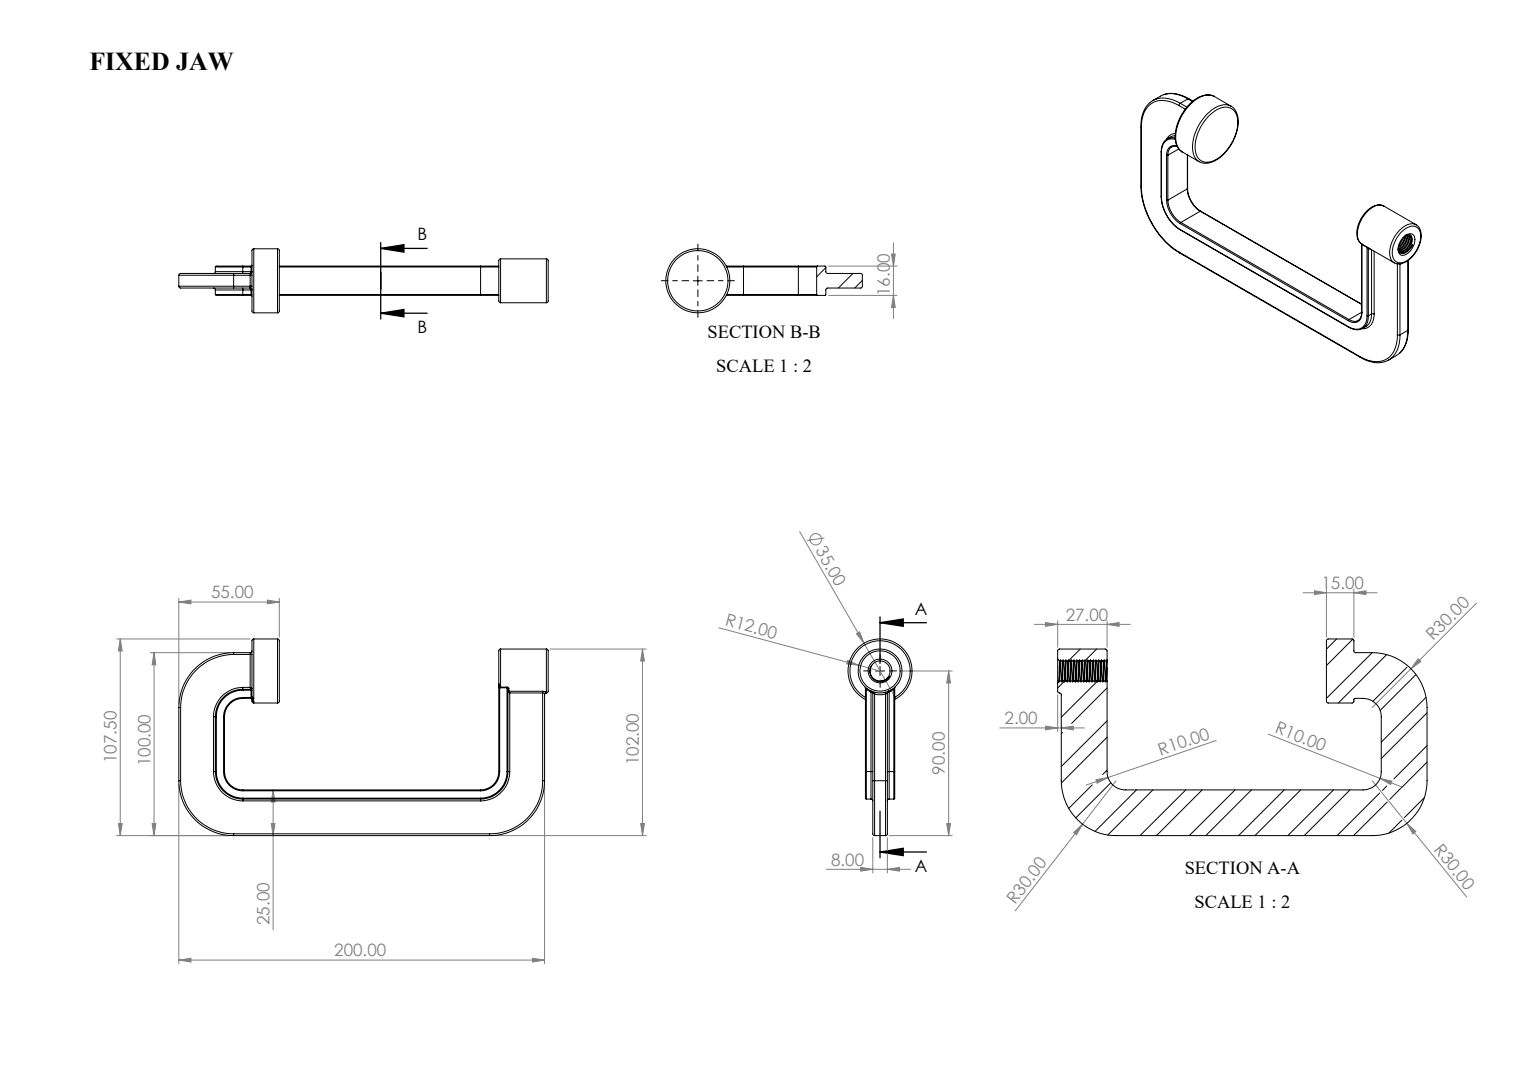
ISO-10303-21;
HEADER;
FILE_DESCRIPTION (('STEP AP214'),
    '1' );
FILE_NAME ('Fixed Jaw.step',
    '2026-10-07T06:38:26',
    ( '' ),
    ( '' ),
    'SwSTEP 2.0',
    'SolidWorks 2021',
    '' );
FILE_SCHEMA (( 'AUTOMOTIVE_DESIGN' ));
ENDSEC;

DATA;
#2=ORIENTED_EDGE ( 'NONE', *, *, #13115, .T. ) ;
#3=CARTESIAN_POINT ( 'NONE',  ( 151.8675748654052029, -5.500000000000012434, 2.278174593052012309 ) ) ;
#4=CARTESIAN_POINT ( 'NONE',  ( 134.2500000000000284, -6.000000000000005329, 0.000000000000000000 ) ) ;
#7=( NAMED_UNIT ( * ) PLANE_ANGLE_UNIT ( ) SI_UNIT ( $, .RADIAN. ) );
#9=ADVANCED_FACE ( 'NONE', ( #19589 ), #12972, .F. ) ;
#11=VECTOR ( 'NONE', #10192, 1000.000000000000000 ) ;
#14=CARTESIAN_POINT ( 'NONE',  ( 116.0000000000000142, 6.735557395310442023E-16, 5.500000000000000000 ) ) ;
#17=CARTESIAN_POINT ( 'NONE',  ( 143.2351497308104058, 3.535533905932725318, -3.535533905932725318 ) ) ;
#19=DIRECTION ( 'NONE',  ( -0.000000000000000000, -0.000000000000000000, -1.000000000000000000 ) ) ;
#25=DIRECTION ( 'NONE',  ( 0.000000000000000000, 0.000000000000000000, -1.000000000000000000 ) ) ;
#28=DIRECTION ( 'NONE',  ( 1.000000000000000000, 0.000000000000000000, 0.000000000000000000 ) ) ;
#31=ORIENTED_EDGE ( 'NONE', *, *, #1535, .F. ) ;
#33=CARTESIAN_POINT ( 'NONE',  ( 142.6875000000000284, 4.242640687119269671, 4.242640687119298093 ) ) ;
#38=CARTESIAN_POINT ( 'NONE',  ( 160.5788997308103774, -4.999999999999989342, 2.071067811865468400 ) ) ;
#42=VERTEX_POINT ( 'NONE', #1381 ) ;
#44=ORIENTED_EDGE ( 'NONE', *, *, #20112, .T. ) ;
#49=CARTESIAN_POINT ( 'NONE',  ( 159.6411875853270885, -12.17723633016814233, -3.777793391642500165 ) ) ;
#53=DIRECTION ( 'NONE',  ( -1.000000000000000000, -0.000000000000000000, -0.000000000000000000 ) ) ;
#54=VECTOR ( 'NONE', #17424, 1000.000000000000000 ) ;
#56=ADVANCED_FACE ( 'NONE', ( #10625 ), #5822, .T. ) ;
#60=CARTESIAN_POINT ( 'NONE',  ( 139.5760635317500089, -9.165151396444613852, -8.000000000000007105 ) ) ;
#64=DIRECTION ( 'NONE',  ( 6.938893903907222067E-15, 1.000000000000000000, 0.000000000000000000 ) ) ;
#69=CARTESIAN_POINT ( 'NONE',  ( 145.1398502691896510, -3.535533905932752852, 3.535533905932725318 ) ) ;
#72=CARTESIAN_POINT ( 'NONE',  ( 157.4062500000000284, 6.000000000000005329, -2.485281374238556218 ) ) ;
#77=DIRECTION ( 'NONE',  ( 1.000000000000000000, 0.000000000000000000, 0.000000000000000000 ) ) ;
#79=CARTESIAN_POINT ( 'NONE',  ( 150.3750000000000284, 0.000000000000000000, 6.000000000000005329 ) ) ;
#83=ORIENTED_EDGE ( 'NONE', *, *, #26629, .F. ) ;
#88=EDGE_CURVE ( 'NONE', #16343, #27983, #2946, .T. ) ;
#93=CARTESIAN_POINT ( 'NONE',  ( 156.4538997308104626, -2.071067811865468400, -4.999999999999989342 ) ) ;
#96=CARTESIAN_POINT ( 'NONE',  ( 135.6737246954180023, -8.728829995094853800, 8.172675940893835644 ) ) ;
#98=ADVANCED_FACE ( 'NONE', ( #17543 ), #26707, .F. ) ;
#101=STYLED_ITEM ( 'NONE', ( #7132 ), #3790 ) ;
#107=CARTESIAN_POINT ( 'NONE',  ( 135.0000000000000284, -54.99999999999993605, -7.500000000000007105 ) ) ;
#108=CARTESIAN_POINT ( 'NONE',  ( 125.0000000000000568, -55.00000000000000711, -7.500000000000007105 ) ) ;
#111=CARTESIAN_POINT ( 'NONE',  ( 161.5461002691896226, -2.071067811865468400, 4.999999999999989342 ) ) ;
#112=CARTESIAN_POINT ( 'NONE',  ( 0.7724517649218355375, -15.49026069396310490, 8.142614232235679594 ) ) ;
#117=CARTESIAN_POINT ( 'NONE',  ( -4.999999999999990230, -55.00000000000002132, 5.000000000000004441 ) ) ;
#121=DIRECTION ( 'NONE',  ( 0.000000000000000000, 0.000000000000000000, -1.000000000000000000 ) ) ;
#125=CARTESIAN_POINT ( 'NONE',  ( 151.9687500000000568, -2.485281374238585972, 6.000000000000005329 ) ) ;
#126=ORIENTED_EDGE ( 'NONE', *, *, #11372, .T. ) ;
#136=CARTESIAN_POINT ( 'NONE',  ( 134.2351497308104058, 3.535533905932725318, -3.535533905932725318 ) ) ;
#138=CARTESIAN_POINT ( 'NONE',  ( 0.1879814459054835185, -15.40071801525260220, -8.313003687118166951 ) ) ;
#139=ADVANCED_FACE ( 'NONE', ( #915 ), #19679, .F. ) ;
#140=COLOUR_RGB ( '', 0.31764706, 0.68627451, 0.89019608) ;
#142=CYLINDRICAL_SURFACE ( 'NONE', #25085, 0.5000000000000004441 ) ;
#146=CARTESIAN_POINT ( 'NONE',  ( -0.5130136762305975706, -9.973972647538804637, -4.738252045315842764 ) ) ;
#147=CARTESIAN_POINT ( 'NONE',  ( 159.9897649647779474, -11.17313463120727057, -4.377898023955410167 ) ) ;
#150=CARTESIAN_POINT ( 'NONE',  ( 135.0000000000000284, -8.662311887307041047, -7.546725650337192448 ) ) ;
#151=CARTESIAN_POINT ( 'NONE',  ( 154.1175748654052313, 5.500000000000012434, -2.278174593052012309 ) ) ;
#158=AXIS2_PLACEMENT_3D ( 'NONE', #25640, #4289, #30093 ) ;
#162=CARTESIAN_POINT ( 'NONE',  ( 142.5863248654052313, 0.000000000000000000, 5.500000000000005329 ) ) ;
#164=ORIENTED_EDGE ( 'NONE', *, *, #27531, .F. ) ;
#167=CARTESIAN_POINT ( 'NONE',  ( 135.1875000000000568, 4.242640687119269671, 4.242640687119298093 ) ) ;
#168=EDGE_CURVE ( 'NONE', #2390, #1119, #5990, .T. ) ;
#169=ADVANCED_FACE ( 'NONE', ( #22749 ), #29791, .T. ) ;
#171=CARTESIAN_POINT ( 'NONE',  ( -4.999999999999920952, -65.50000000000001421, -8.000000000000007105 ) ) ;
#172=( NAMED_UNIT ( * ) PLANE_ANGLE_UNIT ( ) SI_UNIT ( $, .RADIAN. ) );
#175=CIRCLE ( 'NONE', #14898, 0.5000000000000004441 ) ;
#176=CARTESIAN_POINT ( 'NONE',  ( 144.5476497308104058, 0.000000000000000000, -5.000000000000004441 ) ) ;
#180=AXIS2_PLACEMENT_3D ( 'NONE', #24945, #8684, #29090 ) ;
#183=ORIENTED_EDGE ( 'NONE', *, *, #15487, .T. ) ;
#185=DIRECTION ( 'NONE',  ( 0.000000000000000000, 0.000000000000000000, 1.000000000000000000 ) ) ;
#187=ORIENTED_EDGE ( 'NONE', *, *, #6959, .T. ) ;
#189=CARTESIAN_POINT ( 'NONE',  ( 139.2187500000000284, 2.485281374238556218, -6.000000000000005329 ) ) ;
#191=DIRECTION ( 'NONE',  ( -0.000000000000000000, 1.000000000000000000, -0.000000000000000000 ) ) ;
#192=CARTESIAN_POINT ( 'NONE',  ( 132.8437500000000284, -6.000000000000005329, -2.485281374238555774 ) ) ;
#193=COLOUR_RGB ( '', 0.31764706, 0.68627451, 0.89019608) ;
#195=EDGE_CURVE ( 'NONE', #1664, #6421, #4446, .T. ) ;
#200=CARTESIAN_POINT ( 'NONE',  ( -19.99999999999998224, -25.00000000000010658, -5.000000000000004441 ) ) ;
#217=CARTESIAN_POINT ( 'NONE',  ( 145.0461002691896510, -2.071067811865468400, 4.999999999999989342 ) ) ;
#219=CARTESIAN_POINT ( 'NONE',  ( 157.2187500000000284, 2.485281374238556218, -6.000000000000005329 ) ) ;
#227=CARTESIAN_POINT ( 'NONE',  ( 149.4375000000000284, -4.242640687119298093, -4.242640687119298093 ) ) ;
#234=VERTEX_POINT ( 'NONE', #29941 ) ;
#239=CARTESIAN_POINT ( 'NONE',  ( 154.6726497308104058, -5.000000000000004441, 0.000000000000000000 ) ) ;
#242=DIRECTION ( 'NONE',  ( 1.000000000000000000, -0.000000000000000000, -0.000000000000000000 ) ) ;
#245=LINE ( 'NONE', #5439, #2253 ) ;
#246=AXIS2_PLACEMENT_3D ( 'NONE', #9140, #8524, #18081 ) ;
#250=AXIS2_PLACEMENT_3D ( 'NONE', #6454, #4145, #24741 ) ;
#252=DIRECTION ( 'NONE',  ( 1.000000000000000000, 0.000000000000000000, 0.000000000000000000 ) ) ;
#253=CARTESIAN_POINT ( 'NONE',  ( 144.7574251345947687, -2.278174593051733421, 5.500000000000292211 ) ) ;
#257=CARTESIAN_POINT ( 'NONE',  ( 156.7648502691896510, 3.535533905932725318, 3.535533905932752852 ) ) ;
#258=CARTESIAN_POINT ( 'NONE',  ( 124.9999999999999432, -65.00000000000000000, -7.500000000000007105 ) ) ;
#259=ORIENTED_EDGE ( 'NONE', *, *, #5614, .F. ) ;
#273=CARTESIAN_POINT ( 'NONE',  ( 153.4687500000000853, -2.485281374238585972, 6.000000000000005329 ) ) ;
#278=VERTEX_POINT ( 'NONE', #29639 ) ;
#279=CARTESIAN_POINT ( 'NONE',  ( 116.0000000000000142, 0.000000000000000000, 0.000000000000000000 ) ) ;
#289=SURFACE_SIDE_STYLE ('',( #7647 ) ) ;
#294=ORIENTED_EDGE ( 'NONE', *, *, #12008, .F. ) ;
#296=CIRCLE ( 'NONE', #5196, 0.5000000000000004441 ) ;
#299=LINE ( 'NONE', #12465, #20459 ) ;
#302=PLANE ( 'NONE',  #5431 ) ;
#307=CARTESIAN_POINT ( 'NONE',  ( 157.0386751345948539, -5.500000000000005329, 0.000000000000000000 ) ) ;
#308=CARTESIAN_POINT ( 'NONE',  ( 140.9925748654052029, 2.278174593052074925, 5.499999999999950262 ) ) ;
#311=CARTESIAN_POINT ( 'NONE',  ( 138.4687500000000284, -2.485281374238585972, 6.000000000000005329 ) ) ;
#314=( LENGTH_UNIT ( ) NAMED_UNIT ( * ) SI_UNIT ( .MILLI., .METRE. ) );
#318=CARTESIAN_POINT ( 'NONE',  ( 0.1092184406287978471, -15.15152031211519201, 8.760553818335999665 ) ) ;
#319=CARTESIAN_POINT ( 'NONE',  ( 136.1101497308104342, 3.535533905932725318, 3.535533905932725318 ) ) ;
#327=ORIENTED_EDGE ( 'NONE', *, *, #30362, .T. ) ;
#328=ADVANCED_FACE ( 'NONE', ( #15715 ), #11243, .F. ) ;
#329=CARTESIAN_POINT ( 'NONE',  ( -20.99999999999998224, -54.99999999999990763, -4.000000000000003553 ) ) ;
#332=EDGE_CURVE ( 'NONE', #7475, #16343, #25564, .T. ) ;
#333=ORIENTED_EDGE ( 'NONE', *, *, #11296, .T. ) ;
#337=CARTESIAN_POINT ( 'NONE',  ( 133.5000000000000284, 6.000000000000005329, 0.000000000000000000 ) ) ;
#339=COLOUR_RGB ( '', 0.72549020, 0.75294118, 0.79215686) ;
#346=CARTESIAN_POINT ( 'NONE',  ( 159.0000000000000284, -12.00000000000001066, -4.000000000000003553 ) ) ;
#348=AXIS2_PLACEMENT_3D ( 'NONE', #13196, #18093, #13038 ) ;
#350=CARTESIAN_POINT ( 'NONE',  ( 140.9019117484300523, -11.80382349685862486, -4.000000000000003553 ) ) ;
#351=DIRECTION ( 'NONE',  ( 1.000000000000000000, -0.000000000000000000, -0.000000000000000000 ) ) ;
#354=CARTESIAN_POINT ( 'NONE',  ( 140.0509928599997238, -9.340762233865111952, 7.535282035301673176 ) ) ;
#355=AXIS2_PLACEMENT_3D ( 'NONE', #19839, #19142, #17411 ) ;
#358=AXIS2_PLACEMENT_3D ( 'NONE', #28689, #759, #17069 ) ;
#359=CARTESIAN_POINT ( 'NONE',  ( 145.1175748654052597, 5.500000000000012434, -2.278174593052012309 ) ) ;
#362=EDGE_CURVE ( 'NONE', #22602, #4075, #22644, .T. ) ;
#363=CARTESIAN_POINT ( 'NONE',  ( 139.5500633684294769, -9.165151389911672553, 8.000000000000010658 ) ) ;
#364=CARTESIAN_POINT ( 'NONE',  ( 146.8273502691896510, -5.000000000000004441, 0.000000000000000000 ) ) ;
#365=CARTESIAN_POINT ( 'NONE',  ( 13.99999999999999822, 0.000000000000000000, 17.50000000000000355 ) ) ;
#366=CARTESIAN_POINT ( 'NONE',  ( 160.5937500000000284, 6.000000000000005329, 2.485281374238585972 ) ) ;
#367=CARTESIAN_POINT ( 'NONE',  ( 135.0000000000000284, -8.301023251189437957, -7.690744244795082452 ) ) ;
#368=FACE_OUTER_BOUND ( 'NONE', #26036, .T. ) ;
#370=( NAMED_UNIT ( * ) PLANE_ANGLE_UNIT ( ) SI_UNIT ( $, .RADIAN. ) );
#372=CARTESIAN_POINT ( 'NONE',  ( 148.4062500000000568, 6.000000000000005329, -2.485281374238555774 ) ) ;
#374=( NAMED_UNIT ( * ) PLANE_ANGLE_UNIT ( ) SI_UNIT ( $, .RADIAN. ) );
#379=VERTEX_POINT ( 'NONE', #23659 ) ;
#383=CARTESIAN_POINT ( 'NONE',  ( 155.5163997308104342, 4.999999999999989342, 2.071067811865468400 ) ) ;
#387=SURFACE_SIDE_STYLE ('',( #14990 ) ) ;
#397=PLANE ( 'NONE',  #15284 ) ;
#400=CARTESIAN_POINT ( 'NONE',  ( 155.3586002691896226, 2.071067811865468400, 4.999999999999989342 ) ) ;
#404=CARTESIAN_POINT ( 'NONE',  ( 149.3363248654052029, 0.000000000000000000, -5.500000000000005329 ) ) ;
#410=ORIENTED_EDGE ( 'NONE', *, *, #8956, .T. ) ;
#412=ORIENTED_EDGE ( 'NONE', *, *, #17980, .F. ) ;
#413=CARTESIAN_POINT ( 'NONE',  ( 146.7187500000000284, 2.485281374238555774, -6.000000000000005329 ) ) ;
#414=ORIENTED_EDGE ( 'NONE', *, *, #12706, .T. ) ;
#418=UNCERTAINTY_MEASURE_WITH_UNIT (LENGTH_MEASURE( 1.000000000000000082E-05 ), #11834, 'distance_accuracy_value', 'NONE');
#423=CARTESIAN_POINT ( 'NONE',  ( 133.4851497308104058, -3.535533905932725318, 3.535533905932725318 ) ) ;
#426=CARTESIAN_POINT ( 'NONE',  ( 0.2111655239558809238, -15.49101385207805492, -8.141616853885579985 ) ) ;
#427=CARTESIAN_POINT ( 'NONE',  ( 158.5386751345948539, -5.500000000000005329, 0.000000000000000000 ) ) ;
#428=CYLINDRICAL_SURFACE ( 'NONE', #8935, 30.00000000000000000 ) ;
#436=EDGE_CURVE ( 'NONE', #17742, #25655, #11378, .T. ) ;
#438=CARTESIAN_POINT ( 'NONE',  ( 135.4999999999990052, -9.047800747817513312, -8.000000000000007105 ) ) ;
#441=DIRECTION ( 'NONE',  ( 0.000000000000000000, 0.000000000000000000, -1.000000000000000000 ) ) ;
#446=AXIS2_PLACEMENT_3D ( 'NONE', #10967, #13586, #23085 ) ;
#450=( BOUNDED_CURVE ( )  B_SPLINE_CURVE ( 2, ( #19930, #8557, #7941, #22090, #29276, #19775, #5935, #15359, #8402 ),
 .UNSPECIFIED., .F., .F. ) 
 B_SPLINE_CURVE_WITH_KNOTS ( ( 3, 2, 2, 2, 3 ),
 ( 0.1874999999999996947, 0.1937499999999999500, 0.2000000000000002054, 0.2062500000000004330, 0.2125000000000006883 ),
 .UNSPECIFIED. ) 
 CURVE ( )  GEOMETRIC_REPRESENTATION_ITEM ( )  RATIONAL_B_SPLINE_CURVE ( ( 1.000000000000003775, 0.9238795325112830747, 1.000000000000000000, 0.9238795325112867385, 1.000000000000000000, 0.9238795325112867385, 1.000000000000000000, 0.9238795325112783008, 1.000000000000008438 ) ) 
 REPRESENTATION_ITEM ( '' )  );
#452=VERTEX_POINT ( 'NONE', #16766 ) ;
#454=CARTESIAN_POINT ( 'NONE',  ( 134.4523502691896510, 0.000000000000000000, 5.000000000000004441 ) ) ;
#459=CARTESIAN_POINT ( 'NONE',  ( 116.0000000000000142, 0.000000000000000000, -5.500000000000000000 ) ) ;
#461=ORIENTED_EDGE ( 'NONE', *, *, #4777, .F. ) ;
#463=CARTESIAN_POINT ( 'NONE',  ( 0.1053031288717025393, -15.23283975038566318, 8.619984219653339608 ) ) ;
#464=CARTESIAN_POINT ( 'NONE',  ( 139.8601497308104058, -3.535533905932725318, -3.535533905932725318 ) ) ;
#466=DIRECTION ( 'NONE',  ( 1.000000000000000000, 0.000000000000000000, 0.000000000000000000 ) ) ;
#468=( NAMED_UNIT ( * ) PLANE_ANGLE_UNIT ( ) SI_UNIT ( $, .RADIAN. ) );
#476=VERTEX_POINT ( 'NONE', #745 ) ;
#477=DIRECTION ( 'NONE',  ( 0.000000000000000000, 1.224646799147353454E-16, 1.000000000000000000 ) ) ;
#479=ORIENTED_EDGE ( 'NONE', *, *, #25996, .F. ) ;
#481=CARTESIAN_POINT ( 'NONE',  ( 136.2187500000000284, 2.485281374238556218, -6.000000000000005329 ) ) ;
#485=CARTESIAN_POINT ( 'NONE',  ( 160.9538997308104058, -2.071067811865468400, -4.999999999999989342 ) ) ;
#487=CIRCLE ( 'NONE', #25995, 17.50000000000000355 ) ;
#489=AXIS2_PLACEMENT_3D ( 'NONE', #15313, #15469, #1284 ) ;
#493=EDGE_CURVE ( 'NONE', #3216, #20658, #28980, .T. ) ;
#502=CARTESIAN_POINT ( 'NONE',  ( 116.0000000000000142, 0.000000000000000000, -5.500000000000000000 ) ) ;
#507=CARTESIAN_POINT ( 'NONE',  ( 139.6011751345948539, 3.889087296526011706, -3.889087296526011706 ) ) ;
#508=AXIS2_PLACEMENT_3D ( 'NONE', #25825, #23387, #22922 ) ;
#513=CARTESIAN_POINT ( 'NONE',  ( 146.5461002691896510, -2.071067811865468400, 4.999999999999989342 ) ) ;
#515=CARTESIAN_POINT ( 'NONE',  ( 153.9375000000000284, -4.242640687119298093, -4.242640687119298093 ) ) ;
#519=AXIS2_PLACEMENT_3D ( 'NONE', #17217, #21810, #19211 ) ;
#520=ORIENTED_EDGE ( 'NONE', *, *, #8340, .T. ) ;
#521=CARTESIAN_POINT ( 'NONE',  ( 149.6250000000000284, 0.000000000000000000, -6.000000000000005329 ) ) ;
#523=UNCERTAINTY_MEASURE_WITH_UNIT (LENGTH_MEASURE( 1.000000000000000082E-05 ), #26176, 'distance_accuracy_value', 'NONE');
#527=ORIENTED_EDGE ( 'NONE', *, *, #25589, .T. ) ;
#535=ORIENTED_EDGE ( 'NONE', *, *, #24962, .F. ) ;
#540=CARTESIAN_POINT ( 'NONE',  ( 134.9486760520005078, -8.594915014419392207, 8.000000000000007105 ) ) ;
#543=CARTESIAN_POINT ( 'NONE',  ( 143.3363248654052029, 0.000000000000000000, -5.500000000000005329 ) ) ;
#547=( BOUNDED_SURFACE ( )  B_SPLINE_SURFACE ( 3, 2, ( 
 ( #13704, #1829, #23045 ),
 ( #11233, #20739, #27768 ),
 ( #8443, #14456, #16759 ),
 ( #2587, #11702, #20890 ),
 ( #2301, #21499, #23504 ),
 ( #4588, #426, #4740 ),
 ( #16902, #19192, #4435 ),
 ( #7051, #14167, #11858 ),
 ( #21198, #138, #737 ),
 ( #26662, #8079, #7637 ),
 ( #12747, #12446, #19491 ),
 ( #10269, #10420, #14736 ),
 ( #17198, #19634, #26225 ),
 ( #24223, #10119, #7781 ) ),
 .UNSPECIFIED., .F., .F., .F. ) 
 B_SPLINE_SURFACE_WITH_KNOTS ( ( 4, 2, 2, 2, 2, 2, 4 ),
 ( 3, 3 ),
 ( 0.007087992156775593799, 0.007143427954787825995, 0.007198863752800057324, 0.007254299550812288652, 0.007309735348824520848, 0.007420606944848983505, 0.007531478540873447029 ),
 ( 0.000000000000000000, 1.000000000000000000 ),
 .UNSPECIFIED. ) 
 GEOMETRIC_REPRESENTATION_ITEM ( )  RATIONAL_B_SPLINE_SURFACE ( (
 ( 1.000000000000000000, 0.8593225670956824436, 1.000000000000000000),
 ( 1.000000000000000000, 0.8663660590095438874, 1.000000000000000000),
 ( 1.000000000000000000, 0.8726340236266260098, 1.000000000000000000),
 ( 1.000000000000000000, 0.8802009473587890653, 1.000000000000000000),
 ( 1.000000000000000000, 0.8813323811479394365, 1.000000000000000000),
 ( 1.000000000000000000, 0.8771298408144754255, 1.000000000000000000),
 ( 1.000000000000000000, 0.8720285761146205905, 1.000000000000000000),
 ( 1.000000000000000000, 0.8593306477498514617, 1.000000000000000000),
 ( 1.000000000000000000, 0.8518162931196250343, 1.000000000000000000),
 ( 1.000000000000000000, 0.8295128813679467639, 1.000000000000000000),
 ( 1.000000000000000000, 0.8153081809651850920, 1.000000000000000000),
 ( 1.000000000000000000, 0.7919334258735726273, 1.000000000000000000),
 ( 1.000000000000000000, 0.7823637235328708694, 1.000000000000000000),
 ( 1.000000000000000000, 0.7743236465966842896, 1.000000000000000000) ) ) 
 REPRESENTATION_ITEM ( '' )  SURFACE ( )  );
#550=CARTESIAN_POINT ( 'NONE',  ( 145.4136751345948539, 0.000000000000000000, -5.500000000000005329 ) ) ;
#552=CARTESIAN_POINT ( 'NONE',  ( 135.5550748654052313, -5.500000000000012434, -2.278174593052012309 ) ) ;
#556=DIRECTION ( 'NONE',  ( 0.000000000000000000, 0.000000000000000000, -1.000000000000000000 ) ) ;
#557=AXIS2_PLACEMENT_3D ( 'NONE', #30242, #4590, #11704 ) ;
#558=( NAMED_UNIT ( * ) PLANE_ANGLE_UNIT ( ) SI_UNIT ( $, .RADIAN. ) );
#560=ORIENTED_EDGE ( 'NONE', *, *, #8732, .F. ) ;
#573=CARTESIAN_POINT ( 'NONE',  ( 158.3363248654052313, 0.000000000000000000, -5.500000000000005329 ) ) ;
#577=CARTESIAN_POINT ( 'NONE',  ( 132.7351497308104058, 3.535533905932725318, -3.535533905932725318 ) ) ;
#582=CARTESIAN_POINT ( 'NONE',  ( 158.7261751345948539, -3.889087296526011706, -3.889087296526011706 ) ) ;
#587=DIRECTION ( 'NONE',  ( 0.000000000000000000, 1.000000000000000000, -1.224646799147353207E-16 ) ) ;
#588=DIRECTION ( 'NONE',  ( 1.000000000000000000, 0.000000000000000000, 0.000000000000000000 ) ) ;
#591=( BOUNDED_CURVE ( )  B_SPLINE_CURVE ( 3, ( #1681, #22434, #25161, #22888 ),
 .UNSPECIFIED., .F., .T. ) 
 B_SPLINE_CURVE_WITH_KNOTS ( ( 4, 4 ),
 ( 1.570796326794896558, 2.746801533890014468 ),
 .UNSPECIFIED. ) 
 CURVE ( )  GEOMETRIC_REPRESENTATION_ITEM ( )  RATIONAL_B_SPLINE_CURVE ( ( 1.000000000000000000, 0.8880335295585656263, 0.8880335295585656263, 1.000000000000000000 ) ) 
 REPRESENTATION_ITEM ( '' )  );
#593=DIRECTION ( 'NONE',  ( -1.000000000000000000, 6.938893903907221278E-15, 0.000000000000000000 ) ) ;
#598=PLANE ( 'NONE',  #4757 ) ;
#600=ORIENTED_EDGE ( 'NONE', *, *, #19995, .T. ) ;
#601=EDGE_CURVE ( 'NONE', #5531, #29422, #23638, .T. ) ;
#605=VERTEX_POINT ( 'NONE', #14955 ) ;
#608=FACE_OUTER_BOUND ( 'NONE', #22324, .T. ) ;
#609=CARTESIAN_POINT ( 'NONE',  ( 161.5312500000000568, -2.485281374238555774, -6.000000000000005329 ) ) ;
#610=EDGE_CURVE ( 'NONE', #5920, #21964, #16795, .T. ) ;
#612=EDGE_LOOP ( 'NONE', ( #28143, #13844, #4187, #4536 ) ) ;
#613=CARTESIAN_POINT ( 'NONE',  ( 135.0000000000000284, 6.735557395310442023E-16, 5.500000000000000000 ) ) ;
#615=CARTESIAN_POINT ( 'NONE',  ( 116.0000000000000142, 0.000000000000000000, 0.000000000000000000 ) ) ;
#617=LINE ( 'NONE', #459, #26505 ) ;
#618=B_SPLINE_CURVE_WITH_KNOTS ( 'NONE', 3,
 ( #5629, #26527, #9972, #878 ),
 .UNSPECIFIED., .F., .F.,
 ( 4, 4 ),
 ( 0.000000000000000000, 0.0004191943366147233034 ),
 .UNSPECIFIED. ) ;
#619=ORIENTED_EDGE ( 'NONE', *, *, #4595, .F. ) ;
#622=DIRECTION ( 'NONE',  ( 0.000000000000000000, 0.000000000000000000, 1.000000000000000000 ) ) ;
#624=CARTESIAN_POINT ( 'NONE',  ( 139.2038997308104058, 2.071067811865468400, 4.999999999999989342 ) ) ;
#627=DIRECTION ( 'NONE',  ( 1.000000000000000000, 0.000000000000000000, 0.000000000000000000 ) ) ;
#631=( NAMED_UNIT ( * ) SI_UNIT ( $, .STERADIAN. ) SOLID_ANGLE_UNIT ( ) );
#632=CARTESIAN_POINT ( 'NONE',  ( 153.7574251345948539, -2.278174593051795149, 5.500000000000228262 ) ) ;
#652=ORIENTED_EDGE ( 'NONE', *, *, #19956, .F. ) ;
#653=MECHANICAL_DESIGN_GEOMETRIC_PRESENTATION_REPRESENTATION('',(#6546),#18839);
#657=DIRECTION ( 'NONE',  ( 1.000000000000000000, 0.000000000000000000, 0.000000000000000000 ) ) ;
#660=CARTESIAN_POINT ( 'NONE',  ( 152.7261751345948539, -3.889087296526011706, -3.889087296526011706 ) ) ;
#662=CARTESIAN_POINT ( 'NONE',  ( 140.3637585460053288, -11.68187927300243345, -4.222310544175148728 ) ) ;
#665=CARTESIAN_POINT ( 'NONE',  ( 139.9918614756773536, -8.909704403337718404, 8.038575526839014884 ) ) ;
#672=CARTESIAN_POINT ( 'NONE',  ( 144.2961002691896795, 2.071067811865468400, -4.999999999999989342 ) ) ;
#673=CARTESIAN_POINT ( 'NONE',  ( 150.0000000000000284, 6.000000000000005329, 0.000000000000000000 ) ) ;
#676=EDGE_CURVE ( 'NONE', #12037, #42, #5973, .T. ) ;
#678=( LENGTH_UNIT ( ) NAMED_UNIT ( * ) SI_UNIT ( .MILLI., .METRE. ) );
#680=CARTESIAN_POINT ( 'NONE',  ( 142.3125000000000284, 4.242640687119298093, -4.242640687119298093 ) ) ;
#682=B_SPLINE_CURVE_WITH_KNOTS ( 'NONE', 3,
 ( #9797, #28649, #26068, #3010, #25919, #2864, #19176, #7620 ),
 .UNSPECIFIED., .F., .F.,
 ( 4, 2, 2, 4 ),
 ( 0.000000000000000000, 0.0002903981794584280240, 0.0005807963589168560481, 0.001161592717833712096 ),
 .UNSPECIFIED. ) ;
#683=EDGE_CURVE ( 'NONE', #22336, #13151, #10426, .T. ) ;
#691=VERTEX_POINT ( 'NONE', #5851 ) ;
#692=DIRECTION ( 'NONE',  ( -0.000000000000000000, 0.000000000000000000, 1.000000000000000000 ) ) ;
#695=DIRECTION ( 'NONE',  ( 0.000000000000000000, 0.000000000000000000, -1.000000000000000000 ) ) ;
#703=DIRECTION ( 'NONE',  ( 0.000000000000000000, 0.000000000000000000, 1.000000000000000000 ) ) ;
#707=CARTESIAN_POINT ( 'NONE',  ( 140.0000000000000284, 0.000000000000000000, 0.000000000000000000 ) ) ;
#708=CARTESIAN_POINT ( 'NONE',  ( 157.4211002691896510, -4.999999999999989342, -2.071067811865468400 ) ) ;
#714=FILL_AREA_STYLE_COLOUR ( '', #23926 ) ;
#717=EDGE_LOOP ( 'NONE', ( #27605, #12662, #17142, #22496 ) ) ;
#722=CARTESIAN_POINT ( 'NONE',  ( 145.5000000000000284, 6.000000000000005329, 0.000000000000000000 ) ) ;
#731=CARTESIAN_POINT ( 'NONE',  ( -0.4142135623730960892, -9.292893218813460976, 4.000000000000004441 ) ) ;
#732=TOROIDAL_SURFACE ( 'NONE', #28662, 1.000000000000000000, 0.5000000000000000000 ) ;
#737=CARTESIAN_POINT ( 'NONE',  ( 0.7723847956792433411, -15.49036276797524891, -8.142419924191026226 ) ) ;
#738=CARTESIAN_POINT ( 'NONE',  ( 158.2574251345948539, -2.278174593051826236, 5.500000000000198064 ) ) ;
#739=CARTESIAN_POINT ( 'NONE',  ( 116.0000000000000142, 0.000000000000000000, 0.000000000000000000 ) ) ;
#745=CARTESIAN_POINT ( 'NONE',  ( -19.99999999999998224, -25.00000000000010658, 5.000000000000004441 ) ) ;
#746=AXIS2_PLACEMENT_3D ( 'NONE', #18168, #3378, #12804 ) ;
#755=EDGE_LOOP ( 'NONE', ( #871, #25414, #7664, #11467 ) ) ;
#756=FILL_AREA_STYLE ('',( #7658 ) ) ;
#759=DIRECTION ( 'NONE',  ( 1.000000000000000000, 0.000000000000000000, -0.000000000000000000 ) ) ;
#762=ORIENTED_EDGE ( 'NONE', *, *, #5312, .T. ) ;
#763=ORIENTED_EDGE ( 'NONE', *, *, #21634, .T. ) ;
#764=CARTESIAN_POINT ( 'NONE',  ( 135.3898502691896510, 3.535533905932725318, -3.535533905932725318 ) ) ;
#765=VERTEX_POINT ( 'NONE', #10655 ) ;
#769=( LENGTH_UNIT ( ) NAMED_UNIT ( * ) SI_UNIT ( .MILLI., .METRE. ) );
#772=ORIENTED_EDGE ( 'NONE', *, *, #22651, .T. ) ;
#775=CARTESIAN_POINT ( 'NONE',  ( 135.5000000000000284, -9.047800747817580813, -8.000000000000007105 ) ) ;
#777=CARTESIAN_POINT ( 'NONE',  ( 139.7663997308104342, -4.999999999999989342, -2.071067811865468400 ) ) ;
#779=DIRECTION ( 'NONE',  ( 1.000000000000000000, -0.000000000000000000, 0.000000000000000000 ) ) ;
#780=ADVANCED_FACE ( 'NONE', ( #10194 ), #11219, .F. ) ;
#782=CARTESIAN_POINT ( 'NONE',  ( -0.5000000000000004441, -15.50000000000001421, 7.500000000000007105 ) ) ;
#786=CARTESIAN_POINT ( 'NONE',  ( 0.8631338372297875372, -15.37878787878788067, -8.351220472436777342 ) ) ;
#789=DIRECTION ( 'NONE',  ( 1.000000000000000000, 0.000000000000000000, 0.000000000000000000 ) ) ;
#790=ADVANCED_FACE ( 'NONE', ( #29667 ), #8635, .T. ) ;
#791=ORIENTED_EDGE ( 'NONE', *, *, #29842, .T. ) ;
#795=CARTESIAN_POINT ( 'NONE',  ( 13.99999999999999822, 0.000000000000000000, 0.000000000000000000 ) ) ;
#797=CARTESIAN_POINT ( 'NONE',  ( 140.4831164018241338, -11.48311640182299698, 4.126236462591083232 ) ) ;
#800=EDGE_LOOP ( 'NONE', ( #8417, #10263, #10021, #8901 ) ) ;
#802=CARTESIAN_POINT ( 'NONE',  ( 159.0000000000000284, -11.07692307692306777, 4.615384615384604317 ) ) ;
#807=DIRECTION ( 'NONE',  ( -1.000000000000000000, 0.000000000000000000, 0.000000000000000000 ) ) ;
#811=CARTESIAN_POINT ( 'NONE',  ( 140.5000000000000000, -9.600000000000008527, 7.199999999999995737 ) ) ;
#816=ORIENTED_EDGE ( 'NONE', *, *, #14649, .T. ) ;
#817=CARTESIAN_POINT ( 'NONE',  ( 142.0461002691896795, -2.071067811865468400, 4.999999999999989342 ) ) ;
#818=CARTESIAN_POINT ( 'NONE',  ( 152.3437500000000853, -6.000000000000005329, -2.485281374238556218 ) ) ;
#822=CIRCLE ( 'NONE', #18037, 10.49999999999999822 ) ;
#824=CARTESIAN_POINT ( 'NONE',  ( 141.8437500000000284, -6.000000000000005329, -2.485281374238555774 ) ) ;
#825=LINE ( 'NONE', #21591, #17050 ) ;
#826=COLOUR_RGB ( '', 0.31764706, 0.68627451, 0.89019608) ;
#827=CARTESIAN_POINT ( 'NONE',  ( -4.999999999999990230, -9.165151389911669000, -8.000000000000007105 ) ) ;
#831=FILL_AREA_STYLE_COLOUR ( '', #193 ) ;
#834=CARTESIAN_POINT ( 'NONE',  ( 0.000000000000000000, 11.00000000000001066, 4.000000000000003553 ) ) ;
#836=DIRECTION ( 'NONE',  ( 0.000000000000000000, 0.000000000000000000, 1.000000000000000000 ) ) ;
#838=CARTESIAN_POINT ( 'NONE',  ( -20.99999999999998224, -54.99999999999990763, -5.000000000000004441 ) ) ;
#842=CARTESIAN_POINT ( 'NONE',  ( 135.0000000000000284, 6.000000000000005329, 0.000000000000000000 ) ) ;
#845=EDGE_CURVE ( 'NONE', #8188, #25843, #3483, .T. ) ;
#850=DIRECTION ( 'NONE',  ( 0.000000000000000000, 0.000000000000000000, -1.000000000000000000 ) ) ;
#852=( BOUNDED_CURVE ( )  B_SPLINE_CURVE ( 2, ( #24151, #4805, #2504, #29351, #26590, #5848, #8314, #29192, #17722 ),
 .UNSPECIFIED., .F., .T. ) 
 B_SPLINE_CURVE_WITH_KNOTS ( ( 3, 2, 2, 2, 3 ),
 ( 0.2624999999999988454, 0.2687499999999991562, 0.2749999999999993561, 0.2812499999999996114, 0.2874999999999998113 ),
 .UNSPECIFIED. ) 
 CURVE ( )  GEOMETRIC_REPRESENTATION_ITEM ( )  RATIONAL_B_SPLINE_CURVE ( ( 1.000000000000013545, 0.9238795325112731938, 1.000000000000000000, 0.9238795325112867385, 1.000000000000000000, 0.9238795325112867385, 1.000000000000000000, 0.9238795325112887369, 0.9999999999999980016 ) ) 
 REPRESENTATION_ITEM ( '' )  );
#857=MECHANICAL_DESIGN_GEOMETRIC_PRESENTATION_REPRESENTATION('',(#20483),#28806);
#858=CARTESIAN_POINT ( 'NONE',  ( 147.3750000000000284, 0.000000000000000000, 6.000000000000005329 ) ) ;
#867=CARTESIAN_POINT ( 'NONE',  ( 147.0074251345948539, 2.278174593052012309, -5.500000000000012434 ) ) ;
#868=( GEOMETRIC_REPRESENTATION_CONTEXT ( 3 ) GLOBAL_UNCERTAINTY_ASSIGNED_CONTEXT ( ( #5005 ) ) GLOBAL_UNIT_ASSIGNED_CONTEXT ( ( #1107, #10205, #8488 ) ) REPRESENTATION_CONTEXT ( 'NONE', 'WORKASPACE' ) );
#871=ORIENTED_EDGE ( 'NONE', *, *, #20566, .F. ) ;
#872=DIRECTION ( 'NONE',  ( 1.000000000000000000, 1.067522139062651411E-16, -0.000000000000000000 ) ) ;
#874=DIRECTION ( 'NONE',  ( 1.000000000000000000, 1.067522139062651904E-16, -0.000000000000000000 ) ) ;
#878=CARTESIAN_POINT ( 'NONE',  ( 0.000000000000000000, -14.14213562373095634, 8.500000000000007105 ) ) ;
#880=CARTESIAN_POINT ( 'NONE',  ( 160.0000000000000284, -59.99999999999980105, 4.000000000000003553 ) ) ;
#894=FILL_AREA_STYLE ('',( #9836 ) ) ;
#896=DIRECTION ( 'NONE',  ( -1.000000000000000000, 6.938893903907222067E-15, 0.000000000000000000 ) ) ;
#897=ORIENTED_EDGE ( 'NONE', *, *, #14049, .F. ) ;
#898=CARTESIAN_POINT ( 'NONE',  ( 134.5461002691896510, -2.071067811865468400, 4.999999999999989342 ) ) ;
#902=CARTESIAN_POINT ( 'NONE',  ( 161.0000000000000284, 0.000000000000000000, 0.000000000000000000 ) ) ;
#903=CARTESIAN_POINT ( 'NONE',  ( 143.9136751345948539, 0.000000000000000000, -5.500000000000005329 ) ) ;
#905=DIRECTION ( 'NONE',  ( -1.000000000000000000, -6.938893903907222067E-15, 0.000000000000000000 ) ) ;
#906=CARTESIAN_POINT ( 'NONE',  ( -4.999999999999990230, -55.00000000000002132, 8.000000000000007105 ) ) ;
#909=CARTESIAN_POINT ( 'NONE',  ( 137.9851497308104058, -3.535533905932725318, 3.535533905932725318 ) ) ;
#910=CARTESIAN_POINT ( 'NONE',  ( 137.8050748654052597, 5.500000000000012434, 2.278174593052012309 ) ) ;
#913=( LENGTH_UNIT ( ) NAMED_UNIT ( * ) SI_UNIT ( .MILLI., .METRE. ) );
#915=FACE_OUTER_BOUND ( 'NONE', #16215, .T. ) ;
#917=DIRECTION ( 'NONE',  ( 1.000000000000000000, -0.000000000000000000, -0.000000000000000000 ) ) ;
#924=STYLED_ITEM ( 'NONE', ( #25837 ), #14331 ) ;
#927=CARTESIAN_POINT ( 'NONE',  ( 136.5000000000000284, 6.000000000000005329, 0.000000000000000000 ) ) ;
#929=FACE_OUTER_BOUND ( 'NONE', #23458, .T. ) ;
#932=CARTESIAN_POINT ( 'NONE',  ( 140.6451377260904678, -11.29027545218218087, 4.288736938852112601 ) ) ;
#940=FACE_OUTER_BOUND ( 'NONE', #9045, .T. ) ;
#943=ADVANCED_FACE ( 'NONE', ( #22128 ), #15230, .F. ) ;
#945=CARTESIAN_POINT ( 'NONE',  ( 157.2976497308104342, 0.000000000000000000, 5.000000000000004441 ) ) ;
#949=CARTESIAN_POINT ( 'NONE',  ( 135.5000000000000000, -54.99999999999993605, 8.000000000000007105 ) ) ;
#950=CARTESIAN_POINT ( 'NONE',  ( 139.8824251345948539, 5.500000000000012434, 2.278174593052012309 ) ) ;
#953=FACE_OUTER_BOUND ( 'NONE', #5363, .T. ) ;
#955=CARTESIAN_POINT ( 'NONE',  ( 136.0000000000000284, 0.000000000000000000, 0.000000000000000000 ) ) ;
#957=CARTESIAN_POINT ( 'NONE',  ( 138.8586002691896226, 2.071067811865468400, 4.999999999999989342 ) ) ;
#958=CARTESIAN_POINT ( 'NONE',  ( 151.1250000000000284, 0.000000000000000000, -6.000000000000005329 ) ) ;
#960=AXIS2_PLACEMENT_3D ( 'NONE', #4048, #22201, #11151 ) ;
#965=CARTESIAN_POINT ( 'NONE',  ( 146.0625000000000284, -4.242640687119298093, 4.242640687119298093 ) ) ;
#966=CARTESIAN_POINT ( 'NONE',  ( -4.999999999999920952, -65.00000000000001421, 7.500000000000007105 ) ) ;
#973=SURFACE_SIDE_STYLE ('',( #7890 ) ) ;
#977=EDGE_CURVE ( 'NONE', #23810, #29031, #4696, .T. ) ;
#978=ORIENTED_EDGE ( 'NONE', *, *, #13835, .F. ) ;
#979=ADVANCED_FACE ( 'NONE', ( #10082 ), #9930, .F. ) ;
#983=CARTESIAN_POINT ( 'NONE',  ( 135.0000000000000284, -7.170817622374790368, -8.464363312639777703 ) ) ;
#986=CARTESIAN_POINT ( 'NONE',  ( 137.3363248654052029, 0.000000000000000000, -5.500000000000005329 ) ) ;
#991=DIRECTION ( 'NONE',  ( 1.000000000000000000, -0.000000000000000000, -0.000000000000000000 ) ) ;
#1000=CARTESIAN_POINT ( 'NONE',  ( 160.1250000000000568, 0.000000000000000000, -6.000000000000005329 ) ) ;
#1001=DIRECTION ( 'NONE',  ( 1.000000000000000000, 0.000000000000000000, 0.000000000000000000 ) ) ;
#1005=VECTOR ( 'NONE', #25347, 1000.000000000000000 ) ;
#1006=ORIENTED_EDGE ( 'NONE', *, *, #436, .T. ) ;
#1007=AXIS2_PLACEMENT_3D ( 'NONE', #11830, #2700, #14140 ) ;
#1008=CARTESIAN_POINT ( 'NONE',  ( 147.2812500000000284, 2.485281374238585972, 6.000000000000005329 ) ) ;
#1009=ORIENTED_EDGE ( 'NONE', *, *, #24041, .F. ) ;
#1013=EDGE_CURVE ( 'NONE', #6421, #8510, #3135, .T. ) ;
#1014=ORIENTED_EDGE ( 'NONE', *, *, #14291, .F. ) ;
#1020=EDGE_LOOP ( 'NONE', ( #18550, #4036, #18447, #25532 ) ) ;
#1025=CARTESIAN_POINT ( 'NONE',  ( 0.9172842643931518047, -15.89806073124487185, -7.323133569090728656 ) ) ;
#1031=CARTESIAN_POINT ( 'NONE',  ( 116.0000000000000142, 6.735557395310442023E-16, 5.500000000000000000 ) ) ;
#1033=CARTESIAN_POINT ( 'NONE',  ( 135.5571281299438056, -8.633349045433602598, 8.190208147179278697 ) ) ;
#1036=SURFACE_STYLE_FILL_AREA ( #5338 ) ;
#1040=AXIS2_PLACEMENT_3D ( 'NONE', #7864, #2954, #12983 ) ;
#1044=CARTESIAN_POINT ( 'NONE',  ( 135.3284178065447634, -8.627956986131243511, -8.066146656158570849 ) ) ;
#1045=ORIENTED_EDGE ( 'NONE', *, *, #27533, .F. ) ;
#1049=AXIS2_PLACEMENT_3D ( 'NONE', #25942, #13872, #14024 ) ;
#1051=EDGE_CURVE ( 'NONE', #4225, #9180, #11354, .T. ) ;
#1053=VERTEX_POINT ( 'NONE', #1286 ) ;
#1054=AXIS2_PLACEMENT_3D ( 'NONE', #3334, #26390, #14748 ) ;
#1055=ORIENTED_EDGE ( 'NONE', *, *, #17559, .T. ) ;
#1056=EDGE_LOOP ( 'NONE', ( #1553, #10806, #23532, #17880 ) ) ;
#1057=CARTESIAN_POINT ( 'NONE',  ( 133.0461002691896510, -2.071067811865468400, 4.999999999999989342 ) ) ;
#1059=EDGE_CURVE ( 'NONE', #22372, #26763, #10533, .T. ) ;
#1062=CARTESIAN_POINT ( 'NONE',  ( 157.5863248654052597, 0.000000000000000000, 5.500000000000005329 ) ) ;
#1066=CARTESIAN_POINT ( 'NONE',  ( 140.5384615384615756, -11.07692307692306777, -4.615384615384604317 ) ) ;
#1068=CARTESIAN_POINT ( 'NONE',  ( -0.02759001725020546192, -15.32981123538816703, -6.905035842853324723 ) ) ;
#1069=CARTESIAN_POINT ( 'NONE',  ( 149.1636751345948255, 0.000000000000000000, 5.500000000000005329 ) ) ;
#1070=SURFACE_STYLE_FILL_AREA ( #19813 ) ;
#1076=CARTESIAN_POINT ( 'NONE',  ( 135.0000000000000000, 2.502093630246796874, 4.956520372253784501 ) ) ;
#1080=DIRECTION ( 'NONE',  ( 0.000000000000000000, 1.776356839400250465E-15, -1.000000000000000000 ) ) ;
#1082=CARTESIAN_POINT ( 'NONE',  ( 141.8363248654052029, 0.000000000000000000, -5.500000000000005329 ) ) ;
#1090=EDGE_CURVE ( 'NONE', #15347, #24916, #19018, .T. ) ;
#1092=EDGE_CURVE ( 'NONE', #11180, #15059, #22063, .T. ) ;
#1097=CARTESIAN_POINT ( 'NONE',  ( 136.4925748654052882, 2.278174593052074925, 5.499999999999950262 ) ) ;
#1101=CARTESIAN_POINT ( 'NONE',  ( 148.3913997308104058, -2.071067811865468400, 4.999999999999989342 ) ) ;
#1103=CARTESIAN_POINT ( 'NONE',  ( 135.2243793856090690, -8.380352225012890344, 8.129889850246460270 ) ) ;
#1107=( LENGTH_UNIT ( ) NAMED_UNIT ( * ) SI_UNIT ( .MILLI., .METRE. ) );
#1111=CARTESIAN_POINT ( 'NONE',  ( 151.0312500000000568, -2.485281374238556218, -6.000000000000005329 ) ) ;
#1112=CARTESIAN_POINT ( 'NONE',  ( 159.0000000000000284, -11.07692307692306777, 4.615384615384604317 ) ) ;
#1118=VECTOR ( 'NONE', #779, 1000.000000000000000 ) ;
#1119=VERTEX_POINT ( 'NONE', #8675 ) ;
#1120=CARTESIAN_POINT ( 'NONE',  ( 144.6562500000000568, -6.000000000000005329, 2.485281374238555774 ) ) ;
#1121=CARTESIAN_POINT ( 'NONE',  ( 161.4367659555122430, -4.821111411827510906, -3.478723816445097317 ) ) ;
#1130=DIRECTION ( 'NONE',  ( -1.387778780781444256E-14, 1.000000000000000000, 0.000000000000000000 ) ) ;
#1134=LINE ( 'NONE', #26929, #11299 ) ;
#1139=CARTESIAN_POINT ( 'NONE',  ( 137.2574251345947971, -2.278174593051671692, 5.500000000000352607 ) ) ;
#1143=CARTESIAN_POINT ( 'NONE',  ( 140.0000000000000284, -54.99999999999990763, -7.500000000000007105 ) ) ;
#1160=ORIENTED_EDGE ( 'NONE', *, *, #676, .T. ) ;
#1163=DIRECTION ( 'NONE',  ( 0.000000000000000000, 1.000000000000000000, -0.000000000000000000 ) ) ;
#1165=ORIENTED_EDGE ( 'NONE', *, *, #26865, .F. ) ;
#1176=DIRECTION ( 'NONE',  ( 1.000000000000000000, 9.251858538542971828E-16, 0.000000000000000000 ) ) ;
#1178=CARTESIAN_POINT ( 'NONE',  ( -0.5000000000000004441, -10.00000000000000888, -8.000000000000007105 ) ) ;
#1180=FACE_OUTER_BOUND ( 'NONE', #15762, .T. ) ;
#1184=CARTESIAN_POINT ( 'NONE',  ( 125.0000000000000568, -55.00000000000000711, 5.000000000000004441 ) ) ;
#1185=ADVANCED_FACE ( 'NONE', ( #11627 ), #23114, .T. ) ;
#1192=VERTEX_POINT ( 'NONE', #25708 ) ;
#1195=AXIS2_PLACEMENT_3D ( 'NONE', #3435, #9936, #26778 ) ;
#1196=CARTESIAN_POINT ( 'NONE',  ( 154.9687500000000284, -2.485281374238585972, 6.000000000000005329 ) ) ;
#1197=( BOUNDED_SURFACE ( )  B_SPLINE_SURFACE ( 3, 2, ( 
 ( #16094, #26975, #5780 ),
 ( #13065, #19641, #10581 ),
 ( #28979, #6104, #24687 ),
 ( #15515, #18378, #17815 ),
 ( #10430, #3327, #25401 ),
 ( #22556, #11320, #4362 ),
 ( #6675, #22095, #22397 ),
 ( #3475, #8989, #24838 ),
 ( #29281, #15194, #1336 ),
 ( #19935, #3787, #5940 ) ),
 .UNSPECIFIED., .F., .F., .T. ) 
 B_SPLINE_SURFACE_WITH_KNOTS ( ( 4, 2, 2, 2, 4 ),
 ( 3, 3 ),
 ( 6.283185307179586232, 6.675884388878310816, 7.068583470577034511, 7.461282552275758206, 7.853981633974482790 ),
 ( 0.000000000000000000, 1.000000000000000000 ),
 .UNSPECIFIED. ) 
 GEOMETRIC_REPRESENTATION_ITEM ( )  RATIONAL_B_SPLINE_SURFACE ( (
 ( 1.000000000000000000, 0.7071067811865475727, 1.000000000000000000),
 ( 1.000000000000000000, 0.7066757001360375323, 1.000000000000000000),
 ( 1.000000000000000000, 0.7265518147277378880, 1.000000000000000000),
 ( 1.000000000000000000, 0.7876784249694658291, 1.000000000000000000),
 ( 1.000000000000000000, 0.8282379786091598195, 1.000000000000000000),
 ( 1.000000000000000000, 0.9038128289597173737, 1.000000000000000000),
 ( 1.000000000000000000, 0.9386556746367764603, 1.000000000000000000),
 ( 1.000000000000000000, 0.9867291651255370999, 1.000000000000000000),
 ( 1.000000000000000000, 1.000158598892032291, 1.000000000000000000),
 ( 1.000000000000000000, 1.000000000000000000, 1.000000000000000000) ) ) 
 REPRESENTATION_ITEM ( '' )  SURFACE ( )  );
#1203=DIRECTION ( 'NONE',  ( 1.000000000000000000, 0.000000000000000000, 0.000000000000000000 ) ) ;
#1206=CARTESIAN_POINT ( 'NONE',  ( 160.3344755113492681, -11.26008890742377311, -4.149533274956910489 ) ) ;
#1207=AXIS2_PLACEMENT_3D ( 'NONE', #21224, #30270, #23233 ) ;
#1208=CARTESIAN_POINT ( 'NONE',  ( 139.6800748654052313, -2.278174593051950136, 5.500000000000074607 ) ) ;
#1209=CARTESIAN_POINT ( 'NONE',  ( 1.000000000000000888, -14.99923475244192339, -9.015151515151522688 ) ) ;
#1213=DIRECTION ( 'NONE',  ( 1.000000000000000000, -3.469446951953694061E-16, 0.000000000000000000 ) ) ;
#1217=COLOUR_RGB ( '', 0.72549020, 0.75294118, 0.79215686) ;
#1224=DIRECTION ( 'NONE',  ( -1.067522139062651904E-16, 1.000000000000000000, 0.000000000000000000 ) ) ;
#1233=CARTESIAN_POINT ( 'NONE',  ( 135.0000000000000284, 0.000000000000000000, 0.000000000000000000 ) ) ;
#1237=CARTESIAN_POINT ( 'NONE',  ( 141.0937500000000000, 6.000000000000005329, 2.485281374238585972 ) ) ;
#1238=EDGE_LOOP ( 'NONE', ( #7077, #14894, #19379, #17896, #8894, #44 ) ) ;
#1244=CARTESIAN_POINT ( 'NONE',  ( 135.6636751345948255, 0.000000000000000000, 5.500000000000005329 ) ) ;
#1247=CARTESIAN_POINT ( 'NONE',  ( 149.3288997308104626, 4.999999999999989342, -2.071067811865468400 ) ) ;
#1249=PLANE ( 'NONE',  #28981 ) ;
#1254=EDGE_CURVE ( 'NONE', #18627, #2002, #13331, .T. ) ;
#1258=ORIENTED_EDGE ( 'NONE', *, *, #14946, .T. ) ;
#1265=CARTESIAN_POINT ( 'NONE',  ( 145.9687500000000284, -2.485281374238585972, 6.000000000000005329 ) ) ;
#1268=MECHANICAL_DESIGN_GEOMETRIC_PRESENTATION_REPRESENTATION('',(#8628),#18972);
#1269=( NAMED_UNIT ( * ) SI_UNIT ( $, .STERADIAN. ) SOLID_ANGLE_UNIT ( ) );
#1272=CARTESIAN_POINT ( 'NONE',  ( 143.5312500000000284, -2.485281374238555774, -6.000000000000005329 ) ) ;
#1279=ORIENTED_EDGE ( 'NONE', *, *, #8303, .F. ) ;
#1284=DIRECTION ( 'NONE',  ( 0.000000000000000000, 0.000000000000000000, -1.000000000000000000 ) ) ;
#1286=CARTESIAN_POINT ( 'NONE',  ( -4.999999999999886313, -10.00000000000000888, -5.000000000000004441 ) ) ;
#1289=EDGE_CURVE ( 'NONE', #6343, #3203, #19120, .T. ) ;
#1295=CARTESIAN_POINT ( 'NONE',  ( 139.5000000000000284, -54.99999999999990763, 7.500000000000007105 ) ) ;
#1296=DIRECTION ( 'NONE',  ( 1.000000000000000000, 0.000000000000000000, 0.000000000000000000 ) ) ;
#1300=CARTESIAN_POINT ( 'NONE',  ( 151.8898502691896510, 3.535533905932725318, -3.535533905932725318 ) ) ;
#1301=CARTESIAN_POINT ( 'NONE',  ( -0.04562205425674009662, -14.50000000000001243, -8.291335958003937634 ) ) ;
#1302=CARTESIAN_POINT ( 'NONE',  ( 139.5000000000000284, -9.165151389911669000, -8.000000000000007105 ) ) ;
#1309=PRESENTATION_STYLE_ASSIGNMENT (( #17177 ) ) ;
#1323=CARTESIAN_POINT ( 'NONE',  ( 135.0000000000000568, -7.635447689476136723, 8.089997508179699537 ) ) ;
#1331=AXIS2_PLACEMENT_3D ( 'NONE', #12013, #28380, #24086 ) ;
#1336=CARTESIAN_POINT ( 'NONE',  ( -0.8690767379103921941, -9.065461631044712476, 4.000000000000005329 ) ) ;
#1340=CYLINDRICAL_SURFACE ( 'NONE', #18262, 5.500000000000000000 ) ;
#1341=CARTESIAN_POINT ( 'NONE',  ( 135.2045928001402331, -8.331920847649417539, 8.143621320507632433 ) ) ;
#1346=AXIS2_PLACEMENT_3D ( 'NONE', #795, #23995, #7698 ) ;
#1348=ORIENTED_EDGE ( 'NONE', *, *, #15602, .T. ) ;
#1349=DIRECTION ( 'NONE',  ( 0.000000000000000000, -1.000000000000000000, 0.000000000000000000 ) ) ;
#1352=CARTESIAN_POINT ( 'NONE',  ( 150.0863248654052313, 0.000000000000000000, 5.500000000000005329 ) ) ;
#1358=CARTESIAN_POINT ( 'NONE',  ( 156.8437500000000284, -6.000000000000005329, -2.485281374238555774 ) ) ;
#1359=EDGE_CURVE ( 'NONE', #1710, #6311, #12374, .T. ) ;
#1363=CARTESIAN_POINT ( 'NONE',  ( 135.5000000000000284, -9.047800747817580813, -7.500000000000007105 ) ) ;
#1367=CARTESIAN_POINT ( 'NONE',  ( 159.4166817098593754, -11.36111566036954912, 3.917249193633611792 ) ) ;
#1369=ORIENTED_EDGE ( 'NONE', *, *, #28211, .F. ) ;
#1373=CARTESIAN_POINT ( 'NONE',  ( 159.6175193642574186, -12.16729450327831685, -3.789279010572755624 ) ) ;
#1381=CARTESIAN_POINT ( 'NONE',  ( 0.000000000000000000, -10.50000000000000888, -8.500000000000007105 ) ) ;
#1384=DIRECTION ( 'NONE',  ( 0.000000000000000000, 0.000000000000000000, 1.000000000000000000 ) ) ;
#1386=CARTESIAN_POINT ( 'NONE',  ( 135.0000000000000284, 1.408343819019456570E-15, 11.00000000000000355 ) ) ;
#1389=VERTEX_POINT ( 'NONE', #9592 ) ;
#1391=CARTESIAN_POINT ( 'NONE',  ( -15.49999999999999289, -54.99999999999990763, -7.500000000000007105 ) ) ;
#1395=VECTOR ( 'NONE', #26129, 1000.000000000000000 ) ;
#1399=CARTESIAN_POINT ( 'NONE',  ( 145.0312500000000568, -2.485281374238555774, -6.000000000000005329 ) ) ;
#1400=EDGE_CURVE ( 'NONE', #12501, #7661, #12527, .T. ) ;
#1405=LINE ( 'NONE', #5849, #3370 ) ;
#1407=CARTESIAN_POINT ( 'NONE',  ( 136.0386751345948255, -5.500000000000005329, 0.000000000000000000 ) ) ;
#1409=CARTESIAN_POINT ( 'NONE',  ( 135.8007686613928229, -8.946933464881634990, -7.999999999999145572 ) ) ;
#1410=CARTESIAN_POINT ( 'NONE',  ( 152.7038997308104342, 2.071067811865468400, 4.999999999999989342 ) ) ;
#1411=DIRECTION ( 'NONE',  ( -1.000000000000000000, -0.000000000000000000, 0.000000000000000000 ) ) ;
#1412=CARTESIAN_POINT ( 'NONE',  ( 124.9999999999999432, -65.00000000000000000, 8.000000000000007105 ) ) ;
#1414=CYLINDRICAL_SURFACE ( 'NONE', #17751, 5.500000000000000000 ) ;
#1425=CARTESIAN_POINT ( 'NONE',  ( 147.1875000000000284, 4.242640687119269671, 4.242640687119298093 ) ) ;
#1429=CARTESIAN_POINT ( 'NONE',  ( 136.7812500000000284, 2.485281374238585972, 6.000000000000005329 ) ) ;
#1430=CARTESIAN_POINT ( 'NONE',  ( 161.3955526468546395, -5.529849536909571484, -2.068640691029946410 ) ) ;
#1431=ORIENTED_EDGE ( 'NONE', *, *, #24879, .F. ) ;
#1432=EDGE_CURVE ( 'NONE', #20260, #3651, #22699, .T. ) ;
#1433=VECTOR ( 'NONE', #26147, 1000.000000000000000 ) ;
#1436=AXIS2_PLACEMENT_3D ( 'NONE', #24413, #622, #5066 ) ;
#1440=ORIENTED_EDGE ( 'NONE', *, *, #20179, .F. ) ;
#1450=CARTESIAN_POINT ( 'NONE',  ( 137.1488248654052313, -3.889087296526011706, -3.889087296526011706 ) ) ;
#1452=UNCERTAINTY_MEASURE_WITH_UNIT (LENGTH_MEASURE( 1.000000000000000082E-05 ), #15146, 'distance_accuracy_value', 'NONE');
#1459=AXIS2_PLACEMENT_3D ( 'NONE', #19531, #5813, #4086 ) ;
#1462=FACE_OUTER_BOUND ( 'NONE', #8697, .T. ) ;
#1464=FACE_OUTER_BOUND ( 'NONE', #26711, .T. ) ;
#1465=DIRECTION ( 'NONE',  ( 1.000000000000000000, 0.000000000000000000, 0.000000000000000000 ) ) ;
#1470=EDGE_CURVE ( 'NONE', #4270, #27080, #6641, .T. ) ;
#1475=ORIENTED_EDGE ( 'NONE', *, *, #16946, .F. ) ;
#1477=STYLED_ITEM ( 'NONE', ( #24794 ), #15922 ) ;
#1478=CARTESIAN_POINT ( 'NONE',  ( 139.6493076922298542, -8.798545334315203803, -8.160000000000000142 ) ) ;
#1481=ORIENTED_EDGE ( 'NONE', *, *, #23519, .F. ) ;
#1484=CARTESIAN_POINT ( 'NONE',  ( 146.8199251345948539, -2.278174593052012309, -5.500000000000012434 ) ) ;
#1491=FACE_BOUND ( 'NONE', #4334, .T. ) ;
#1492=CARTESIAN_POINT ( 'NONE',  ( 135.0000000000000284, -8.851767004199837530, 7.500000047444594919 ) ) ;
#1493=ORIENTED_EDGE ( 'NONE', *, *, #29535, .F. ) ;
#1499=ORIENTED_EDGE ( 'NONE', *, *, #30014, .F. ) ;
#1503=CARTESIAN_POINT ( 'NONE',  ( 149.6175748654052882, 5.500000000000012434, -2.278174593052012309 ) ) ;
#1509=CARTESIAN_POINT ( 'NONE',  ( 154.0312500000000568, -2.485281374238555774, -6.000000000000005329 ) ) ;
#1513=CARTESIAN_POINT ( 'NONE',  ( 156.8363248654052313, 0.000000000000000000, -5.500000000000005329 ) ) ;
#1517=CARTESIAN_POINT ( 'NONE',  ( -4.999999999999990230, -24.99999999999999289, 8.000000000000007105 ) ) ;
#1518=AXIS2_PLACEMENT_3D ( 'NONE', #6966, #23719, #12077 ) ;
#1521=LINE ( 'NONE', #3819, #9306 ) ;
#1522=CARTESIAN_POINT ( 'NONE',  ( 159.6319105802860179, -11.40177967602063269, -3.791719585355142641 ) ) ;
#1523=CARTESIAN_POINT ( 'NONE',  ( 140.3363248654052029, 0.000000000000000000, -5.500000000000005329 ) ) ;
#1529=CARTESIAN_POINT ( 'NONE',  ( 136.0000000000000284, 0.000000000000000000, 0.000000000000000000 ) ) ;
#1534=FACE_OUTER_BOUND ( 'NONE', #3335, .T. ) ;
#1535=EDGE_CURVE ( 'NONE', #19344, #17248, #8802, .T. ) ;
#1542=CARTESIAN_POINT ( 'NONE',  ( 137.8273502691896510, -5.000000000000004441, 0.000000000000000000 ) ) ;
#1548=VECTOR ( 'NONE', #5368, 1000.000000000000000 ) ;
#1549=CARTESIAN_POINT ( 'NONE',  ( 135.0000000000000284, 5.402039670393428139, -2.232486041264207799 ) ) ;
#1553=ORIENTED_EDGE ( 'NONE', *, *, #7638, .F. ) ;
#1555=CARTESIAN_POINT ( 'NONE',  ( 140.9062500000000568, 6.000000000000005329, -2.485281374238555774 ) ) ;
#1562=( NAMED_UNIT ( * ) SI_UNIT ( $, .STERADIAN. ) SOLID_ANGLE_UNIT ( ) );
#1565=CARTESIAN_POINT ( 'NONE',  ( 152.2351497308104342, 3.535533905932725318, -3.535533905932725318 ) ) ;
#1566=CARTESIAN_POINT ( 'NONE',  ( 135.0000000000000284, 1.949781249179022291, 5.142796231657420947 ) ) ;
#1567=DIRECTION ( 'NONE',  ( 0.000000000000000000, -0.8907235428302476832, 0.4545454545454524764 ) ) ;
#1568=DIRECTION ( 'NONE',  ( 1.000000000000000000, 0.000000000000000000, 0.000000000000000000 ) ) ;
#1569=VECTOR ( 'NONE', #12546, 1000.000000000000000 ) ;
#1575=EDGE_CURVE ( 'NONE', #8510, #9581, #30137, .T. ) ;
#1581=CARTESIAN_POINT ( 'NONE',  ( 145.6875000000000284, 4.242640687119269671, 4.242640687119298093 ) ) ;
#1582=DIRECTION ( 'NONE',  ( 0.000000000000000000, -1.000000000000000000, 0.000000000000000000 ) ) ;
#1588=ORIENTED_EDGE ( 'NONE', *, *, #15099, .T. ) ;
#1589=CARTESIAN_POINT ( 'NONE',  ( 139.6875000000000284, 4.242640687119269671, 4.242640687119298093 ) ) ;
#1590=CARTESIAN_POINT ( 'NONE',  ( 161.2720946962140260, -5.187633567512120791, 2.550615076069009834 ) ) ;
#1595=ORIENTED_EDGE ( 'NONE', *, *, #20144, .T. ) ;
#1601=CARTESIAN_POINT ( 'NONE',  ( 147.8363248654052029, 0.000000000000000000, -5.500000000000005329 ) ) ;
#1602=CARTESIAN_POINT ( 'NONE',  ( 135.1170309136356877, -7.914290706147571797, -8.323885487687906704 ) ) ;
#1614=CARTESIAN_POINT ( 'NONE',  ( 151.7023502691896510, 0.000000000000000000, -5.000000000000004441 ) ) ;
#1618=DIRECTION ( 'NONE',  ( 0.000000000000000000, -1.000000000000000000, 0.000000000000000000 ) ) ;
#1619=CARTESIAN_POINT ( 'NONE',  ( 150.5550748654052313, -5.500000000000012434, -2.278174593052012309 ) ) ;
#1622=ORIENTED_EDGE ( 'NONE', *, *, #4777, .T. ) ;
#1623=CARTESIAN_POINT ( 'NONE',  ( 157.4062500000000284, 6.000000000000005329, -2.485281374238555774 ) ) ;
#1624=CARTESIAN_POINT ( 'NONE',  ( -0.004063854759415918595, -15.42149627498952569, 6.273580390957694597 ) ) ;
#1637=CARTESIAN_POINT ( 'NONE',  ( 116.0000000000000142, 6.735557395310442023E-16, 5.500000000000000000 ) ) ;
#1639=CARTESIAN_POINT ( 'NONE',  ( 157.4136751345948539, 0.000000000000000000, -5.500000000000005329 ) ) ;
#1643=CARTESIAN_POINT ( 'NONE',  ( -0.07850599468832326899, -14.93747518635459137, 8.093769840972308671 ) ) ;
#1648=EDGE_CURVE ( 'NONE', #20340, #20437, #27789, .T. ) ;
#1651=CARTESIAN_POINT ( 'NONE',  ( 141.1011751345948539, 3.889087296526011706, -3.889087296526011706 ) ) ;
#1652=CYLINDRICAL_SURFACE ( 'NONE', #16550, 30.00000000000000000 ) ;
#1653=VERTEX_POINT ( 'NONE', #18617 ) ;
#1660=TOROIDAL_SURFACE ( 'NONE', #18861, 15.99999999999999289, 1.000000000000000000 ) ;
#1664=VERTEX_POINT ( 'NONE', #13570 ) ;
#1667=EDGE_LOOP ( 'NONE', ( #23038, #23188, #19873, #8884 ) ) ;
#1668=CARTESIAN_POINT ( 'NONE',  ( 155.9062500000000853, 6.000000000000005329, -2.485281374238555774 ) ) ;
#1677=CARTESIAN_POINT ( 'NONE',  ( 159.9406005586360209, -11.50931141900650978, 3.432783163228085410 ) ) ;
#1679=ORIENTED_EDGE ( 'NONE', *, *, #24279, .T. ) ;
#1680=CARTESIAN_POINT ( 'NONE',  ( 162.0000000000000284, 0.000000000000000000, 0.000000000000000000 ) ) ;
#1681=CARTESIAN_POINT ( 'NONE',  ( 141.0000000000000284, -12.00000000000001066, 4.000000000000003553 ) ) ;
#1682=CARTESIAN_POINT ( 'NONE',  ( 159.2682291426874599, -12.02340987637674097, -3.972341123820091191 ) ) ;
#1689=CARTESIAN_POINT ( 'NONE',  ( -4.999999999999990230, -55.00000000000002132, 8.000000000000007105 ) ) ;
#1690=DIRECTION ( 'NONE',  ( -1.734723475976824844E-16, 1.000000000000000000, 0.000000000000000000 ) ) ;
#1696=CARTESIAN_POINT ( 'NONE',  ( 160.4925748654052597, 2.278174593051894625, 5.500000000000129674 ) ) ;
#1697=CARTESIAN_POINT ( 'NONE',  ( 138.4836002691896510, 4.999999999999989342, -2.071067811865468400 ) ) ;
#1701=( LENGTH_UNIT ( ) NAMED_UNIT ( * ) SI_UNIT ( .MILLI., .METRE. ) );
#1704=CARTESIAN_POINT ( 'NONE',  ( 140.5126264503620916, -11.05212133306707578, -4.674908800639064665 ) ) ;
#1706=VERTEX_POINT ( 'NONE', #21217 ) ;
#1708=CARTESIAN_POINT ( 'NONE',  ( 139.1250000000000284, 0.000000000000000000, -6.000000000000005329 ) ) ;
#1709=B_SPLINE_CURVE_WITH_KNOTS ( 'NONE', 3,
 ( #26383, #5330, #29279, #1643, #20388, #13063, #15828, #11199 ),
 .UNSPECIFIED., .F., .F.,
 ( 4, 2, 2, 4 ),
 ( 0.000000000000000000, 0.0005811766152209535885, 0.0008717649228314284853, 0.001162353230441903491 ),
 .UNSPECIFIED. ) ;
#1710=VERTEX_POINT ( 'NONE', #9537 ) ;
#1711=EDGE_LOOP ( 'NONE', ( #1006, #16931, #8148, #24469 ) ) ;
#1716=CARTESIAN_POINT ( 'NONE',  ( 136.3199251345947971, -2.278174593052089136, -5.499999999999934275 ) ) ;
#1718=CARTESIAN_POINT ( 'NONE',  ( 152.4226497308104058, 5.000000000000004441, 0.000000000000000000 ) ) ;
#1720=CARTESIAN_POINT ( 'NONE',  ( 140.0000000000000284, -12.00000000000001066, 4.000000000000003553 ) ) ;
#1722=SURFACE_STYLE_USAGE ( .BOTH. , #13434 ) ;
#1723=( BOUNDED_SURFACE ( )  B_SPLINE_SURFACE ( 3, 2, ( 
 ( #19669, #7676, #22126 ),
 ( #29316, #5811, #5365 ),
 ( #17087, #7974, #15069 ),
 ( #1068, #26414, #10458 ),
 ( #14773, #8274, #15228 ),
 ( #17688, #27014, #5979 ) ),
 .UNSPECIFIED., .F., .F., .F. ) 
 B_SPLINE_SURFACE_WITH_KNOTS ( ( 4, 2, 4 ),
 ( 3, 3 ),
 ( 0.02423702093288230414, 0.02523827330272541969, 0.02623952567256853524 ),
 ( 0.000000000000000000, 1.000000000000000000 ),
 .UNSPECIFIED. ) 
 GEOMETRIC_REPRESENTATION_ITEM ( )  RATIONAL_B_SPLINE_SURFACE ( (
 ( 1.000000000000000000, 0.7071067811865475727, 1.000000000000000000),
 ( 1.000000000000000000, 0.7329025660702759293, 1.000000000000000000),
 ( 1.000000000000000000, 0.7587231434688260778, 1.000000000000000000),
 ( 1.000000000000000000, 0.8097046771148294075, 1.000000000000000000),
 ( 1.000000000000000000, 0.8349103174451857345, 1.000000000000000000),
 ( 1.000000000000000000, 0.8593225670956807782, 1.000000000000000000) ) ) 
 REPRESENTATION_ITEM ( '' )  SURFACE ( )  );
#1732=VERTEX_POINT ( 'NONE', #11419 ) ;
#1735=CARTESIAN_POINT ( 'NONE',  ( 145.4062500000000284, 6.000000000000005329, -2.485281374238556218 ) ) ;
#1737=DIRECTION ( 'NONE',  ( 0.000000000000000000, 0.000000000000000000, 1.000000000000000000 ) ) ;
#1739=VECTOR ( 'NONE', #11454, 1000.000000000000000 ) ;
#1748=TOROIDAL_SURFACE ( 'NONE', #18963, 16.00000000000000000, 1.000000000000000000 ) ;
#1757=CARTESIAN_POINT ( 'NONE',  ( 139.5000000000000284, -9.165151389911676105, -8.000000000000007105 ) ) ;
#1758=CARTESIAN_POINT ( 'NONE',  ( 156.2738248654052029, -3.889087296526011706, 3.889087296526011706 ) ) ;
#1759=AXIS2_PLACEMENT_3D ( 'NONE', #7502, #24234, #23956 ) ;
#1762=CARTESIAN_POINT ( 'NONE',  ( 149.4523502691896510, 0.000000000000000000, 5.000000000000004441 ) ) ;
#1766=DIRECTION ( 'NONE',  ( 0.000000000000000000, -1.000000000000000000, 0.000000000000000000 ) ) ;
#1771=ORIENTED_EDGE ( 'NONE', *, *, #19013, .T. ) ;
#1772=CARTESIAN_POINT ( 'NONE',  ( 155.3437500000000284, -6.000000000000005329, -2.485281374238555774 ) ) ;
#1779=EDGE_CURVE ( 'NONE', #25181, #20028, #27857, .T. ) ;
#1783=SURFACE_SIDE_STYLE ('',( #1942 ) ) ;
#1792=AXIS2_PLACEMENT_3D ( 'NONE', #5987, #22896, #8917 ) ;
#1796=CARTESIAN_POINT ( 'NONE',  ( 146.2425748654051745, -2.278174593052290753, -5.499999999999732658 ) ) ;
#1798=CARTESIAN_POINT ( 'NONE',  ( 159.5773502691896510, 5.000000000000004441, 0.000000000000000000 ) ) ;
#1800=CARTESIAN_POINT ( 'NONE',  ( -0.06962969976386645943, -14.74801126815780528, 8.209584733985920479 ) ) ;
#1807=DIRECTION ( 'NONE',  ( -1.000000000000000000, -6.938893903907222067E-15, 0.000000000000000000 ) ) ;
#1810=EDGE_LOOP ( 'NONE', ( #11720, #30071, #1258, #8892 ) ) ;
#1811=VECTOR ( 'NONE', #9109, 1000.000000000000000 ) ;
#1813=AXIS2_PLACEMENT_3D ( 'NONE', #14799, #12808, #24141 ) ;
#1815=CARTESIAN_POINT ( 'NONE',  ( 156.3750000000000284, 0.000000000000000000, 6.000000000000005329 ) ) ;
#1820=EDGE_CURVE ( 'NONE', #30157, #28361, #13821, .T. ) ;
#1823=CARTESIAN_POINT ( 'NONE',  ( -4.999999999999990230, -55.00000000000002132, 7.500000000000007105 ) ) ;
#1826=CARTESIAN_POINT ( 'NONE',  ( 116.0000000000000142, 0.000000000000000000, 0.000000000000000000 ) ) ;
#1829=CARTESIAN_POINT ( 'NONE',  ( 0.1950273200666285678, -15.66255992321438129, -7.807776097887585642 ) ) ;
#1832=DIRECTION ( 'NONE',  ( 0.000000000000000000, 0.000000000000000000, 1.000000000000000000 ) ) ;
#1833=FACE_OUTER_BOUND ( 'NONE', #5210, .T. ) ;
#1838=DIRECTION ( 'NONE',  ( 1.000000000000000000, -6.938893903907221278E-15, 0.000000000000000000 ) ) ;
#1840=CARTESIAN_POINT ( 'NONE',  ( -1.000000000000002665, -9.000000000000007105, -4.000000000000005329 ) ) ;
#1842=AXIS2_PLACEMENT_3D ( 'NONE', #17174, #24348, #2706 ) ;
#1848=CARTESIAN_POINT ( 'NONE',  ( 139.6086002691896795, -2.071067811865468400, -4.999999999999989342 ) ) ;
#1854=( BOUNDED_CURVE ( )  B_SPLINE_CURVE ( 2, ( #28256, #9546, #6919, #16345, #11730, #3, #9388, #11888, #18938 ),
 .UNSPECIFIED., .F., .T. ) 
 B_SPLINE_CURVE_WITH_KNOTS ( ( 3, 2, 2, 2, 3 ),
 ( 0.3125000000000007772, 0.3187500000000005329, 0.3250000000000003442, 0.3312500000000000444, 0.3374999999999998557 ),
 .UNSPECIFIED. ) 
 CURVE ( )  GEOMETRIC_REPRESENTATION_ITEM ( )  RATIONAL_B_SPLINE_CURVE ( ( 0.9999999999999905631, 0.9238795325112961754, 1.000000000000000000, 0.9238795325112867385, 1.000000000000000000, 0.9238795325112867385, 1.000000000000000000, 0.9238795325112887369, 0.9999999999999980016 ) ) 
 REPRESENTATION_ITEM ( '' )  );
#1856=ORIENTED_EDGE ( 'NONE', *, *, #21549, .F. ) ;
#1858=CARTESIAN_POINT ( 'NONE',  ( 160.0000000000000000, -12.58734484189959879, 3.130213737083505698 ) ) ;
#1859=CARTESIAN_POINT ( 'NONE',  ( 142.5937500000000568, 6.000000000000005329, 2.485281374238585972 ) ) ;
#1860=AXIS2_PLACEMENT_3D ( 'NONE', #30009, #23122, #20498 ) ;
#1867=FACE_OUTER_BOUND ( 'NONE', #29364, .T. ) ;
#1868=DIRECTION ( 'NONE',  ( 0.000000000000000000, 0.000000000000000000, -1.000000000000000000 ) ) ;
#1870=CARTESIAN_POINT ( 'NONE',  ( 143.7976497308104058, 0.000000000000000000, 5.000000000000004441 ) ) ;
#1874=CARTESIAN_POINT ( 'NONE',  ( 129.9999999999998010, -89.00000000000001421, 4.000000000000003553 ) ) ;
#1878=CARTESIAN_POINT ( 'NONE',  ( 116.0000000000000142, 0.000000000000000000, -5.500000000000000000 ) ) ;
#1887=CARTESIAN_POINT ( 'NONE',  ( 147.5625000000000284, -4.242640687119298093, 4.242640687119298093 ) ) ;
#1888=CARTESIAN_POINT ( 'NONE',  ( 160.7409933946964031, -11.42047333460522474, -3.685613295175590665 ) ) ;
#1891=CARTESIAN_POINT ( 'NONE',  ( 141.0937500000000000, 6.000000000000005329, 2.485281374238585972 ) ) ;
#1898=ORIENTED_EDGE ( 'NONE', *, *, #21254, .T. ) ;
#1910=DIRECTION ( 'NONE',  ( -0.000000000000000000, -0.000000000000000000, -1.000000000000000000 ) ) ;
#1916=CYLINDRICAL_SURFACE ( 'NONE', #246, 1.000000000000000000 ) ;
#1922=DIRECTION ( 'NONE',  ( 0.000000000000000000, -1.000000000000000000, 0.000000000000000000 ) ) ;
#1928=DIRECTION ( 'NONE',  ( 0.000000000000000000, 0.000000000000000000, -1.000000000000000000 ) ) ;
#1929=ORIENTED_EDGE ( 'NONE', *, *, #6081, .F. ) ;
#1930=CIRCLE ( 'NONE', #21567, 11.00000000000000355 ) ;
#1931=CARTESIAN_POINT ( 'NONE',  ( 154.1250000000000284, 0.000000000000000000, -6.000000000000005329 ) ) ;
#1935=VERTEX_POINT ( 'NONE', #329 ) ;
#1936=EDGE_CURVE ( 'NONE', #25911, #13576, #10683, .T. ) ;
#1938=ORIENTED_EDGE ( 'NONE', *, *, #29081, .F. ) ;
#1940=( BOUNDED_CURVE ( )  B_SPLINE_CURVE ( 2, ( #3758, #16104, #27701, #6682, #23138, #6828, #7134 ),
 .UNSPECIFIED., .F., .T. ) 
 B_SPLINE_CURVE_WITH_KNOTS ( ( 3, 2, 2, 3 ),
 ( 0.02366385240269184426, 0.02499999999999995975, 0.03124999999999976755, 0.03749999999999957534 ),
 .UNSPECIFIED. ) 
 CURVE ( )  GEOMETRIC_REPRESENTATION_ITEM ( )  RATIONAL_B_SPLINE_CURVE ( ( 0.9744113160502365645, 0.9837266912414370790, 1.000000000000000000, 0.9238795325112867385, 1.000000000000000000, 0.9238795325112918455, 0.9999999999999948930 ) ) 
 REPRESENTATION_ITEM ( '' )  );
#1942=SURFACE_STYLE_FILL_AREA ( #6545 ) ;
#1947=ORIENTED_EDGE ( 'NONE', *, *, #20230, .F. ) ;
#1950=CIRCLE ( 'NONE', #25490, 1.000000000000000000 ) ;
#1954=AXIS2_PLACEMENT_3D ( 'NONE', #14886, #23796, #2730 ) ;
#1958=CARTESIAN_POINT ( 'NONE',  ( -19.49999999999998224, -25.00000000000010658, 7.500000000000007105 ) ) ;
#1960=CARTESIAN_POINT ( 'NONE',  ( 159.0148502691896510, -3.535533905932725318, -3.535533905932725318 ) ) ;
#1961=CARTESIAN_POINT ( 'NONE',  ( 0.8347181576680260395, -15.41331385233628382, 8.287403863818649796 ) ) ;
#1967=CARTESIAN_POINT ( 'NONE',  ( 157.7886751345948255, 5.500000000000005329, 0.000000000000000000 ) ) ;
#1971=MECHANICAL_DESIGN_GEOMETRIC_PRESENTATION_REPRESENTATION('',(#20620),#8337);
#1972=ORIENTED_EDGE ( 'NONE', *, *, #12405, .F. ) ;
#1974=EDGE_CURVE ( 'NONE', #21999, #20568, #22925, .T. ) ;
#1975=CARTESIAN_POINT ( 'NONE',  ( 148.6875000000000284, 4.242640687119269671, 4.242640687119298093 ) ) ;
#1980=CARTESIAN_POINT ( 'NONE',  ( 157.1175748654052029, 5.500000000000012434, -2.278174593052012309 ) ) ;
#1987=DIRECTION ( 'NONE',  ( 1.000000000000000000, 0.000000000000000000, 0.000000000000000000 ) ) ;
#1988=CARTESIAN_POINT ( 'NONE',  ( -0.5000000000000004441, -15.00000000000001421, 8.000000000000007105 ) ) ;
#1997=CARTESIAN_POINT ( 'NONE',  ( 160.4913278202574247, -11.31223276408536549, -4.005158905402271152 ) ) ;
#2000=DIRECTION ( 'NONE',  ( -1.067522139062651904E-16, 1.000000000000000000, 0.000000000000000000 ) ) ;
#2001=CARTESIAN_POINT ( 'NONE',  ( 139.5000000000000000, -9.165151389911669000, 8.500000000000007105 ) ) ;
#2002=VERTEX_POINT ( 'NONE', #12956 ) ;
#2005=CARTESIAN_POINT ( 'NONE',  ( -15.49999999999999289, -54.99999999999990763, -8.000000000000007105 ) ) ;
#2006=CARTESIAN_POINT ( 'NONE',  ( 136.2336002691896510, -4.999999999999989342, 2.071067811865468400 ) ) ;
#2008=ORIENTED_EDGE ( 'NONE', *, *, #12210, .F. ) ;
#2019=CARTESIAN_POINT ( 'NONE',  ( 135.6562500000000284, -6.000000000000005329, 2.485281374238555774 ) ) ;
#2020=AXIS2_PLACEMENT_3D ( 'NONE', #19418, #29051, #7422 ) ;
#2023=AXIS2_PLACEMENT_3D ( 'NONE', #27438, #18124, #1807 ) ;
#2024=AXIS2_PLACEMENT_3D ( 'NONE', #28082, #5188, #588 ) ;
#2025=DIRECTION ( 'NONE',  ( -1.000000000000000000, 3.469446951953694061E-16, -0.000000000000000000 ) ) ;
#2027=SURFACE_SIDE_STYLE ('',( #25198 ) ) ;
#2030=CARTESIAN_POINT ( 'NONE',  ( 134.9985123063133869, -7.386692690749734780, -8.423607852771413107 ) ) ;
#2031=CARTESIAN_POINT ( 'NONE',  ( 142.4851497308104058, -3.535533905932725318, 3.535533905932725318 ) ) ;
#2032=CARTESIAN_POINT ( 'NONE',  ( 0.000000000000000000, 11.00000000000001066, 3.000000000000002665 ) ) ;
#2043=PRESENTATION_STYLE_ASSIGNMENT (( #27968 ) ) ;
#2045=COLOUR_RGB ( '', 0.09019608, 0.27058824, 0.51372549) ;
#2046=EDGE_CURVE ( 'NONE', #29814, #10891, #21251, .T. ) ;
#2051=( BOUNDED_CURVE ( )  B_SPLINE_CURVE ( 2, ( #6170, #20309, #10807, #6006, #6465, #18175, #15582, #23078, #24895 ),
 .UNSPECIFIED., .F., .T. ) 
 B_SPLINE_CURVE_WITH_KNOTS ( ( 3, 2, 2, 2, 3 ),
 ( 0.1874999999999996947, 0.1937499999999994504, 0.1999999999999991784, 0.2062499999999990452, 0.2124999999999988010 ),
 .UNSPECIFIED. ) 
 CURVE ( )  GEOMETRIC_REPRESENTATION_ITEM ( )  RATIONAL_B_SPLINE_CURVE ( ( 1.000000000000003775, 0.9238795325112830747, 1.000000000000000000, 0.9238795325112867385, 1.000000000000000000, 0.9238795325112867385, 1.000000000000000000, 0.9238795325113016155, 0.9999999999999851230 ) ) 
 REPRESENTATION_ITEM ( '' )  );
#2053=AXIS2_PLACEMENT_3D ( 'NONE', #21662, #12021, #441 ) ;
#2055=CARTESIAN_POINT ( 'NONE',  ( 139.1250000000000284, 0.000000000000000000, -6.000000000000005329 ) ) ;
#2056=CARTESIAN_POINT ( 'NONE',  ( 160.0000000000000284, -12.64911064067350566, -3.000000000000002665 ) ) ;
#2059=CARTESIAN_POINT ( 'NONE',  ( 138.1875000000000284, 4.242640687119269671, 4.242640687119298093 ) ) ;
#2062=CIRCLE ( 'NONE', #19237, 0.5000000000000000000 ) ;
#2068=CIRCLE ( 'NONE', #29054, 1.000000000000000888 ) ;
#2070=CARTESIAN_POINT ( 'NONE',  ( -0.7071067811865482389, -9.585786437626913070, -4.000000000000004441 ) ) ;
#2071=CARTESIAN_POINT ( 'NONE',  ( 116.0000000000000142, 0.000000000000000000, 0.000000000000000000 ) ) ;
#2072=CARTESIAN_POINT ( 'NONE',  ( 0.000000000000000000, 0.000000000000000000, 5.000000000000004441 ) ) ;
#2076=CARTESIAN_POINT ( 'NONE',  ( -14.99999999999999289, -25.00000000000007816, 8.000000000000007105 ) ) ;
#2079=( LENGTH_UNIT ( ) NAMED_UNIT ( * ) SI_UNIT ( .MILLI., .METRE. ) );
#2081=EDGE_CURVE ( 'NONE', #17791, #22266, #26800, .T. ) ;
#2083=CARTESIAN_POINT ( 'NONE',  ( 147.3898502691896510, 3.535533905932725318, -3.535533905932725318 ) ) ;
#2086=CARTESIAN_POINT ( 'NONE',  ( 157.0312500000000568, -2.485281374238556218, -6.000000000000005329 ) ) ;
#2087=DIRECTION ( 'NONE',  ( 1.000000000000000000, 0.000000000000000000, 0.000000000000000000 ) ) ;
#2092=CARTESIAN_POINT ( 'NONE',  ( 158.5312500000000284, -2.485281374238555774, -6.000000000000005329 ) ) ;
#2093=FACE_OUTER_BOUND ( 'NONE', #12186, .T. ) ;
#2107=CARTESIAN_POINT ( 'NONE',  ( 136.0000000000000284, -9.165151389911669000, 8.000000000000007105 ) ) ;
#2111=DIRECTION ( 'NONE',  ( 1.000000000000000000, 0.000000000000000000, 0.000000000000000000 ) ) ;
#2116=CARTESIAN_POINT ( 'NONE',  ( 145.8675748654052313, -5.500000000000012434, 2.278174593052012309 ) ) ;
#2119=CARTESIAN_POINT ( 'NONE',  ( 162.3898502691896510, 3.535533905932725318, -3.535533905932725318 ) ) ;
#2120=CARTESIAN_POINT ( 'NONE',  ( 135.0000000000000284, -7.310118669088633503, 8.297092313840531475 ) ) ;
#2126=DIRECTION ( 'NONE',  ( 0.000000000000000000, 0.000000000000000000, 1.000000000000000000 ) ) ;
#2127=EDGE_LOOP ( 'NONE', ( #2247, #600, #24235, #26920 ) ) ;
#2131=DIRECTION ( 'NONE',  ( -0.000000000000000000, -0.000000000000000000, -1.000000000000000000 ) ) ;
#2133=VECTOR ( 'NONE', #5155, 1000.000000000000000 ) ;
#2134=CIRCLE ( 'NONE', #6042, 0.5000000000000004441 ) ;
#2135=CARTESIAN_POINT ( 'NONE',  ( 152.9062500000000000, 6.000000000000005329, -2.485281374238555774 ) ) ;
#2136=ORIENTED_EDGE ( 'NONE', *, *, #29691, .T. ) ;
#2145=CARTESIAN_POINT ( 'NONE',  ( 160.0000000000000284, -12.58795266400503365, 3.128932333554976797 ) ) ;
#2149=FACE_OUTER_BOUND ( 'NONE', #11451, .T. ) ;
#2156=CARTESIAN_POINT ( 'NONE',  ( -0.7481905315629638897, -9.503618936874122625, -4.126213593628788701 ) ) ;
#2159=EDGE_CURVE ( 'NONE', #29595, #25966, #14183, .T. ) ;
#2162=DIRECTION ( 'NONE',  ( -0.000000000000000000, -0.000000000000000000, -1.000000000000000000 ) ) ;
#2165=ORIENTED_EDGE ( 'NONE', *, *, #23927, .T. ) ;
#2167=ORIENTED_EDGE ( 'NONE', *, *, #21263, .T. ) ;
#2172=EDGE_LOOP ( 'NONE', ( #12798, #3021, #17719, #29733 ) ) ;
#2175=CARTESIAN_POINT ( 'NONE',  ( 137.5312500000000284, -2.485281374238555774, -6.000000000000005329 ) ) ;
#2177=DIRECTION ( 'NONE',  ( 1.000000000000000000, 0.000000000000000000, 0.000000000000000000 ) ) ;
#2179=ADVANCED_FACE ( 'NONE', ( #14033 ), #25806, .T. ) ;
#2182=DIRECTION ( 'NONE',  ( -0.000000000000000000, -0.000000000000000000, -1.000000000000000000 ) ) ;
#2184=CARTESIAN_POINT ( 'NONE',  ( 144.8288997308104058, 4.999999999999989342, -2.071067811865468400 ) ) ;
#2188=CARTESIAN_POINT ( 'NONE',  ( 156.3824251345947971, 5.500000000000012434, 2.278174593052012309 ) ) ;
#2195=CARTESIAN_POINT ( 'NONE',  ( 140.5000000000000284, 0.000000000000000000, 0.000000000000000000 ) ) ;
#2197=ORIENTED_EDGE ( 'NONE', *, *, #29081, .T. ) ;
#2201=CARTESIAN_POINT ( 'NONE',  ( -15.49999999999999289, -25.00000000000007816, 8.000000000000007105 ) ) ;
#2204=CARTESIAN_POINT ( 'NONE',  ( 143.0625000000000284, -4.242640687119298093, 4.242640687119298093 ) ) ;
#2207=CARTESIAN_POINT ( 'NONE',  ( 143.1636751345948255, 0.000000000000000000, 5.500000000000005329 ) ) ;
#2208=CARTESIAN_POINT ( 'NONE',  ( 132.4687500000000284, -2.485281374238585972, 6.000000000000005329 ) ) ;
#2210=ORIENTED_EDGE ( 'NONE', *, *, #26698, .F. ) ;
#2213=EDGE_LOOP ( 'NONE', ( #24247, #3446, #20523, #13445 ) ) ;
#2216=EDGE_CURVE ( 'NONE', #20260, #9814, #23063, .T. ) ;
#2218=CARTESIAN_POINT ( 'NONE',  ( -19.49999999999998224, -54.99999999999990763, -7.500000000000007105 ) ) ;
#2220=ADVANCED_FACE ( 'NONE', ( #30106 ), #27475, .F. ) ;
#2228=CARTESIAN_POINT ( 'NONE',  ( 139.7119292434102249, -8.976731581292797912, -7.966772205599107259 ) ) ;
#2237=CARTESIAN_POINT ( 'NONE',  ( 148.1398502691896510, -3.535533905932752852, 3.535533905932725318 ) ) ;
#2239=DIRECTION ( 'NONE',  ( 0.000000000000000000, 0.000000000000000000, -1.000000000000000000 ) ) ;
#2240=CARTESIAN_POINT ( 'NONE',  ( 160.0312500000000284, -2.485281374238556218, -6.000000000000005329 ) ) ;
#2241=SURFACE_STYLE_FILL_AREA ( #9299 ) ;
#2246=FACE_OUTER_BOUND ( 'NONE', #26085, .T. ) ;
#2247=ORIENTED_EDGE ( 'NONE', *, *, #8554, .T. ) ;
#2248=CARTESIAN_POINT ( 'NONE',  ( 155.0625000000000284, -4.242640687119298093, 4.242640687119298093 ) ) ;
#2252=VERTEX_POINT ( 'NONE', #18770 ) ;
#2253=VECTOR ( 'NONE', #9934, 1000.000000000000000 ) ;
#2259=DIRECTION ( 'NONE',  ( 0.000000000000000000, 0.000000000000000000, -1.000000000000000000 ) ) ;
#2260=CARTESIAN_POINT ( 'NONE',  ( 1.000000000000000888, -14.14213562373095634, -8.500000000000007105 ) ) ;
#2262=ORIENTED_EDGE ( 'NONE', *, *, #18472, .F. ) ;
#2268=( BOUNDED_CURVE ( )  B_SPLINE_CURVE ( 2, ( #1523, #27321, #13396, #8445, #6284, #24872, #22281, #1208, #10461 ),
 .UNSPECIFIED., .F., .F. ) 
 B_SPLINE_CURVE_WITH_KNOTS ( ( 3, 2, 2, 2, 3 ),
 ( 0.7125000000000011324, 0.7187500000000008882, 0.7250000000000006439, 0.7312500000000003997, 0.7375000000000002665 ),
 .UNSPECIFIED. ) 
 CURVE ( )  GEOMETRIC_REPRESENTATION_ITEM ( )  RATIONAL_B_SPLINE_CURVE ( ( 0.9999999999999864553, 0.9238795325113002832, 1.000000000000000000, 0.9238795325112867385, 1.000000000000000000, 0.9238795325112867385, 1.000000000000000000, 0.9238795325112840739, 1.000000000000002665 ) ) 
 REPRESENTATION_ITEM ( '' )  );
#2272=( NAMED_UNIT ( * ) SI_UNIT ( $, .STERADIAN. ) SOLID_ANGLE_UNIT ( ) );
#2273=CARTESIAN_POINT ( 'NONE',  ( 151.4136751345948539, 0.000000000000000000, -5.500000000000005329 ) ) ;
#2275=CIRCLE ( 'NONE', #11624, 30.00000000000000000 ) ;
#2281=ORIENTED_EDGE ( 'NONE', *, *, #27299, .T. ) ;
#2285=EDGE_CURVE ( 'NONE', #27416, #2984, #9679, .T. ) ;
#2287=ORIENTED_EDGE ( 'NONE', *, *, #21549, .T. ) ;
#2288=CARTESIAN_POINT ( 'NONE',  ( 153.0937500000000284, 6.000000000000005329, 2.485281374238585972 ) ) ;
#2292=EDGE_CURVE ( 'NONE', #4004, #11247, #822, .T. ) ;
#2294=ORIENTED_EDGE ( 'NONE', *, *, #5521, .T. ) ;
#2295=DIRECTION ( 'NONE',  ( 1.000000000000000000, -0.000000000000000000, -0.000000000000000000 ) ) ;
#2298=VECTOR ( 'NONE', #2025, 1000.000000000000000 ) ;
#2299=( GEOMETRIC_REPRESENTATION_CONTEXT ( 3 ) GLOBAL_UNCERTAINTY_ASSIGNED_CONTEXT ( ( #14584 ) ) GLOBAL_UNIT_ASSIGNED_CONTEXT ( ( #913, #468, #12790 ) ) REPRESENTATION_CONTEXT ( 'NONE', 'WORKASPACE' ) );
#2301=CARTESIAN_POINT ( 'NONE',  ( -0.08259260911911876779, -15.14630466264630648, -7.836667287028713957 ) ) ;
#2307=CARTESIAN_POINT ( 'NONE',  ( -0.8690767379103921941, -9.065461631044712476, -4.000000000000005329 ) ) ;
#2313=CIRCLE ( 'NONE', #11665, 12.00000000000000178 ) ;
#2319=CONICAL_SURFACE ( 'NONE', #19486, 5.500000000000000000, 0.7853981633974369547 ) ;
#2324=SURFACE_STYLE_FILL_AREA ( #23378 ) ;
#2327=ORIENTED_EDGE ( 'NONE', *, *, #19995, .F. ) ;
#2328=VERTEX_POINT ( 'NONE', #11249 ) ;
#2330=CARTESIAN_POINT ( 'NONE',  ( 136.5937500000000853, 6.000000000000005329, 2.485281374238585972 ) ) ;
#2335=FACE_OUTER_BOUND ( 'NONE', #11656, .T. ) ;
#2339=DIRECTION ( 'NONE',  ( 1.000000000000000000, 0.000000000000000000, 0.000000000000000000 ) ) ;
#2340=CARTESIAN_POINT ( 'NONE',  ( 145.9538997308103774, -2.071067811865468400, -4.999999999999989342 ) ) ;
#2343=CARTESIAN_POINT ( 'NONE',  ( 146.9136751345948539, 0.000000000000000000, -5.500000000000005329 ) ) ;
#2347=CARTESIAN_POINT ( 'NONE',  ( -14.99999999999999289, -54.99999999999990763, -7.500000000000007105 ) ) ;
#2349=DIRECTION ( 'NONE',  ( 0.000000000000000000, 0.000000000000000000, -1.000000000000000000 ) ) ;
#2350=ORIENTED_EDGE ( 'NONE', *, *, #29699, .F. ) ;
#2356=CARTESIAN_POINT ( 'NONE',  ( 137.3437500000000284, -6.000000000000005329, -2.485281374238556218 ) ) ;
#2359=VECTOR ( 'NONE', #6119, 1000.000000000000000 ) ;
#2360=CARTESIAN_POINT ( 'NONE',  ( 160.8601497308104058, -3.535533905932725318, -3.535533905932725318 ) ) ;
#2364=ADVANCED_FACE ( 'NONE', ( #24098 ), #598, .F. ) ;
#2366=EDGE_CURVE ( 'NONE', #8039, #28361, #299, .T. ) ;
#2367=VERTEX_POINT ( 'NONE', #21807 ) ;
#2372=CARTESIAN_POINT ( 'NONE',  ( 152.4449251345948824, -5.500000000000012434, 2.278174593052012309 ) ) ;
#2377=CARTESIAN_POINT ( 'NONE',  ( 139.6502262449442924, -9.198487685513971002, -7.982156388384278323 ) ) ;
#2383=FILL_AREA_STYLE ('',( #9602 ) ) ;
#2384=CARTESIAN_POINT ( 'NONE',  ( 158.7187500000000284, 2.485281374238556218, -6.000000000000005329 ) ) ;
#2390=VERTEX_POINT ( 'NONE', #9534 ) ;
#2391=CARTESIAN_POINT ( 'NONE',  ( 147.8437500000000284, -6.000000000000005329, -2.485281374238555774 ) ) ;
#2394=EDGE_LOOP ( 'NONE', ( #2136, #24211, #9224, #3417 ) ) ;
#2404=FILL_AREA_STYLE ('',( #7155 ) ) ;
#2405=CARTESIAN_POINT ( 'NONE',  ( 158.3288997308104058, 4.999999999999989342, -2.071067811865468400 ) ) ;
#2408=CARTESIAN_POINT ( 'NONE',  ( 135.8344003793675085, -8.798545317550690470, 8.160000018076395634 ) ) ;
#2419=SURFACE_STYLE_FILL_AREA ( #9335 ) ;
#2420=CARTESIAN_POINT ( 'NONE',  ( 134.9999999999997158, -6.982120021892662898, 8.500000000000007105 ) ) ;
#2421=ORIENTED_EDGE ( 'NONE', *, *, #20777, .F. ) ;
#2427=CARTESIAN_POINT ( 'NONE',  ( 157.9761751345948255, 3.889087296526011706, 3.889087296526011706 ) ) ;
#2429=VERTEX_POINT ( 'NONE', #2603 ) ;
#2436=CARTESIAN_POINT ( 'NONE',  ( 152.2500000000000284, -6.000000000000005329, 0.000000000000000000 ) ) ;
#2443=CARTESIAN_POINT ( 'NONE',  ( 158.9925748654052313, 2.278174593051907504, 5.500000000000116351 ) ) ;
#2444=CIRCLE ( 'NONE', #1436, 14.49999999999999822 ) ;
#2447=CARTESIAN_POINT ( 'NONE',  ( 133.2976497308104058, 0.000000000000000000, 5.000000000000004441 ) ) ;
#2448=ORIENTED_EDGE ( 'NONE', *, *, #9048, .F. ) ;
#2450=DIRECTION ( 'NONE',  ( 0.000000000000000000, 0.000000000000000000, 1.000000000000000000 ) ) ;
#2456=CARTESIAN_POINT ( 'NONE',  ( 134.9999999999992895, -6.982120021884474781, -8.500000000000007105 ) ) ;
#2460=CARTESIAN_POINT ( 'NONE',  ( 0.000000000000000000, -15.50000000000001421, -5.656854249492387687 ) ) ;
#2461=DIRECTION ( 'NONE',  ( 0.000000000000000000, 0.000000000000000000, 1.000000000000000000 ) ) ;
#2462=CARTESIAN_POINT ( 'NONE',  ( 135.0000000000000000, 1.949781249179272091, -5.142796231657337458 ) ) ;
#2464=ORIENTED_EDGE ( 'NONE', *, *, #16603, .F. ) ;
#2473=CARTESIAN_POINT ( 'NONE',  ( 134.9062500000000284, 6.000000000000005329, -2.485281374238555774 ) ) ;
#2479=CARTESIAN_POINT ( 'NONE',  ( 143.3288997308104911, 4.999999999999989342, -2.071067811865468400 ) ) ;
#2481=LINE ( 'NONE', #16056, #19708 ) ;
#2492=ORIENTED_EDGE ( 'NONE', *, *, #12853, .T. ) ;
#2494=CARTESIAN_POINT ( 'NONE',  ( 140.1562500000000568, -6.000000000000005329, 2.485281374238556218 ) ) ;
#2496=AXIS2_PLACEMENT_3D ( 'NONE', #19663, #3507, #12624 ) ;
#2498=CARTESIAN_POINT ( 'NONE',  ( 159.8288997308104058, 4.999999999999989342, -2.071067811865468400 ) ) ;
#2500=ORIENTED_EDGE ( 'NONE', *, *, #21909, .T. ) ;
#2504=CARTESIAN_POINT ( 'NONE',  ( 140.3511751345948255, -3.889087296526011706, 3.889087296526011706 ) ) ;
#2507=DIRECTION ( 'NONE',  ( 1.000000000000000000, 0.000000000000000000, 0.000000000000000000 ) ) ;
#2508=ADVANCED_FACE ( 'NONE', ( #15948 ), #8848, .F. ) ;
#2514=CARTESIAN_POINT ( 'NONE',  ( 139.6067523651853151, -8.946933530859819683, 7.999999965039304328 ) ) ;
#2521=EDGE_CURVE ( 'NONE', #14299, #26206, #15206, .T. ) ;
#2523=EDGE_CURVE ( 'NONE', #15395, #9180, #5366, .T. ) ;
#2524=CARTESIAN_POINT ( 'NONE',  ( 143.0773502691896510, 5.000000000000004441, 0.000000000000000000 ) ) ;
#2526=CARTESIAN_POINT ( 'NONE',  ( 155.2500000000000284, -6.000000000000005329, 0.000000000000000000 ) ) ;
#2527=FACE_OUTER_BOUND ( 'NONE', #25917, .T. ) ;
#2529=SURFACE_SIDE_STYLE ('',( #23741 ) ) ;
#2535=CARTESIAN_POINT ( 'NONE',  ( 147.3750000000000284, 0.000000000000000000, 6.000000000000005329 ) ) ;
#2541=ORIENTED_EDGE ( 'NONE', *, *, #18260, .T. ) ;
#2546=CARTESIAN_POINT ( 'NONE',  ( 155.0476497308104342, 0.000000000000000000, -5.000000000000004441 ) ) ;
#2560=CARTESIAN_POINT ( 'NONE',  ( 156.1086002691896510, -2.071067811865468400, -4.999999999999989342 ) ) ;
#2562=EDGE_LOOP ( 'NONE', ( #24072, #13087, #479, #12346 ) ) ;
#2568=CARTESIAN_POINT ( 'NONE',  ( 161.0872520967092782, 0.6323632113212951378, 5.560287570051549721 ) ) ;
#2569=( BOUNDED_CURVE ( )  B_SPLINE_CURVE ( 2, ( #3185, #5194, #12609, #2894, #5640, #12461, #21803, #10283, #19358 ),
 .UNSPECIFIED., .F., .T. ) 
 B_SPLINE_CURVE_WITH_KNOTS ( ( 3, 2, 2, 2, 3 ),
 ( 0.5374999999999999778, 0.5437499999999997335, 0.5499999999999996003, 0.5562499999999993561, 0.5624999999999991118 ),
 .UNSPECIFIED. ) 
 CURVE ( )  GEOMETRIC_REPRESENTATION_ITEM ( )  RATIONAL_B_SPLINE_CURVE ( ( 1.000000000000000000, 0.9238795325112867385, 1.000000000000000000, 0.9238795325112867385, 1.000000000000000000, 0.9238795325112867385, 1.000000000000000000, 0.9238795325112975076, 0.9999999999999892308 ) ) 
 REPRESENTATION_ITEM ( '' )  );
#2571=DIRECTION ( 'NONE',  ( 1.000000000000000000, 0.000000000000000000, 0.000000000000000000 ) ) ;
#2572=LINE ( 'NONE', #21325, #18737 ) ;
#2575=CARTESIAN_POINT ( 'NONE',  ( 149.2500000000000284, -6.000000000000005329, 0.000000000000000000 ) ) ;
#2580=EDGE_LOOP ( 'NONE', ( #15203, #2944 ) ) ;
#2584=( NAMED_UNIT ( * ) PLANE_ANGLE_UNIT ( ) SI_UNIT ( $, .RADIAN. ) );
#2585=EDGE_CURVE ( 'NONE', #5920, #379, #5587, .T. ) ;
#2587=CARTESIAN_POINT ( 'NONE',  ( -0.08237010255012430782, -15.17881940287713149, -7.764910707444049542 ) ) ;
#2595=CARTESIAN_POINT ( 'NONE',  ( 160.7876825596520405, -11.44597140916194711, -3.606058123595494713 ) ) ;
#2596=UNCERTAINTY_MEASURE_WITH_UNIT (LENGTH_MEASURE( 1.000000000000000082E-05 ), #27730, 'distance_accuracy_value', 'NONE');
#2602=CARTESIAN_POINT ( 'NONE',  ( -0.02761656219841567006, -15.32973869486954754, 6.905504754228253717 ) ) ;
#2603=CARTESIAN_POINT ( 'NONE',  ( -39.99999999999998579, -59.99999999999980105, -3.000000000000002665 ) ) ;
#2605=AXIS2_PLACEMENT_3D ( 'NONE', #117, #9498, #28203 ) ;
#2607=( NAMED_UNIT ( * ) PLANE_ANGLE_UNIT ( ) SI_UNIT ( $, .RADIAN. ) );
#2610=CARTESIAN_POINT ( 'NONE',  ( 159.0000000000000284, -12.00000000000001066, -4.000000000000003553 ) ) ;
#2615=CARTESIAN_POINT ( 'NONE',  ( 136.7812500000000284, 2.485281374238585972, 6.000000000000005329 ) ) ;
#2623=PLANE ( 'NONE',  #11819 ) ;
#2626=CARTESIAN_POINT ( 'NONE',  ( 136.2976497308104058, 0.000000000000000000, 5.000000000000004441 ) ) ;
#2627=CARTESIAN_POINT ( 'NONE',  ( 137.8988248654052313, 3.889087296526011706, 3.889087296526011706 ) ) ;
#2637=CARTESIAN_POINT ( 'NONE',  ( 135.5000000000000284, -54.99999999999993605, -8.000000000000007105 ) ) ;
#2638=EDGE_LOOP ( 'NONE', ( #17869, #15243, #6960, #18367 ) ) ;
#2640=CARTESIAN_POINT ( 'NONE',  ( 139.6875000000000284, 4.242640687119269671, 4.242640687119298093 ) ) ;
#2644=CARTESIAN_POINT ( 'NONE',  ( 159.2663997308104058, -4.999999999999989342, -2.071067811865468400 ) ) ;
#2646=EDGE_CURVE ( 'NONE', #16115, #1732, #29138, .T. ) ;
#2648=VERTEX_POINT ( 'NONE', #22256 ) ;
#2655=EDGE_CURVE ( 'NONE', #16741, #19034, #20264, .T. ) ;
#2657=CARTESIAN_POINT ( 'NONE',  ( 140.8531441848274710, -11.85314418482602150, -4.000138456839524181 ) ) ;
#2660=CARTESIAN_POINT ( 'NONE',  ( 140.1568281512133183, -9.009466367372738205, 7.926673930277594593 ) ) ;
#2668=CARTESIAN_POINT ( 'NONE',  ( 158.8125000000000284, 4.242640687119298093, -4.242640687119298093 ) ) ;
#2669=DIRECTION ( 'NONE',  ( 1.000000000000000000, 1.387778780781444413E-14, 0.000000000000000000 ) ) ;
#2670=( LENGTH_UNIT ( ) NAMED_UNIT ( * ) SI_UNIT ( .MILLI., .METRE. ) );
#2673=DIRECTION ( 'NONE',  ( 1.000000000000000000, -0.000000000000000000, -0.000000000000000000 ) ) ;
#2675=CARTESIAN_POINT ( 'NONE',  ( 149.3437500000000284, -6.000000000000005329, -2.485281374238555774 ) ) ;
#2678=FACE_OUTER_BOUND ( 'NONE', #30205, .T. ) ;
#2690=CARTESIAN_POINT ( 'NONE',  ( 154.5788997308104058, -4.999999999999989342, 2.071067811865468400 ) ) ;
#2700=DIRECTION ( 'NONE',  ( 1.000000000000000000, -3.469446951953694061E-16, 0.000000000000000000 ) ) ;
#2702=CARTESIAN_POINT ( 'NONE',  ( 155.4523502691896510, 0.000000000000000000, 5.000000000000004441 ) ) ;
#2706=DIRECTION ( 'NONE',  ( 0.000000000000000000, 0.000000000000000000, -1.000000000000000000 ) ) ;
#2714=CARTESIAN_POINT ( 'NONE',  ( 145.7812500000000284, 2.485281374238585972, 6.000000000000005329 ) ) ;
#2715=EDGE_LOOP ( 'NONE', ( #27835, #18399, #6894, #21530 ) ) ;
#2719=EDGE_CURVE ( 'NONE', #1935, #7475, #10031, .T. ) ;
#2722=DIRECTION ( 'NONE',  ( -1.000000000000000000, 0.000000000000000000, 0.000000000000000000 ) ) ;
#2725=CARTESIAN_POINT ( 'NONE',  ( 133.9538997308104342, -2.071067811865468400, -4.999999999999989342 ) ) ;
#2730=DIRECTION ( 'NONE',  ( 0.000000000000000000, 0.000000000000000000, -1.000000000000000000 ) ) ;
#2738=FACE_OUTER_BOUND ( 'NONE', #22689, .T. ) ;
#2740=EDGE_LOOP ( 'NONE', ( #7967, #11336, #27256, #978 ) ) ;
#2742=VECTOR ( 'NONE', #12531, 1000.000000000000000 ) ;
#2743=DIRECTION ( 'NONE',  ( 1.000000000000000000, 0.000000000000000000, 0.000000000000000000 ) ) ;
#2758=EDGE_LOOP ( 'NONE', ( #26210, #2327, #29337, #1440 ) ) ;
#2759=FACE_OUTER_BOUND ( 'NONE', #18505, .T. ) ;
#2760=CARTESIAN_POINT ( 'NONE',  ( 160.1250000000000568, 0.000000000000000000, -6.000000000000005329 ) ) ;
#2767=CARTESIAN_POINT ( 'NONE',  ( -4.999999999999886313, -70.00000000000001421, 5.000000000000004441 ) ) ;
#2768=DIRECTION ( 'NONE',  ( 0.000000000000000000, 0.000000000000000000, -1.000000000000000000 ) ) ;
#2770=CARTESIAN_POINT ( 'NONE',  ( 135.3601497308104342, -3.535533905932725318, -3.535533905932725318 ) ) ;
#2774=DIRECTION ( 'NONE',  ( -1.000000000000000000, 1.387778780781444413E-14, 0.000000000000000000 ) ) ;
#2779=ORIENTED_EDGE ( 'NONE', *, *, #3365, .F. ) ;
#2781=DIRECTION ( 'NONE',  ( 0.000000000000000000, 0.000000000000000000, 1.000000000000000000 ) ) ;
#2791=CARTESIAN_POINT ( 'NONE',  ( 135.0000000000000284, 6.000000000000005329, 0.000000000000000000 ) ) ;
#2793=VECTOR ( 'NONE', #191, 1000.000000000000000 ) ;
#2796=ORIENTED_EDGE ( 'NONE', *, *, #1289, .T. ) ;
#2810=DIRECTION ( 'NONE',  ( 0.000000000000000000, 0.000000000000000000, -1.000000000000000000 ) ) ;
#2814=CYLINDRICAL_SURFACE ( 'NONE', #17181, 5.500000000000000000 ) ;
#2820=CARTESIAN_POINT ( 'NONE',  ( 142.7961002691896510, 2.071067811865468400, -4.999999999999989342 ) ) ;
#2821=CARTESIAN_POINT ( 'NONE',  ( 145.5863248654052313, 0.000000000000000000, 5.500000000000005329 ) ) ;
#2822=CARTESIAN_POINT ( 'NONE',  ( 152.6250000000000284, 0.000000000000000000, -6.000000000000005329 ) ) ;
#2825=FACE_OUTER_BOUND ( 'NONE', #21627, .T. ) ;
#2827=ORIENTED_EDGE ( 'NONE', *, *, #24879, .T. ) ;
#2828=CARTESIAN_POINT ( 'NONE',  ( 152.8125000000000568, 4.242640687119298093, -4.242640687119298093 ) ) ;
#2832=( BOUNDED_CURVE ( )  B_SPLINE_CURVE ( 2, ( #29045, #10190, #15431, #24758, #14950, #3698, #27199, #24292, #3238 ),
 .UNSPECIFIED., .F., .F. ) 
 B_SPLINE_CURVE_WITH_KNOTS ( ( 3, 2, 2, 2, 3 ),
 ( 0.8875000000000003997, 0.8937500000000002665, 0.9000000000000000222, 0.9062499999999997780, 0.9124999999999995337 ),
 .UNSPECIFIED. ) 
 CURVE ( )  GEOMETRIC_REPRESENTATION_ITEM ( )  RATIONAL_B_SPLINE_CURVE ( ( 0.9999999999999945599, 0.9238795325112921786, 1.000000000000000000, 0.9238795325112867385, 1.000000000000000000, 0.9238795325112867385, 1.000000000000000000, 0.9238795325112921786, 0.9999999999999945599 ) ) 
 REPRESENTATION_ITEM ( '' )  );
#2835=ORIENTED_EDGE ( 'NONE', *, *, #12855, .F. ) ;
#2838=ORIENTED_EDGE ( 'NONE', *, *, #5555, .T. ) ;
#2842=CARTESIAN_POINT ( 'NONE',  ( 124.9999999999999432, -70.00000000000000000, 8.000000000000007105 ) ) ;
#2844=CARTESIAN_POINT ( 'NONE',  ( 135.0000273856245201, -6.966962943922541562, 8.502862253531825232 ) ) ;
#2851=CARTESIAN_POINT ( 'NONE',  ( 148.5863248654052313, 0.000000000000000000, 5.500000000000005329 ) ) ;
#2852=ADVANCED_FACE ( 'NONE', ( #27188 ), #29181, .F. ) ;
#2854=CARTESIAN_POINT ( 'NONE',  ( 144.9449251345948255, -5.500000000000012434, 2.278174593052012309 ) ) ;
#2864=CARTESIAN_POINT ( 'NONE',  ( -0.08385222888512024186, -15.14261269756462269, -7.883965026287834910 ) ) ;
#2866=ORIENTED_EDGE ( 'NONE', *, *, #14291, .T. ) ;
#2867=CARTESIAN_POINT ( 'NONE',  ( 145.9687500000000568, -2.485281374238585972, 6.000000000000005329 ) ) ;
#2868=ORIENTED_EDGE ( 'NONE', *, *, #14613, .T. ) ;
#2874=ORIENTED_EDGE ( 'NONE', *, *, #20069, .F. ) ;
#2878=CARTESIAN_POINT ( 'NONE',  ( 133.0163997308104058, 4.999999999999989342, 2.071067811865468400 ) ) ;
#2883=DIRECTION ( 'NONE',  ( 0.000000000000000000, 0.000000000000000000, -1.000000000000000000 ) ) ;
#2888=PLANE ( 'NONE',  #25881 ) ;
#2894=CARTESIAN_POINT ( 'NONE',  ( 148.6949251345948539, 5.500000000000012434, -2.278174593052012309 ) ) ;
#2895=VERTEX_POINT ( 'NONE', #9506 ) ;
#2903=EDGE_LOOP ( 'NONE', ( #27728, #28703, #9986, #25114 ) ) ;
#2908=CARTESIAN_POINT ( 'NONE',  ( 135.2961002691896226, 2.071067811865468400, -4.999999999999989342 ) ) ;
#2914=ORIENTED_EDGE ( 'NONE', *, *, #22757, .F. ) ;
#2916=DIRECTION ( 'NONE',  ( 1.000000000000000000, 0.000000000000000000, -0.000000000000000000 ) ) ;
#2917=DIRECTION ( 'NONE',  ( -0.000000000000000000, -0.000000000000000000, -1.000000000000000000 ) ) ;
#2919=CARTESIAN_POINT ( 'NONE',  ( 138.8288997308104058, 4.999999999999989342, -2.071067811865468400 ) ) ;
#2920=CARTESIAN_POINT ( 'NONE',  ( 137.9925748654052029, 2.278174593052074925, 5.499999999999950262 ) ) ;
#2926=TOROIDAL_SURFACE ( 'NONE', #6853, 10.49999999999998934, 0.5000000000000000000 ) ;
#2928=CARTESIAN_POINT ( 'NONE',  ( 1.000000000000000888, -14.99923475244191451, -9.015151515151503148 ) ) ;
#2931=DIRECTION ( 'NONE',  ( 1.000000000000000000, 0.000000000000000000, 0.000000000000000000 ) ) ;
#2941=CYLINDRICAL_SURFACE ( 'NONE', #14986, 1.000000000000000000 ) ;
#2942=AXIS2_PLACEMENT_3D ( 'NONE', #11189, #17802, #25263 ) ;
#2944=ORIENTED_EDGE ( 'NONE', *, *, #3388, .T. ) ;
#2945=EDGE_LOOP ( 'NONE', ( #7663, #23528, #21633, #126 ) ) ;
#2946=CIRCLE ( 'NONE', #28920, 15.00000000000000000 ) ;
#2949=DIRECTION ( 'NONE',  ( 1.000000000000000000, 0.000000000000000000, -0.000000000000000000 ) ) ;
#2950=CARTESIAN_POINT ( 'NONE',  ( 159.5344527694593921, -12.11656139239292784, -3.856021467126169000 ) ) ;
#2954=DIRECTION ( 'NONE',  ( -1.000000000000000000, -0.000000000000000000, -0.000000000000000000 ) ) ;
#2955=FILL_AREA_STYLE_COLOUR ( '', #25889 ) ;
#2960=CARTESIAN_POINT ( 'NONE',  ( 140.4999999888488276, -9.513811511959360701, 7.314917984054192246 ) ) ;
#2965=CARTESIAN_POINT ( 'NONE',  ( 146.9211002691896510, -4.999999999999989342, -2.071067811865468400 ) ) ;
#2966=CARTESIAN_POINT ( 'NONE',  ( 152.4375000000000284, -4.242640687119298093, -4.242640687119298093 ) ) ;
#2967=CARTESIAN_POINT ( 'NONE',  ( 135.0000000000000284, -9.047800747817580813, -7.500000000000007105 ) ) ;
#2970=CARTESIAN_POINT ( 'NONE',  ( 135.0000000000000284, -12.00000000000001066, -5.000000000000004441 ) ) ;
#2972=EDGE_LOOP ( 'NONE', ( #19771, #1972, #9379, #9654 ) ) ;
#2973=CARTESIAN_POINT ( 'NONE',  ( 153.0000000000000284, 6.000000000000005329, 0.000000000000000000 ) ) ;
#2975=UNCERTAINTY_MEASURE_WITH_UNIT (LENGTH_MEASURE( 1.000000000000000082E-05 ), #20026, 'distance_accuracy_value', 'NONE');
#2976=LINE ( 'NONE', #24318, #19245 ) ;
#2980=ORIENTED_EDGE ( 'NONE', *, *, #18472, .T. ) ;
#2982=AXIS2_PLACEMENT_3D ( 'NONE', #23278, #9278, #2507 ) ;
#2984=VERTEX_POINT ( 'NONE', #8221 ) ;
#2985=CIRCLE ( 'NONE', #3972, 1.000000000000000000 ) ;
#2988=CARTESIAN_POINT ( 'NONE',  ( 125.0000000000000568, -55.00000000000000711, -5.000000000000004441 ) ) ;
#2995=CARTESIAN_POINT ( 'NONE',  ( 135.0000000000000284, 5.526307313663695098, 1.967927276880694576 ) ) ;
#3000=CARTESIAN_POINT ( 'NONE',  ( 116.0000000000000142, 6.735557395310442023E-16, 5.500000000000000000 ) ) ;
#3004=FACE_OUTER_BOUND ( 'NONE', #20337, .T. ) ;
#3005=AXIS2_PLACEMENT_3D ( 'NONE', #9363, #2450, #4128 ) ;
#3010=CARTESIAN_POINT ( 'NONE',  ( -0.07568246969667169477, -14.85893693147072447, -8.149031565298297863 ) ) ;
#3016=EDGE_CURVE ( 'NONE', #7376, #4225, #13199, .T. ) ;
#3021=ORIENTED_EDGE ( 'NONE', *, *, #28436, .F. ) ;
#3024=CARTESIAN_POINT ( 'NONE',  ( 135.0000000000000284, -7.065583442230452427, 8.449385501354864658 ) ) ;
#3025=CARTESIAN_POINT ( 'NONE',  ( 134.4226497308104058, 5.000000000000004441, 0.000000000000000000 ) ) ;
#3026=CIRCLE ( 'NONE', #21218, 0.4999999999999993894 ) ;
#3028=ORIENTED_EDGE ( 'NONE', *, *, #8081, .F. ) ;
#3037=CARTESIAN_POINT ( 'NONE',  ( 155.1636751345948255, 0.000000000000000000, 5.500000000000005329 ) ) ;
#3042=CARTESIAN_POINT ( 'NONE',  ( -9.999999999999793943, 9.000000000000007105, 3.000000000000002665 ) ) ;
#3047=CARTESIAN_POINT ( 'NONE',  ( -4.999999999999990230, -24.99999999999999289, -8.000000000000007105 ) ) ;
#3049=CARTESIAN_POINT ( 'NONE',  ( -20.99999999999998224, -54.99999999999990763, 5.000000000000004441 ) ) ;
#3056=CARTESIAN_POINT ( 'NONE',  ( 133.7023502691896510, 0.000000000000000000, -5.000000000000004441 ) ) ;
#3069=CARTESIAN_POINT ( 'NONE',  ( 136.6726497308104058, -5.000000000000004441, 0.000000000000000000 ) ) ;
#3079=CARTESIAN_POINT ( 'NONE',  ( 161.0000000000000284, 1.469576158976823947E-15, 12.00000000000000178 ) ) ;
#3089=VECTOR ( 'NONE', #4789, 1000.000000000000000 ) ;
#3090=VERTEX_POINT ( 'NONE', #13649 ) ;
#3091=VECTOR ( 'NONE', #14746, 1000.000000000000000 ) ;
#3099=DIRECTION ( 'NONE',  ( 1.000000000000000000, 0.000000000000000000, 0.000000000000000000 ) ) ;
#3101=LINE ( 'NONE', #12674, #16794 ) ;
#3104=CARTESIAN_POINT ( 'NONE',  ( 140.0546052829554071, -9.478432856838029608, 7.360605440459326410 ) ) ;
#3106=CARTESIAN_POINT ( 'NONE',  ( 140.0699251345947971, 2.278174593052322283, 5.499999999999701572 ) ) ;
#3107=CARTESIAN_POINT ( 'NONE',  ( 146.8050748654052313, 5.500000000000012434, 2.278174593052012309 ) ) ;
#3113=CARTESIAN_POINT ( 'NONE',  ( 141.6711002691896795, 4.999999999999989342, 2.071067811865468400 ) ) ;
#3115=CARTESIAN_POINT ( 'NONE',  ( 150.2812500000000284, 2.485281374238585972, 6.000000000000005329 ) ) ;
#3116=DIRECTION ( 'NONE',  ( 1.387778780781521564E-14, -1.000000000000000000, 0.000000000000000000 ) ) ;
#3122=CARTESIAN_POINT ( 'NONE',  ( 142.0312500000000284, -2.485281374238555774, -6.000000000000005329 ) ) ;
#3133=FACE_OUTER_BOUND ( 'NONE', #17440, .T. ) ;
#3135=LINE ( 'NONE', #19887, #4881 ) ;
#3136=FACE_OUTER_BOUND ( 'NONE', #1711, .T. ) ;
#3138=CARTESIAN_POINT ( 'NONE',  ( 160.9761751345948255, 3.889087296526011706, 3.889087296526011706 ) ) ;
#3140=FACE_OUTER_BOUND ( 'NONE', #8232, .T. ) ;
#3141=CARTESIAN_POINT ( 'NONE',  ( 148.9613248654052029, -5.500000000000005329, 0.000000000000000000 ) ) ;
#3143=FILL_AREA_STYLE ('',( #12718 ) ) ;
#3149=FILL_AREA_STYLE ('',( #714 ) ) ;
#3150=CARTESIAN_POINT ( 'NONE',  ( 161.0086076262249151, 3.226123241052607060, 4.476387269555026194 ) ) ;
#3152=CARTESIAN_POINT ( 'NONE',  ( 160.5000000000000284, 6.000000000000005329, 0.000000000000000000 ) ) ;
#3153=DIRECTION ( 'NONE',  ( 1.000000000000000000, -0.000000000000000000, -0.000000000000000000 ) ) ;
#3154=CARTESIAN_POINT ( 'NONE',  ( 124.9999999999999432, -71.00000000000001421, -4.000000000000003553 ) ) ;
#3158=EDGE_CURVE ( 'NONE', #28288, #22958, #20397, .T. ) ;
#3159=CARTESIAN_POINT ( 'NONE',  ( 146.6250000000000284, 0.000000000000000000, -6.000000000000005329 ) ) ;
#3168=CIRCLE ( 'NONE', #23811, 0.5000000000000004441 ) ;
#3169=CIRCLE ( 'NONE', #22826, 14.99999999999998579 ) ;
#3175=PLANE ( 'NONE',  #26084 ) ;
#3180=DIRECTION ( 'NONE',  ( 0.000000000000000000, 0.9165151389911677660, 0.4000000000000004663 ) ) ;
#3184=( BOUNDED_CURVE ( )  B_SPLINE_CURVE ( 3, ( #22646, #15768, #18359, #29685 ),
 .UNSPECIFIED., .F., .T. ) 
 B_SPLINE_CURVE_WITH_KNOTS ( ( 4, 4 ),
 ( 3.536383773289572652, 4.712388980384689674 ),
 .UNSPECIFIED. ) 
 CURVE ( )  GEOMETRIC_REPRESENTATION_ITEM ( )  RATIONAL_B_SPLINE_CURVE ( ( 1.000000000000000000, 0.8880335295585657374, 0.8880335295585657374, 1.000000000000000000 ) ) 
 REPRESENTATION_ITEM ( '' )  );
#3185=CARTESIAN_POINT ( 'NONE',  ( 148.4136751345948539, 0.000000000000000000, -5.500000000000005329 ) ) ;
#3187=ADVANCED_FACE ( 'NONE', ( #11500 ), #25375, .F. ) ;
#3189=DIRECTION ( 'NONE',  ( -0.000000000000000000, -0.000000000000000000, -1.000000000000000000 ) ) ;
#3190=ORIENTED_EDGE ( 'NONE', *, *, #845, .F. ) ;
#3193=SURFACE_STYLE_USAGE ( .BOTH. , #26685 ) ;
#3197=CARTESIAN_POINT ( 'NONE',  ( 133.2336002691896510, -4.999999999999989342, 2.071067811865468400 ) ) ;
#3203=VERTEX_POINT ( 'NONE', #16852 ) ;
#3207=CARTESIAN_POINT ( 'NONE',  ( 138.4538997308104342, -2.071067811865468400, -4.999999999999989342 ) ) ;
#3210=AXIS2_PLACEMENT_3D ( 'NONE', #10135, #7366, #19504 ) ;
#3211=PRESENTATION_STYLE_ASSIGNMENT (( #26419 ) ) ;
#3216=VERTEX_POINT ( 'NONE', #15100 ) ;
#3218=EDGE_CURVE ( 'NONE', #21999, #14866, #18853, .T. ) ;
#3224=CARTESIAN_POINT ( 'NONE',  ( 135.8437500000000284, -6.000000000000005329, -2.485281374238556218 ) ) ;
#3232=CARTESIAN_POINT ( 'NONE',  ( 140.2643372958527266, -11.26433729585132681, 4.292342582647273197 ) ) ;
#3235=ORIENTED_EDGE ( 'NONE', *, *, #23025, .T. ) ;
#3236=CARTESIAN_POINT ( 'NONE',  ( 160.9860723913248819, -11.61453176910477048, 3.019692173012635372 ) ) ;
#3238=CARTESIAN_POINT ( 'NONE',  ( 159.6636751345948539, 0.000000000000000000, 5.500000000000005329 ) ) ;
#3239=CARTESIAN_POINT ( 'NONE',  ( -1.000000000000000888, -9.000000000000007105, 4.000000000000003553 ) ) ;
#3242=CARTESIAN_POINT ( 'NONE',  ( 157.0163997308104058, 4.999999999999989342, 2.071067811865468400 ) ) ;
#3244=CIRCLE ( 'NONE', #28275, 0.5000000000000004441 ) ;
#3246=DIRECTION ( 'NONE',  ( 0.000000000000000000, 0.000000000000000000, -1.000000000000000000 ) ) ;
#3248=CARTESIAN_POINT ( 'NONE',  ( -1.000000000000000888, 9.000000000000007105, 4.000000000000003553 ) ) ;
#3250=CARTESIAN_POINT ( 'NONE',  ( 139.4136751345948539, 0.000000000000000000, -5.500000000000005329 ) ) ;
#3252=ADVANCED_FACE ( 'NONE', ( #2678 ), #9467, .F. ) ;
#3255=DIRECTION ( 'NONE',  ( -0.000000000000000000, -0.000000000000000000, -1.000000000000000000 ) ) ;
#3257=CARTESIAN_POINT ( 'NONE',  ( 137.0773502691896510, 5.000000000000004441, 0.000000000000000000 ) ) ;
#3258=CARTESIAN_POINT ( 'NONE',  ( 154.4062500000000284, 6.000000000000005329, -2.485281374238556218 ) ) ;
#3259=CARTESIAN_POINT ( 'NONE',  ( 139.5000000000000000, -8.944271909999162773, 8.000000000000007105 ) ) ;
#3263=ADVANCED_FACE ( 'NONE', ( #19005 ), #28532, .F. ) ;
#3267=CARTESIAN_POINT ( 'NONE',  ( 141.4687500000000568, -2.485281374238585972, 6.000000000000005329 ) ) ;
#3268=CARTESIAN_POINT ( 'NONE',  ( 142.8675748654052029, -5.500000000000012434, 2.278174593052012309 ) ) ;
#3269=AXIS2_PLACEMENT_3D ( 'NONE', #15492, #15339, #29254 ) ;
#3272=CIRCLE ( 'NONE', #4254, 14.49999999999999822 ) ;
#3282=CARTESIAN_POINT ( 'NONE',  ( 0.000000000000000000, 9.000000000000007105, -3.000000000000002665 ) ) ;
#3283=CARTESIAN_POINT ( 'NONE',  ( 135.2991173618607945, -8.337648098118274120, 8.244751738007437325 ) ) ;
#3284=TOROIDAL_SURFACE ( 'NONE', #1346, 16.50000000000000355, 1.000000000000000000 ) ;
#3291=CARTESIAN_POINT ( 'NONE',  ( 142.5863248654052313, 0.000000000000000000, 5.500000000000005329 ) ) ;
#3292=DIRECTION ( 'NONE',  ( 0.000000000000000000, -1.000000000000000000, 0.000000000000000000 ) ) ;
#3295=CARTESIAN_POINT ( 'NONE',  ( 151.7961002691896226, 2.071067811865468400, -4.999999999999989342 ) ) ;
#3297=CARTESIAN_POINT ( 'NONE',  ( 139.8600870026756695, -9.432236288125531942, -7.851756037878587335 ) ) ;
#3307=CIRCLE ( 'NONE', #1860, 1.000000000000000000 ) ;
#3309=CARTESIAN_POINT ( 'NONE',  ( 146.1562500000000853, -6.000000000000005329, 2.485281374238555774 ) ) ;
#3312=ORIENTED_EDGE ( 'NONE', *, *, #1974, .T. ) ;
#3316=( GEOMETRIC_REPRESENTATION_CONTEXT ( 3 ) GLOBAL_UNCERTAINTY_ASSIGNED_CONTEXT ( ( #22359 ) ) GLOBAL_UNIT_ASSIGNED_CONTEXT ( ( #2079, #8842, #16250 ) ) REPRESENTATION_CONTEXT ( 'NONE', 'WORKASPACE' ) );
#3318=VERTEX_POINT ( 'NONE', #15367 ) ;
#3325=CARTESIAN_POINT ( 'NONE',  ( 152.4300748654052029, 2.278174593051795149, -5.500000000000228262 ) ) ;
#3327=CARTESIAN_POINT ( 'NONE',  ( -0.3085845443849983827, -9.691415455615135954, 4.244941038143176470 ) ) ;
#3331=SURFACE_STYLE_USAGE ( .BOTH. , #28983 ) ;
#3334=CARTESIAN_POINT ( 'NONE',  ( 15.00000000000000000, 0.000000000000000000, 0.000000000000000000 ) ) ;
#3335=EDGE_LOOP ( 'NONE', ( #12325, #19985, #15303, #21526 ) ) ;
#3338=CARTESIAN_POINT ( 'NONE',  ( 135.0338636289978069, -7.698222997088485009, -8.313259093246843534 ) ) ;
#3345=ORIENTED_EDGE ( 'NONE', *, *, #2521, .F. ) ;
#3346=CARTESIAN_POINT ( 'NONE',  ( 133.4211002691896510, -4.999999999999989342, -2.071067811865468400 ) ) ;
#3348=VERTEX_POINT ( 'NONE', #24532 ) ;
#3352=ORIENTED_EDGE ( 'NONE', *, *, #29806, .T. ) ;
#3354=CARTESIAN_POINT ( 'NONE',  ( 149.2574251345948255, -2.278174593051764951, 5.500000000000262013 ) ) ;
#3357=CARTESIAN_POINT ( 'NONE',  ( 134.7038997308104058, 2.071067811865468400, 4.999999999999989342 ) ) ;
#3363=DIRECTION ( 'NONE',  ( 0.000000000000000000, 0.3428396514843867759, 0.9393939393939395588 ) ) ;
#3365=EDGE_CURVE ( 'NONE', #28361, #18697, #7651, .T. ) ;
#3370=VECTOR ( 'NONE', #29514, 1000.000000000000000 ) ;
#3372=FACE_OUTER_BOUND ( 'NONE', #8859, .T. ) ;
#3373=FACE_OUTER_BOUND ( 'NONE', #12431, .T. ) ;
#3375=COLOUR_RGB ( '', 0.40784314, 0.44705882, 0.49803922) ;
#3378=DIRECTION ( 'NONE',  ( 1.000000000000000000, -0.000000000000000000, -0.000000000000000000 ) ) ;
#3382=CARTESIAN_POINT ( 'NONE',  ( -9.999999999999772626, -90.00000000000001421, 3.000000000000002665 ) ) ;
#3384=SURFACE_STYLE_FILL_AREA ( #8005 ) ;
#3385=FACE_OUTER_BOUND ( 'NONE', #7622, .T. ) ;
#3388=EDGE_CURVE ( 'NONE', #15417, #2367, #12871, .T. ) ;
#3391=DIRECTION ( 'NONE',  ( 0.000000000000000000, 0.000000000000000000, 1.000000000000000000 ) ) ;
#3395=CARTESIAN_POINT ( 'NONE',  ( 155.6101497308104058, 3.535533905932725318, 3.535533905932725318 ) ) ;
#3402=EDGE_CURVE ( 'NONE', #17791, #9387, #22101, .T. ) ;
#3409=DIRECTION ( 'NONE',  ( -1.000000000000000000, -0.000000000000000000, -0.000000000000000000 ) ) ;
#3410=VERTEX_POINT ( 'NONE', #3633 ) ;
#3411=CARTESIAN_POINT ( 'NONE',  ( 153.3750000000000284, 0.000000000000000000, 6.000000000000005329 ) ) ;
#3415=CARTESIAN_POINT ( 'NONE',  ( 143.7187500000000284, 2.485281374238555774, -6.000000000000005329 ) ) ;
#3416=CARTESIAN_POINT ( 'NONE',  ( 161.4448303879796640, -4.634055226201747146, -3.737401695183885764 ) ) ;
#3417=ORIENTED_EDGE ( 'NONE', *, *, #3601, .F. ) ;
#3420=ORIENTED_EDGE ( 'NONE', *, *, #25051, .F. ) ;
#3422=ADVANCED_FACE ( 'NONE', ( #22249 ), #1340, .F. ) ;
#3426=DIRECTION ( 'NONE',  ( -1.387778780781444256E-14, 1.000000000000000000, 0.000000000000000000 ) ) ;
#3427=TOROIDAL_SURFACE ( 'NONE', #20160, 11.00000000000000355, 1.000000000000000000 ) ;
#3429=CARTESIAN_POINT ( 'NONE',  ( 134.9304254777565291, -7.819842479447205896, 8.000000000000008882 ) ) ;
#3435=CARTESIAN_POINT ( 'NONE',  ( -9.999999999999980460, -60.00000000000001421, -3.000000000000002665 ) ) ;
#3438=( BOUNDED_CURVE ( )  B_SPLINE_CURVE ( 2, ( #17647, #24976, #13214, #15187, #20087, #26969, #22551, #1484, #20247 ),
 .UNSPECIFIED., .F., .T. ) 
 B_SPLINE_CURVE_WITH_KNOTS ( ( 3, 2, 2, 2, 3 ),
 ( 0.4624999999999990230, 0.4687499999999992228, 0.4749999999999994782, 0.4812499999999997335, 0.4875000000000000444 ),
 .UNSPECIFIED. ) 
 CURVE ( )  GEOMETRIC_REPRESENTATION_ITEM ( )  RATIONAL_B_SPLINE_CURVE ( ( 1.000000000000012212, 0.9238795325112745260, 1.000000000000000000, 0.9238795325112867385, 1.000000000000000000, 0.9238795325112867385, 1.000000000000000000, 0.9238795325112867385, 1.000000000000000000 ) ) 
 REPRESENTATION_ITEM ( '' )  );
#3439=CARTESIAN_POINT ( 'NONE',  ( 151.4211002691896510, -4.999999999999989342, -2.071067811865468400 ) ) ;
#3441=CARTESIAN_POINT ( 'NONE',  ( 151.6011751345948539, 3.889087296526011706, -3.889087296526011706 ) ) ;
#3444=CARTESIAN_POINT ( 'NONE',  ( -15.49999999999999289, -24.99999999999999289, -8.000000000000007105 ) ) ;
#3446=ORIENTED_EDGE ( 'NONE', *, *, #15487, .F. ) ;
#3447=CARTESIAN_POINT ( 'NONE',  ( 161.4375000000000284, -4.242640687119298093, -4.242640687119298093 ) ) ;
#3451=VECTOR ( 'NONE', #18949, 1000.000000000000000 ) ;
#3453=ORIENTED_EDGE ( 'NONE', *, *, #11147, .F. ) ;
#3454=CIRCLE ( 'NONE', #26044, 0.5000000000000004441 ) ;
#3456=EDGE_CURVE ( 'NONE', #19810, #28850, #30213, .T. ) ;
#3463=COLOUR_RGB ( '', 0.08235294, 0.09019608, 0.10196078) ;
#3465=ORIENTED_EDGE ( 'NONE', *, *, #24886, .F. ) ;
#3467=EDGE_CURVE ( 'NONE', #14042, #25961, #5469, .T. ) ;
#3475=CARTESIAN_POINT ( 'NONE',  ( -0.8691260360719469391, -9.261747927856070817, 4.026027341348647148 ) ) ;
#3481=DIRECTION ( 'NONE',  ( 0.000000000000000000, 0.000000000000000000, -1.000000000000000000 ) ) ;
#3483=( BOUNDED_CURVE ( )  B_SPLINE_CURVE ( 3, ( #21384, #28412, #26121, #5068 ),
 .UNSPECIFIED., .F., .T. ) 
 B_SPLINE_CURVE_WITH_KNOTS ( ( 4, 4 ),
 ( 0.000000000000000000, 1.570796326794896558 ),
 .UNSPECIFIED. ) 
 CURVE ( )  GEOMETRIC_REPRESENTATION_ITEM ( )  RATIONAL_B_SPLINE_CURVE ( ( 1.000000000000000000, 0.8047378541243649375, 0.8047378541243649375, 1.000000000000000000 ) ) 
 REPRESENTATION_ITEM ( '' )  );
#3484=AXIS2_PLACEMENT_3D ( 'NONE', #11118, #20467, #29825 ) ;
#3487=AXIS2_PLACEMENT_3D ( 'NONE', #15111, #807, #7862 ) ;
#3494=CARTESIAN_POINT ( 'NONE',  ( 138.9300748654052029, 2.278174593051671692, -5.500000000000352607 ) ) ;
#3500=CARTESIAN_POINT ( 'NONE',  ( 156.7500000000000284, -6.000000000000005329, 0.000000000000000000 ) ) ;
#3504=EDGE_LOOP ( 'NONE', ( #1431, #26587, #1475, #1499 ) ) ;
#3505=CARTESIAN_POINT ( 'NONE',  ( 157.3988248654052313, 3.889087296526011706, 3.889087296526011706 ) ) ;
#3507=DIRECTION ( 'NONE',  ( -1.000000000000000000, 0.000000000000000000, 0.000000000000000000 ) ) ;
#3515=DIRECTION ( 'NONE',  ( 1.000000000000000000, 0.000000000000000000, 0.000000000000000000 ) ) ;
#3517=FACE_OUTER_BOUND ( 'NONE', #612, .T. ) ;
#3519=CARTESIAN_POINT ( 'NONE',  ( 135.0000000000000568, 3.752929936578043080, 4.235410701944677392 ) ) ;
#3520=LINE ( 'NONE', #17699, #16113 ) ;
#3526=CARTESIAN_POINT ( 'NONE',  ( -0.5000000000000004441, -10.50000000000000888, 8.500000000000007105 ) ) ;
#3527=FACE_OUTER_BOUND ( 'NONE', #11967, .T. ) ;
#3533=CARTESIAN_POINT ( 'NONE',  ( 135.0000000000001705, 4.957041246451966643, -2.976925002759783112 ) ) ;
#3534=( BOUNDED_CURVE ( )  B_SPLINE_CURVE ( 2, ( #12874, #3759, #3441, #5904, #10868, #17324, #17469, #13029, #26783 ),
 .UNSPECIFIED., .F., .T. ) 
 B_SPLINE_CURVE_WITH_KNOTS ( ( 3, 2, 2, 2, 3 ),
 ( 0.6375000000000001776, 0.6437500000000000444, 0.6499999999999996891, 0.6562499999999994449, 0.6624999999999992006 ),
 .UNSPECIFIED. ) 
 CURVE ( )  GEOMETRIC_REPRESENTATION_ITEM ( )  RATIONAL_B_SPLINE_CURVE ( ( 0.9999999999999973355, 0.9238795325112894030, 1.000000000000000000, 0.9238795325112867385, 1.000000000000000000, 0.9238795325112867385, 1.000000000000000000, 0.9238795325112961754, 0.9999999999999905631 ) ) 
 REPRESENTATION_ITEM ( '' )  );
#3537=CARTESIAN_POINT ( 'NONE',  ( 140.6083823193137334, -11.80419115965730015, 4.059228028636210794 ) ) ;
#3538=EDGE_CURVE ( 'NONE', #1389, #8961, #29474, .T. ) ;
#3549=CARTESIAN_POINT ( 'NONE',  ( 152.1413997308104058, 2.071067811865468400, -4.999999999999989342 ) ) ;
#3556=DIRECTION ( 'NONE',  ( -0.000000000000000000, 0.000000000000000000, 1.000000000000000000 ) ) ;
#3560=DIRECTION ( 'NONE',  ( 0.000000000000000000, 0.000000000000000000, -1.000000000000000000 ) ) ;
#3563=CARTESIAN_POINT ( 'NONE',  ( 145.2187500000000000, 2.485281374238556218, -6.000000000000005329 ) ) ;
#3568=CIRCLE ( 'NONE', #19288, 10.49999999999998224 ) ;
#3570=CARTESIAN_POINT ( 'NONE',  ( 144.8437500000000000, -6.000000000000005329, -2.485281374238555774 ) ) ;
#3574=EDGE_CURVE ( 'NONE', #27416, #13233, #10395, .T. ) ;
#3582=VERTEX_POINT ( 'NONE', #21765 ) ;
#3590=CARTESIAN_POINT ( 'NONE',  ( 156.3675748654052029, -5.500000000000012434, 2.278174593052012309 ) ) ;
#3598=CARTESIAN_POINT ( 'NONE',  ( 154.3273502691896510, -5.000000000000004441, 0.000000000000000000 ) ) ;
#3599=CARTESIAN_POINT ( 'NONE',  ( 140.0000000000000284, -10.00000000000000888, -7.500000000000007105 ) ) ;
#3601=EDGE_CURVE ( 'NONE', #23494, #15347, #11417, .T. ) ;
#3602=CARTESIAN_POINT ( 'NONE',  ( 124.9999999999999432, -69.50000000000000000, 8.000000000000007105 ) ) ;
#3605=ORIENTED_EDGE ( 'NONE', *, *, #27533, .T. ) ;
#3609=VERTEX_POINT ( 'NONE', #27546 ) ;
#3611=ORIENTED_EDGE ( 'NONE', *, *, #9332, .F. ) ;
#3616=CYLINDRICAL_SURFACE ( 'NONE', #8803, 0.5000000000000004441 ) ;
#3617=CARTESIAN_POINT ( 'NONE',  ( 135.0000000000000284, -8.850103465153400961, 7.500000000000122569 ) ) ;
#3619=ORIENTED_EDGE ( 'NONE', *, *, #29167, .T. ) ;
#3620=CARTESIAN_POINT ( 'NONE',  ( -19.99999999999998224, -25.00000000000010658, 8.000000000000007105 ) ) ;
#3622=( BOUNDED_CURVE ( )  B_SPLINE_CURVE ( 2, ( #986, #17774, #1450, #27094, #15475, #24799, #14993, #8680, #3747 ),
 .UNSPECIFIED., .F., .T. ) 
 B_SPLINE_CURVE_WITH_KNOTS ( ( 3, 2, 2, 2, 3 ),
 ( 0.8125000000000013323, 0.8187500000000010880, 0.8250000000000007327, 0.8312500000000004885, 0.8375000000000002442 ),
 .UNSPECIFIED. ) 
 CURVE ( )  GEOMETRIC_REPRESENTATION_ITEM ( )  RATIONAL_B_SPLINE_CURVE ( ( 0.9999999999999837907, 0.9238795325113029477, 1.000000000000000000, 0.9238795325112867385, 1.000000000000000000, 0.9238795325112867385, 1.000000000000000000, 0.9238795325112840739, 1.000000000000002665 ) ) 
 REPRESENTATION_ITEM ( '' )  );
#3633=CARTESIAN_POINT ( 'NONE',  ( 158.3363248654052313, 0.000000000000000000, -5.500000000000005329 ) ) ;
#3634=FILL_AREA_STYLE_COLOUR ( '', #19445 ) ;
#3639=EDGE_CURVE ( 'NONE', #17215, #25878, #22525, .T. ) ;
#3647=ORIENTED_EDGE ( 'NONE', *, *, #13236, .F. ) ;
#3651=VERTEX_POINT ( 'NONE', #25101 ) ;
#3652=CARTESIAN_POINT ( 'NONE',  ( 154.6875000000000284, 4.242640687119269671, 4.242640687119298093 ) ) ;
#3655=VERTEX_POINT ( 'NONE', #13026 ) ;
#3665=DIRECTION ( 'NONE',  ( -0.000000000000000000, -0.000000000000000000, -1.000000000000000000 ) ) ;
#3672=CARTESIAN_POINT ( 'NONE',  ( -10.00000000000000178, -12.00000000000001066, -4.000000000000003553 ) ) ;
#3686=B_SPLINE_CURVE_WITH_KNOTS ( 'NONE', 3,
 ( #8124, #10617, #8446, #17692, #27018, #5983, #15867, #29933 ),
 .UNSPECIFIED., .F., .F.,
 ( 4, 2, 2, 4 ),
 ( 0.000000000000000000, 0.0001164977210824447509, 0.0002329954421648895019, 0.0004659908843297791122 ),
 .UNSPECIFIED. ) ;
#3689=VECTOR ( 'NONE', #9022, 1000.000000000000000 ) ;
#3693=CARTESIAN_POINT ( 'NONE',  ( 144.5625000000000284, -4.242640687119298093, 4.242640687119298093 ) ) ;
#3695=CARTESIAN_POINT ( 'NONE',  ( 136.0238248654052029, 3.889087296526011706, -3.889087296526011706 ) ) ;
#3696=( GEOMETRIC_REPRESENTATION_CONTEXT ( 3 ) GLOBAL_UNCERTAINTY_ASSIGNED_CONTEXT ( ( #12130 ) ) GLOBAL_UNIT_ASSIGNED_CONTEXT ( ( #678, #370, #19441 ) ) REPRESENTATION_CONTEXT ( 'NONE', 'WORKASPACE' ) );
#3698=CARTESIAN_POINT ( 'NONE',  ( 159.3824251345948255, 5.500000000000012434, 2.278174593052012309 ) ) ;
#3702=CARTESIAN_POINT ( 'NONE',  ( 0.000000000000000000, -10.50000000000000888, -7.500000000000007105 ) ) ;
#3703=CARTESIAN_POINT ( 'NONE',  ( 148.1101497308104058, 3.535533905932725318, 3.535533905932725318 ) ) ;
#3705=FACE_OUTER_BOUND ( 'NONE', #2127, .T. ) ;
#3706=CARTESIAN_POINT ( 'NONE',  ( -9.999999999999765521, -90.00000000000001421, 4.000000000000003553 ) ) ;
#3707=( LENGTH_UNIT ( ) NAMED_UNIT ( * ) SI_UNIT ( .MILLI., .METRE. ) );
#3708=CARTESIAN_POINT ( 'NONE',  ( 135.4710248857196859, -8.959958897678786727, 8.000000000000005329 ) ) ;
#3720=EDGE_CURVE ( 'NONE', #15258, #28330, #8648, .T. ) ;
#3722=ORIENTED_EDGE ( 'NONE', *, *, #18431, .T. ) ;
#3724=CARTESIAN_POINT ( 'NONE',  ( 143.4375000000000284, -4.242640687119298093, -4.242640687119298093 ) ) ;
#3727=ORIENTED_EDGE ( 'NONE', *, *, #2046, .T. ) ;
#3728=CARTESIAN_POINT ( 'NONE',  ( 140.9062500000000568, 6.000000000000005329, -2.485281374238555774 ) ) ;
#3729=CARTESIAN_POINT ( 'NONE',  ( 142.6800748654051745, -2.278174593051950136, 5.500000000000074607 ) ) ;
#3732=ORIENTED_EDGE ( 'NONE', *, *, #18337, .F. ) ;
#3735=AXIS2_PLACEMENT_3D ( 'NONE', #30287, #27961, #6938 ) ;
#3739=CARTESIAN_POINT ( 'NONE',  ( -9.999999999999772626, -90.00000000000001421, -3.000000000000002665 ) ) ;
#3747=CARTESIAN_POINT ( 'NONE',  ( 136.5863248654052313, 0.000000000000000000, 5.500000000000005329 ) ) ;
#3752=CIRCLE ( 'NONE', #16558, 28.99999999999999645 ) ;
#3754=( NAMED_UNIT ( * ) SI_UNIT ( $, .STERADIAN. ) SOLID_ANGLE_UNIT ( ) );
#3757=CARTESIAN_POINT ( 'NONE',  ( 151.3273502691896510, -5.000000000000004441, 0.000000000000000000 ) ) ;
#3758=CARTESIAN_POINT ( 'NONE',  ( 161.0000000000000284, -5.424442335930618420, -0.9085292203135086897 ) ) ;
#3759=CARTESIAN_POINT ( 'NONE',  ( 151.5074251345948255, 2.278174593052074925, -5.499999999999950262 ) ) ;
#3762=CARTESIAN_POINT ( 'NONE',  ( -4.999999999999990230, -55.00000000000002132, -7.500000000000007105 ) ) ;
#3764=ORIENTED_EDGE ( 'NONE', *, *, #11537, .F. ) ;
#3765=FACE_OUTER_BOUND ( 'NONE', #28995, .T. ) ;
#3766=CARTESIAN_POINT ( 'NONE',  ( 135.0000000000000284, -11.07692307692306777, 4.615384615384604317 ) ) ;
#3769=ORIENTED_EDGE ( 'NONE', *, *, #9184, .T. ) ;
#3771=AXIS2_PLACEMENT_3D ( 'NONE', #8592, #8905, #20734 ) ;
#3777=CARTESIAN_POINT ( 'NONE',  ( 139.5000000000000284, -8.798545334315205579, -8.160000000000000142 ) ) ;
#3779=EDGE_CURVE ( 'NONE', #7022, #10874, #16334, .T. ) ;
#3781=ORIENTED_EDGE ( 'NONE', *, *, #28923, .T. ) ;
#3782=DIRECTION ( 'NONE',  ( 0.000000000000000000, 0.000000000000000000, 1.000000000000000000 ) ) ;
#3783=CARTESIAN_POINT ( 'NONE',  ( 125.0000000000000568, -55.00000000000000711, 8.000000000000007105 ) ) ;
#3786=SURFACE_SIDE_STYLE ('',( #22555 ) ) ;
#3787=CARTESIAN_POINT ( 'NONE',  ( -1.000000000000002220, -9.000000000000007105, 4.000000000000005329 ) ) ;
#3790=ADVANCED_FACE ( 'NONE', ( #21276 ), #6982, .F. ) ;
#3792=CARTESIAN_POINT ( 'NONE',  ( 135.0000000000000284, -7.797751917820416878, 7.985411280316564664 ) ) ;
#3796=AXIS2_PLACEMENT_3D ( 'NONE', #26788, #17327, #16885 ) ;
#3799=ORIENTED_EDGE ( 'NONE', *, *, #1359, .F. ) ;
#3800=CARTESIAN_POINT ( 'NONE',  ( 139.2113248654052313, 5.500000000000005329, 0.000000000000000000 ) ) ;
#3805=ORIENTED_EDGE ( 'NONE', *, *, #21805, .F. ) ;
#3806=CARTESIAN_POINT ( 'NONE',  ( 154.4062500000000284, 6.000000000000005329, -2.485281374238555774 ) ) ;
#3810=ORIENTED_EDGE ( 'NONE', *, *, #21573, .F. ) ;
#3811=DIRECTION ( 'NONE',  ( 0.000000000000000000, -1.000000000000000000, 0.000000000000000000 ) ) ;
#3813=PRESENTATION_STYLE_ASSIGNMENT (( #23681 ) ) ;
#3814=VECTOR ( 'NONE', #7793, 1000.000000000000000 ) ;
#3816=( LENGTH_UNIT ( ) NAMED_UNIT ( * ) SI_UNIT ( .MILLI., .METRE. ) );
#3817=ADVANCED_FACE ( 'NONE', ( #19863 ), #19433, .T. ) ;
#3819=CARTESIAN_POINT ( 'NONE',  ( -40.00000000000000000, -20.00000000000021316, -3.000000000000002665 ) ) ;
#3820=LINE ( 'NONE', #6283, #27542 ) ;
#3831=EDGE_CURVE ( 'NONE', #18461, #16010, #3752, .T. ) ;
#3834=ORIENTED_EDGE ( 'NONE', *, *, #9953, .F. ) ;
#3836=CARTESIAN_POINT ( 'NONE',  ( 160.0238248654052313, 3.889087296526011706, -3.889087296526011706 ) ) ;
#3838=CARTESIAN_POINT ( 'NONE',  ( 136.7961002691896510, 2.071067811865468400, -4.999999999999989342 ) ) ;
#3843=ORIENTED_EDGE ( 'NONE', *, *, #22645, .F. ) ;
#3845=CARTESIAN_POINT ( 'NONE',  ( 141.7500000000000568, -6.000000000000005329, 0.000000000000000000 ) ) ;
#3847=PRESENTATION_STYLE_ASSIGNMENT (( #22920 ) ) ;
#3848=FILL_AREA_STYLE ('',( #24901 ) ) ;
#3855=CARTESIAN_POINT ( 'NONE',  ( 147.2663997308104058, -4.999999999999989342, -2.071067811865468400 ) ) ;
#3859=ADVANCED_FACE ( 'NONE', ( #9906 ), #6219, .T. ) ;
#3861=AXIS2_PLACEMENT_3D ( 'NONE', #23367, #7365, #12017 ) ;
#3864=DIRECTION ( 'NONE',  ( 1.000000000000000000, -0.000000000000000000, -0.000000000000000000 ) ) ;
#3865=ORIENTED_EDGE ( 'NONE', *, *, #13519, .T. ) ;
#3868=CARTESIAN_POINT ( 'NONE',  ( 125.0000000000000568, -55.00000000000000711, -8.000000000000007105 ) ) ;
#3872=CARTESIAN_POINT ( 'NONE',  ( 143.2500000000000568, -6.000000000000005329, 0.000000000000000000 ) ) ;
#3875=ORIENTED_EDGE ( 'NONE', *, *, #23559, .T. ) ;
#3876=CARTESIAN_POINT ( 'NONE',  ( 135.6562500000000284, -6.000000000000005329, 2.485281374238555774 ) ) ;
#3878=ORIENTED_EDGE ( 'NONE', *, *, #22677, .F. ) ;
#3883=ADVANCED_FACE ( 'NONE', ( #7874 ), #24455, .T. ) ;
#3887=CARTESIAN_POINT ( 'NONE',  ( 141.0000000000000284, -12.00000000000001066, 4.000000000000003553 ) ) ;
#3888=DIRECTION ( 'NONE',  ( -1.000000000000000000, -1.387778780781444413E-14, 0.000000000000000000 ) ) ;
#3889=CARTESIAN_POINT ( 'NONE',  ( 116.0000000000000142, 0.000000000000000000, -5.500000000000000000 ) ) ;
#3896=VECTOR ( 'NONE', #6096, 1000.000000000000000 ) ;
#3902=CARTESIAN_POINT ( 'NONE',  ( 154.6086002691896510, -2.071067811865468400, -4.999999999999989342 ) ) ;
#3905=CIRCLE ( 'NONE', #22576, 9.999999999999998224 ) ;
#3908=CARTESIAN_POINT ( 'NONE',  ( 150.7425748654052313, -2.278174593052229469, -5.499999999999796607 ) ) ;
#3909=DIRECTION ( 'NONE',  ( 0.000000000000000000, -1.000000000000000000, 0.000000000000000000 ) ) ;
#3911=CARTESIAN_POINT ( 'NONE',  ( 153.9375000000000284, -4.242640687119298093, -4.242640687119298093 ) ) ;
#3914=ORIENTED_EDGE ( 'NONE', *, *, #19067, .T. ) ;
#3926=ORIENTED_EDGE ( 'NONE', *, *, #20453, .T. ) ;
#3927=LINE ( 'NONE', #1637, #3896 ) ;
#3940=MECHANICAL_DESIGN_GEOMETRIC_PRESENTATION_REPRESENTATION('',(#23108),#15786);
#3942=TOROIDAL_SURFACE ( 'NONE', #12833, 10.49999999999998934, 0.5000000000000000000 ) ;
#3943=ORIENTED_EDGE ( 'NONE', *, *, #17363, .F. ) ;
#3948=ADVANCED_FACE ( 'NONE', ( #25068 ), #6190, .T. ) ;
#3951=VERTEX_POINT ( 'NONE', #26903 ) ;
#3953=VECTOR ( 'NONE', #20634, 1000.000000000000000 ) ;
#3955=ORIENTED_EDGE ( 'NONE', *, *, #12405, .T. ) ;
#3956=CARTESIAN_POINT ( 'NONE',  ( 158.9062500000000284, 6.000000000000005329, -2.485281374238555774 ) ) ;
#3960=CARTESIAN_POINT ( 'NONE',  ( 140.0769230769231228, -11.53846153846155254, -4.615384615384604317 ) ) ;
#3964=CARTESIAN_POINT ( 'NONE',  ( 159.3293511854687949, -12.04413325411710467, 3.946525873397269457 ) ) ;
#3969=DIRECTION ( 'NONE',  ( -1.000000000000000000, 0.000000000000000000, 0.000000000000000000 ) ) ;
#3971=CARTESIAN_POINT ( 'NONE',  ( 125.0000000000000568, -55.00000000000000711, 4.000000000000003553 ) ) ;
#3972=AXIS2_PLACEMENT_3D ( 'NONE', #4867, #30377, #16449 ) ;
#3982=DIRECTION ( 'NONE',  ( 0.000000000000000000, 0.000000000000000000, -1.000000000000000000 ) ) ;
#3988=CARTESIAN_POINT ( 'NONE',  ( 137.7336002691896510, -4.999999999999989342, 2.071067811865468400 ) ) ;
#3991=SURFACE_SIDE_STYLE ('',( #15576 ) ) ;
#3996=CARTESIAN_POINT ( 'NONE',  ( 135.0000000000000284, 3.979704198237310919, -4.051284705845048961 ) ) ;
#3998=DIRECTION ( 'NONE',  ( 1.000000000000000000, 0.000000000000000000, 0.000000000000000000 ) ) ;
#4000=CARTESIAN_POINT ( 'NONE',  ( 159.8141916148839812, -12.30834012067592020, 3.594214859449901933 ) ) ;
#4001=CARTESIAN_POINT ( 'NONE',  ( 141.2812500000000284, 2.485281374238585972, 6.000000000000005329 ) ) ;
#4004=VERTEX_POINT ( 'NONE', #2201 ) ;
#4006=CIRCLE ( 'NONE', #12889, 0.5000000000000004441 ) ;
#4010=SURFACE_STYLE_USAGE ( .BOTH. , #2027 ) ;
#4011=CARTESIAN_POINT ( 'NONE',  ( 140.0000000000000284, -10.00000000000000888, 7.500000000000007105 ) ) ;
#4013=CARTESIAN_POINT ( 'NONE',  ( 151.2976497308104058, 0.000000000000000000, 5.000000000000004441 ) ) ;
#4016=DIRECTION ( 'NONE',  ( 0.000000000000000000, -1.000000000000000000, 0.000000000000000000 ) ) ;
#4025=CARTESIAN_POINT ( 'NONE',  ( -19.49999999999998224, -24.99999999999999289, 7.500000000000007105 ) ) ;
#4026=VERTEX_POINT ( 'NONE', #2637 ) ;
#4028=CARTESIAN_POINT ( 'NONE',  ( 147.3750000000000284, 0.000000000000000000, 6.000000000000005329 ) ) ;
#4029=DIRECTION ( 'NONE',  ( 6.938893903907221278E-15, -1.000000000000000000, 0.000000000000000000 ) ) ;
#4030=CIRCLE ( 'NONE', #4989, 0.5000000000000004441 ) ;
#4031=EDGE_CURVE ( 'NONE', #21964, #25175, #11455, .T. ) ;
#4032=ORIENTED_EDGE ( 'NONE', *, *, #28023, .F. ) ;
#4033=CARTESIAN_POINT ( 'NONE',  ( 137.4375000000000568, -4.242640687119298093, -4.242640687119298093 ) ) ;
#4034=PLANE ( 'NONE',  #21496 ) ;
#4036=ORIENTED_EDGE ( 'NONE', *, *, #23880, .F. ) ;
#4037=EDGE_CURVE ( 'NONE', #6912, #8542, #14215, .T. ) ;
#4044=ORIENTED_EDGE ( 'NONE', *, *, #2521, .T. ) ;
#4048=CARTESIAN_POINT ( 'NONE',  ( 140.5000000000000284, 0.000000000000000000, 0.000000000000000000 ) ) ;
#4055=CYLINDRICAL_SURFACE ( 'NONE', #20513, 5.500000000000000000 ) ;
#4058=CARTESIAN_POINT ( 'NONE',  ( 148.7961002691896510, 2.071067811865468400, -4.999999999999989342 ) ) ;
#4063=DIRECTION ( 'NONE',  ( 1.000000000000000000, 1.067522139062651904E-16, -0.000000000000000000 ) ) ;
#4064=EDGE_CURVE ( 'NONE', #11180, #6328, #20956, .T. ) ;
#4066=CARTESIAN_POINT ( 'NONE',  ( 161.0000000000000284, 0.000000000000000000, 0.000000000000000000 ) ) ;
#4070=CARTESIAN_POINT ( 'NONE',  ( 156.8437500000000284, -6.000000000000005329, -2.485281374238555774 ) ) ;
#4075=VERTEX_POINT ( 'NONE', #11916 ) ;
#4082=( GEOMETRIC_REPRESENTATION_CONTEXT ( 3 ) GLOBAL_UNCERTAINTY_ASSIGNED_CONTEXT ( ( #19186 ) ) GLOBAL_UNIT_ASSIGNED_CONTEXT ( ( #18415, #21310, #25438 ) ) REPRESENTATION_CONTEXT ( 'NONE', 'WORKASPACE' ) );
#4083=CARTESIAN_POINT ( 'NONE',  ( 0.7669223171414760731, -15.58766199952932396, 7.954545454545463912 ) ) ;
#4086=DIRECTION ( 'NONE',  ( 0.000000000000000000, 0.000000000000000000, -1.000000000000000000 ) ) ;
#4087=ORIENTED_EDGE ( 'NONE', *, *, #15454, .F. ) ;
#4089=DIRECTION ( 'NONE',  ( -1.000000000000000000, -1.067522139062651904E-16, 0.000000000000000000 ) ) ;
#4098=CARTESIAN_POINT ( 'NONE',  ( 161.0773502691896510, 5.000000000000004441, 0.000000000000000000 ) ) ;
#4100=CARTESIAN_POINT ( 'NONE',  ( -0.08258755314531825154, -15.14553112961706560, 7.837970064863971409 ) ) ;
#4109=CARTESIAN_POINT ( 'NONE',  ( 116.0000000000000142, 0.000000000000000000, -5.500000000000000000 ) ) ;
#4111=DIRECTION ( 'NONE',  ( -0.9230769230769190203, 0.000000000000000000, -0.3846153846153945177 ) ) ;
#4113=CARTESIAN_POINT ( 'NONE',  ( 157.5000000000000284, 6.000000000000005329, 0.000000000000000000 ) ) ;
#4122=CARTESIAN_POINT ( 'NONE',  ( 159.9946976994248757, -11.54806779403923045, 3.290164197027113602 ) ) ;
#4123=( LENGTH_UNIT ( ) NAMED_UNIT ( * ) SI_UNIT ( .MILLI., .METRE. ) );
#4127=CARTESIAN_POINT ( 'NONE',  ( 159.0000000000000284, -12.00000000000000000, -4.000000000000002665 ) ) ;
#4128=DIRECTION ( 'NONE',  ( 1.000000000000000000, 0.000000000000000000, 0.000000000000000000 ) ) ;
#4133=EDGE_CURVE ( 'NONE', #17999, #13456, #16071, .T. ) ;
#4136=LINE ( 'NONE', #27928, #20998 ) ;
#4140=EDGE_LOOP ( 'NONE', ( #6308, #4388, #17370, #1595 ) ) ;
#4142=CARTESIAN_POINT ( 'NONE',  ( -1.000000000000000888, 0.000000000000000000, -5.000000000000004441 ) ) ;
#4144=CARTESIAN_POINT ( 'NONE',  ( 138.2023502691896510, 0.000000000000000000, -5.000000000000004441 ) ) ;
#4145=DIRECTION ( 'NONE',  ( 1.000000000000000000, 1.067522139062651411E-16, -0.000000000000000000 ) ) ;
#4155=CARTESIAN_POINT ( 'NONE',  ( 139.8750000000000284, 0.000000000000000000, 6.000000000000005329 ) ) ;
#4156=VERTEX_POINT ( 'NONE', #17403 ) ;
#4162=CARTESIAN_POINT ( 'NONE',  ( 136.2261751345948539, -3.889087296526011706, -3.889087296526011706 ) ) ;
#4164=CARTESIAN_POINT ( 'NONE',  ( 135.5105870461000279, -9.078052452530132044, -8.000000000000007105 ) ) ;
#4165=CARTESIAN_POINT ( 'NONE',  ( 145.6726497308104058, -5.000000000000004441, 0.000000000000000000 ) ) ;
#4166=DIRECTION ( 'NONE',  ( -0.000000000000000000, -0.6000000000000000888, -0.8000000000000001554 ) ) ;
#4171=CARTESIAN_POINT ( 'NONE',  ( -4.999999999999886313, -15.00000000000001421, 7.500000000000007105 ) ) ;
#4172=DIRECTION ( 'NONE',  ( 1.000000000000000000, -0.000000000000000000, -0.000000000000000000 ) ) ;
#4176=DIRECTION ( 'NONE',  ( -0.000000000000000000, -1.000000000000000000, 0.000000000000000000 ) ) ;
#4179=APPLICATION_CONTEXT ( 'automotive_design' ) ;
#4187=ORIENTED_EDGE ( 'NONE', *, *, #24710, .F. ) ;
#4189=CARTESIAN_POINT ( 'NONE',  ( 148.6875000000000284, 4.242640687119269671, 4.242640687119298093 ) ) ;
#4191=CARTESIAN_POINT ( 'NONE',  ( 140.2500000000000284, -6.000000000000005329, 0.000000000000000000 ) ) ;
#4199=CIRCLE ( 'NONE', #11606, 9.999999999999980460 ) ;
#4201=CIRCLE ( 'NONE', #25284, 1.000000000000000000 ) ;
#4202=ADVANCED_FACE ( 'NONE', ( #26828 ), #12173, .T. ) ;
#4204=CARTESIAN_POINT ( 'NONE',  ( 140.5384615384615756, -11.07692307692308908, -4.615384615384614975 ) ) ;
#4205=DIRECTION ( 'NONE',  ( 0.000000000000000000, -1.000000000000000000, 0.000000000000000000 ) ) ;
#4206=PRODUCT_CONTEXT ( 'NONE', #24772, 'mechanical' ) ;
#4210=CARTESIAN_POINT ( 'NONE',  ( -9.999999999999793943, 9.000000000000007105, 4.000000000000003553 ) ) ;
#4216=CARTESIAN_POINT ( 'NONE',  ( 148.2336002691896510, -4.999999999999989342, 2.071067811865468400 ) ) ;
#4218=DIRECTION ( 'NONE',  ( 1.000000000000000000, 1.067522139062651411E-16, -0.000000000000000000 ) ) ;
#4219=DIRECTION ( 'NONE',  ( 0.000000000000000000, 0.000000000000000000, 1.000000000000000000 ) ) ;
#4225=VERTEX_POINT ( 'NONE', #21436 ) ;
#4226=CARTESIAN_POINT ( 'NONE',  ( 153.6562500000000568, -6.000000000000005329, 2.485281374238555774 ) ) ;
#4236=CARTESIAN_POINT ( 'NONE',  ( 159.0000000000000284, -12.00000000000001066, 5.000000000000004441 ) ) ;
#4237=CARTESIAN_POINT ( 'NONE',  ( 140.0000000000000284, -54.99999999999990763, 7.500000000000007105 ) ) ;
#4238=EDGE_CURVE ( 'NONE', #20811, #6421, #8176, .T. ) ;
#4243=CARTESIAN_POINT ( 'NONE',  ( 147.5550748654052313, -5.500000000000012434, -2.278174593052012309 ) ) ;
#4251=CARTESIAN_POINT ( 'NONE',  ( 158.6398502691896510, -3.535533905932752852, 3.535533905932725318 ) ) ;
#4253=CARTESIAN_POINT ( 'NONE',  ( 0.7528846038989732703, -15.55265717403477232, 8.022794483535989229 ) ) ;
#4254=AXIS2_PLACEMENT_3D ( 'NONE', #6078, #10876, #1001 ) ;
#4260=CARTESIAN_POINT ( 'NONE',  ( 158.0699251345948255, 2.278174593052198382, 5.499999999999826805 ) ) ;
#4261=ORIENTED_EDGE ( 'NONE', *, *, #20032, .T. ) ;
#4262=SURFACE_SIDE_STYLE ('',( #6569 ) ) ;
#4267=CARTESIAN_POINT ( 'NONE',  ( 159.0863248654052597, 0.000000000000000000, 5.500000000000005329 ) ) ;
#4270=VERTEX_POINT ( 'NONE', #18998 ) ;
#4271=CARTESIAN_POINT ( 'NONE',  ( 149.7187500000000568, 2.485281374238555774, -6.000000000000005329 ) ) ;
#4281=PRESENTATION_STYLE_ASSIGNMENT (( #9054 ) ) ;
#4285=LINE ( 'NONE', #9205, #22081 ) ;
#4286=EDGE_CURVE ( 'NONE', #11502, #13173, #26170, .T. ) ;
#4289=DIRECTION ( 'NONE',  ( -1.000000000000000000, 0.000000000000000000, 0.000000000000000000 ) ) ;
#4294=CARTESIAN_POINT ( 'NONE',  ( -0.4963810631259262252, -9.251809468437068418, -4.126213593628771825 ) ) ;
#4301=CARTESIAN_POINT ( 'NONE',  ( 136.4136751345948539, 0.000000000000000000, -5.500000000000005329 ) ) ;
#4303=DIRECTION ( 'NONE',  ( 1.000000000000000000, 0.000000000000000000, 0.000000000000000000 ) ) ;
#4305=CARTESIAN_POINT ( 'NONE',  ( 136.6086002691896510, -2.071067811865468400, -4.999999999999989342 ) ) ;
#4308=CARTESIAN_POINT ( 'NONE',  ( 151.2113248654052313, 5.500000000000005329, 0.000000000000000000 ) ) ;
#4316=CARTESIAN_POINT ( 'NONE',  ( 142.1250000000000284, 0.000000000000000000, -6.000000000000005329 ) ) ;
#4325=CARTESIAN_POINT ( 'NONE',  ( 143.7038997308103774, 2.071067811865468400, 4.999999999999989342 ) ) ;
#4329=DIRECTION ( 'NONE',  ( 0.000000000000000000, 1.000000000000000000, 0.000000000000000000 ) ) ;
#4334=EDGE_LOOP ( 'NONE', ( #21111, #21534, #22640, #12031, #23846 ) ) ;
#4338=CARTESIAN_POINT ( 'NONE',  ( 141.7500000000000568, -6.000000000000005329, 0.000000000000000000 ) ) ;
#4339=CARTESIAN_POINT ( 'NONE',  ( 140.0000000000000284, -8.500000000000007105, 5.000000000000004441 ) ) ;
#4340=CARTESIAN_POINT ( 'NONE',  ( 139.1250000000000284, 0.000000000000000000, -6.000000000000005329 ) ) ;
#4345=ORIENTED_EDGE ( 'NONE', *, *, #19325, .T. ) ;
#4362=CARTESIAN_POINT ( 'NONE',  ( -0.3854532388872732307, -9.307273380556338793, 4.200333198739636842 ) ) ;
#4368=DIRECTION ( 'NONE',  ( 0.000000000000000000, 0.000000000000000000, 1.000000000000000000 ) ) ;
#4369=CARTESIAN_POINT ( 'NONE',  ( 157.5937500000000284, 6.000000000000005329, 2.485281374238585972 ) ) ;
#4372=CIRCLE ( 'NONE', #21563, 15.00000000000000000 ) ;
#4374=FILL_AREA_STYLE_COLOUR ( '', #14540 ) ;
#4375=ORIENTED_EDGE ( 'NONE', *, *, #22507, .F. ) ;
#4376=CARTESIAN_POINT ( 'NONE',  ( 156.5625000000000284, -4.242640687119298093, 4.242640687119298093 ) ) ;
#4379=ADVANCED_FACE ( 'NONE', ( #368 ), #19509, .F. ) ;
#4383=ORIENTED_EDGE ( 'NONE', *, *, #4839, .T. ) ;
#4388=ORIENTED_EDGE ( 'NONE', *, *, #26976, .T. ) ;
#4390=CARTESIAN_POINT ( 'NONE',  ( 1.000000000000000888, -14.99923475244191451, 9.015151515151503148 ) ) ;
#4392=EDGE_LOOP ( 'NONE', ( #21286, #10171, #17906, #1588 ) ) ;
#4394=CARTESIAN_POINT ( 'NONE',  ( -9.999999999999994671, -71.00000000000002842, 5.000000000000004441 ) ) ;
#4397=CARTESIAN_POINT ( 'NONE',  ( 147.4613248654052029, -5.500000000000005329, 0.000000000000000000 ) ) ;
#4405=SURFACE_SIDE_STYLE ('',( #2419 ) ) ;
#4406=CARTESIAN_POINT ( 'NONE',  ( 0.1659452612680607231, -15.34501306676551202, 8.417236167508884037 ) ) ;
#4418=( GEOMETRIC_REPRESENTATION_CONTEXT ( 3 ) GLOBAL_UNCERTAINTY_ASSIGNED_CONTEXT ( ( #9677 ) ) GLOBAL_UNIT_ASSIGNED_CONTEXT ( ( #14808, #10341, #29047 ) ) REPRESENTATION_CONTEXT ( 'NONE', 'WORKASPACE' ) );
#4422=CARTESIAN_POINT ( 'NONE',  ( 147.8437500000000284, -6.000000000000005329, -2.485281374238555774 ) ) ;
#4428=ORIENTED_EDGE ( 'NONE', *, *, #3402, .F. ) ;
#4429=PRESENTATION_STYLE_ASSIGNMENT (( #16156 ) ) ;
#4432=CARTESIAN_POINT ( 'NONE',  ( 160.9999999919967877, -11.61962113023372289, 3.007375573655278966 ) ) ;
#4433=SURFACE_STYLE_USAGE ( .BOTH. , #5135 ) ;
#4435=CARTESIAN_POINT ( 'NONE',  ( 0.7580070251407292625, -15.51657223718414791, -8.092363357809270852 ) ) ;
#4436=CIRCLE ( 'NONE', #6246, 0.5000000000000004441 ) ;
#4437=DIRECTION ( 'NONE',  ( 0.000000000000000000, 0.000000000000000000, 1.000000000000000000 ) ) ;
#4445=CARTESIAN_POINT ( 'NONE',  ( -9.757819552369539906E-16, -10.00000000000000888, -5.000000000000004441 ) ) ;
#4446=LINE ( 'NONE', #18155, #18692 ) ;
#4449=CARTESIAN_POINT ( 'NONE',  ( 135.2765744903421137, -8.508179439634940167, -8.095374785726331623 ) ) ;
#4450=DIRECTION ( 'NONE',  ( 0.000000000000000000, 0.000000000000000000, 1.000000000000000000 ) ) ;
#4466=ORIENTED_EDGE ( 'NONE', *, *, #6923, .F. ) ;
#4468=CARTESIAN_POINT ( 'NONE',  ( 134.8125000000000284, 4.242640687119298093, -4.242640687119298093 ) ) ;
#4471=MECHANICAL_DESIGN_GEOMETRIC_PRESENTATION_REPRESENTATION('',(#29966),#21181);
#4474=CARTESIAN_POINT ( 'NONE',  ( 125.0000000000000568, -55.00000000000000711, 8.000000000000007105 ) ) ;
#4476=CARTESIAN_POINT ( 'NONE',  ( 134.9304254777555911, -7.819842479424068848, -8.000000000000007105 ) ) ;
#4477=CARTESIAN_POINT ( 'NONE',  ( 141.3601497308104058, -3.535533905932725318, -3.535533905932725318 ) ) ;
#4480=CARTESIAN_POINT ( 'NONE',  ( 129.9999999999998010, -90.00000000000001421, -3.000000000000002665 ) ) ;
#4483=( NAMED_UNIT ( * ) PLANE_ANGLE_UNIT ( ) SI_UNIT ( $, .RADIAN. ) );
#4490=TOROIDAL_SURFACE ( 'NONE', #3005, 28.99999999999999645, 1.000000000000000000 ) ;
#4493=DIRECTION ( 'NONE',  ( 0.000000000000000000, 0.000000000000000000, 1.000000000000000000 ) ) ;
#4497=CARTESIAN_POINT ( 'NONE',  ( 137.9062500000000568, 6.000000000000005329, -2.485281374238556218 ) ) ;
#4499=CARTESIAN_POINT ( 'NONE',  ( -15.49999999999999289, -25.00000000000007816, -8.000000000000007105 ) ) ;
#4501=CARTESIAN_POINT ( 'NONE',  ( 132.1875000000000284, 4.242640687119269671, 4.242640687119298093 ) ) ;
#4503=CIRCLE ( 'NONE', #11409, 17.50000000000000355 ) ;
#4506=ORIENTED_EDGE ( 'NONE', *, *, #2655, .F. ) ;
#4509=EDGE_LOOP ( 'NONE', ( #560, #29654, #25424, #12185 ) ) ;
#4515=CARTESIAN_POINT ( 'NONE',  ( -19.49999999999998224, -25.00000000000010658, -7.500000000000007105 ) ) ;
#4519=CARTESIAN_POINT ( 'NONE',  ( 140.0000000000000284, -10.00000000000000888, -7.500000000000007105 ) ) ;
#4522=LINE ( 'NONE', #26158, #23454 ) ;
#4527=CARTESIAN_POINT ( 'NONE',  ( 148.0461002691896510, -2.071067811865468400, 4.999999999999989342 ) ) ;
#4529=CARTESIAN_POINT ( 'NONE',  ( 1.000000000000000888, 0.000000000000000000, 0.000000000000000000 ) ) ;
#4530=CARTESIAN_POINT ( 'NONE',  ( 160.9687500000000568, -2.485281374238585972, 6.000000000000005329 ) ) ;
#4534=DIRECTION ( 'NONE',  ( 0.000000000000000000, 0.000000000000000000, 1.000000000000000000 ) ) ;
#4536=ORIENTED_EDGE ( 'NONE', *, *, #17911, .F. ) ;
#4537=CARTESIAN_POINT ( 'NONE',  ( 156.2812500000000284, 2.485281374238585972, 6.000000000000005329 ) ) ;
#4549=DIRECTION ( 'NONE',  ( 0.000000000000000000, 0.000000000000000000, -1.000000000000000000 ) ) ;
#4550=DIRECTION ( 'NONE',  ( 0.000000000000000000, 1.000000000000000000, 0.000000000000000000 ) ) ;
#4553=ORIENTED_EDGE ( 'NONE', *, *, #11147, .T. ) ;
#4555=STYLED_ITEM ( 'NONE', ( #4829 ), #22508 ) ;
#4564=CARTESIAN_POINT ( 'NONE',  ( 159.2023502691896510, 0.000000000000000000, -5.000000000000004441 ) ) ;
#4565=CARTESIAN_POINT ( 'NONE',  ( 135.0101475501562049, -7.374327361089822119, 8.398546155689757597 ) ) ;
#4566=VERTEX_POINT ( 'NONE', #17294 ) ;
#4571=ADVANCED_FACE ( 'NONE', ( #6657 ), #20648, .F. ) ;
#4575=( NAMED_UNIT ( * ) SI_UNIT ( $, .STERADIAN. ) SOLID_ANGLE_UNIT ( ) );
#4578=CARTESIAN_POINT ( 'NONE',  ( 152.0625000000000568, -4.242640687119298093, 4.242640687119298093 ) ) ;
#4584=CARTESIAN_POINT ( 'NONE',  ( 137.3363248654052029, 0.000000000000000000, -5.500000000000005329 ) ) ;
#4588=CARTESIAN_POINT ( 'NONE',  ( -0.08172395017747559332, -15.06317155720421930, -7.964553512345503350 ) ) ;
#4589=CARTESIAN_POINT ( 'NONE',  ( 153.0074251345948255, 2.278174593052074925, -5.499999999999950262 ) ) ;
#4590=DIRECTION ( 'NONE',  ( 0.000000000000000000, 0.000000000000000000, 1.000000000000000000 ) ) ;
#4594=CARTESIAN_POINT ( 'NONE',  ( -0.5000000001309222730, -10.00000000000000888, -4.869076758059778243 ) ) ;
#4595=EDGE_CURVE ( 'NONE', #24916, #18033, #3184, .T. ) ;
#4596=CARTESIAN_POINT ( 'NONE',  ( -0.5000000000000004441, -15.50000000000001421, -7.500000000000007105 ) ) ;
#4601=EDGE_LOOP ( 'NONE', ( #15848, #25840, #21184, #11667 ) ) ;
#4603=CARTESIAN_POINT ( 'NONE',  ( 143.5386751345948255, -5.500000000000005329, 0.000000000000000000 ) ) ;
#4604=EDGE_CURVE ( 'NONE', #24916, #27766, #29792, .T. ) ;
#4612=ORIENTED_EDGE ( 'NONE', *, *, #2655, .T. ) ;
#4613=ORIENTED_EDGE ( 'NONE', *, *, #1013, .F. ) ;
#4615=CARTESIAN_POINT ( 'NONE',  ( 133.3125000000000284, 4.242640687119298093, -4.242640687119298093 ) ) ;
#4619=( LENGTH_UNIT ( ) NAMED_UNIT ( * ) SI_UNIT ( .MILLI., .METRE. ) );
#4623=CARTESIAN_POINT ( 'NONE',  ( 144.7351497308104058, 3.535533905932725318, -3.535533905932725318 ) ) ;
#4633=DIRECTION ( 'NONE',  ( 1.000000000000000000, 0.000000000000000000, 0.000000000000000000 ) ) ;
#4635=FILL_AREA_STYLE_COLOUR ( '', #24824 ) ;
#4642=CARTESIAN_POINT ( 'NONE',  ( 141.0000000000000284, 6.000000000000005329, 0.000000000000000000 ) ) ;
#4646=MECHANICAL_DESIGN_GEOMETRIC_PRESENTATION_REPRESENTATION('',(#14023),#7105);
#4648=CARTESIAN_POINT ( 'NONE',  ( 134.0625000000000284, -4.242640687119298093, 4.242640687119298093 ) ) ;
#4656=DIRECTION ( 'NONE',  ( 0.000000000000000000, 0.000000000000000000, -1.000000000000000000 ) ) ;
#4665=CARTESIAN_POINT ( 'NONE',  ( 140.0758535114726726, -9.341226305241869809, -7.537168216789017272 ) ) ;
#4670=CARTESIAN_POINT ( 'NONE',  ( -9.999999999999980460, -60.00000000000001421, 3.000000000000002665 ) ) ;
#4671=CARTESIAN_POINT ( 'NONE',  ( -4.999999999999886313, -10.00000000000000888, 7.500000000000007105 ) ) ;
#4673=CARTESIAN_POINT ( 'NONE',  ( 155.5312500000000284, -2.485281374238556218, -6.000000000000005329 ) ) ;
#4675=AXIS2_PLACEMENT_3D ( 'NONE', #3868, #11289, #13443 ) ;
#4676=FILL_AREA_STYLE ('',( #7137 ) ) ;
#4682=CARTESIAN_POINT ( 'NONE',  ( 149.9062500000000568, 6.000000000000005329, -2.485281374238555774 ) ) ;
#4685=ORIENTED_EDGE ( 'NONE', *, *, #1779, .T. ) ;
#4686=ORIENTED_EDGE ( 'NONE', *, *, #15120, .F. ) ;
#4687=CIRCLE ( 'NONE', #29701, 0.5000000000000004441 ) ;
#4693=CARTESIAN_POINT ( 'NONE',  ( 157.6726497308104058, -5.000000000000004441, 0.000000000000000000 ) ) ;
#4696=LINE ( 'NONE', #9481, #7813 ) ;
#4699=EDGE_CURVE ( 'NONE', #7475, #12687, #10989, .T. ) ;
#4706=DIRECTION ( 'NONE',  ( 1.000000000000000000, 0.000000000000000000, 0.000000000000000000 ) ) ;
#4708=DIRECTION ( 'NONE',  ( 0.000000000000000000, 0.000000000000000000, -1.000000000000000000 ) ) ;
#4709=CARTESIAN_POINT ( 'NONE',  ( 160.2336002691896226, -4.999999999999989342, 2.071067811865468400 ) ) ;
#4710=CARTESIAN_POINT ( 'NONE',  ( 135.0000000000002842, -7.177308154933044193, 8.449997537985554530 ) ) ;
#4714=CARTESIAN_POINT ( 'NONE',  ( 136.0000000000000284, 0.000000000000000000, -11.00000000000000355 ) ) ;
#4716=FACE_OUTER_BOUND ( 'NONE', #1667, .T. ) ;
#4718=AXIS2_PLACEMENT_3D ( 'NONE', #23871, #12681, #16986 ) ;
#4720=CYLINDRICAL_SURFACE ( 'NONE', #15811, 0.5000000000000004441 ) ;
#4724=CARTESIAN_POINT ( 'NONE',  ( -40.00000000000000000, -20.00000000000021316, 3.000000000000002665 ) ) ;
#4727=CARTESIAN_POINT ( 'NONE',  ( 152.5312500000000000, -2.485281374238555774, -6.000000000000005329 ) ) ;
#4729=EDGE_CURVE ( 'NONE', #9839, #11992, #29657, .T. ) ;
#4734=CARTESIAN_POINT ( 'NONE',  ( -4.999999999999879208, -71.00000000000002842, 4.000000000000003553 ) ) ;
#4737=SURFACE_SIDE_STYLE ('',( #9813 ) ) ;
#4740=CARTESIAN_POINT ( 'NONE',  ( 0.7548275425895982771, -15.52547035223602734, -8.075280843867185254 ) ) ;
#4743=DIRECTION ( 'NONE',  ( 0.000000000000000000, 0.000000000000000000, 1.000000000000000000 ) ) ;
#4747=CARTESIAN_POINT ( 'NONE',  ( -0.2003331987396576308, -9.399833400630168256, -4.385453238887252247 ) ) ;
#4749=CARTESIAN_POINT ( 'NONE',  ( 160.2059167087800802, -11.22359236516978775, -4.246869790297142622 ) ) ;
#4751=CARTESIAN_POINT ( 'NONE',  ( 135.0000000000000284, -7.800712729749759156, -7.983520772873845317 ) ) ;
#4755=CARTESIAN_POINT ( 'NONE',  ( 143.3511751345948255, -3.889087296526011706, 3.889087296526011706 ) ) ;
#4757=AXIS2_PLACEMENT_3D ( 'NONE', #3047, #2461, #21663 ) ;
#4759=CIRCLE ( 'NONE', #20466, 11.00000000000000355 ) ;
#4760=CARTESIAN_POINT ( 'NONE',  ( 151.5863248654052313, 0.000000000000000000, 5.500000000000005329 ) ) ;
#4763=CARTESIAN_POINT ( 'NONE',  ( 140.3363248654052029, 0.000000000000000000, -5.500000000000005329 ) ) ;
#4767=CARTESIAN_POINT ( 'NONE',  ( 136.5000000000000284, 6.000000000000005329, 0.000000000000000000 ) ) ;
#4768=EDGE_CURVE ( 'NONE', #8327, #14623, #21106, .T. ) ;
#4774=COLOUR_RGB ( '', 0.72549020, 0.75294118, 0.79215686) ;
#4776=CARTESIAN_POINT ( 'NONE',  ( 0.07033120956265798140, -15.06949959929781357, 8.898246228163568361 ) ) ;
#4777=EDGE_CURVE ( 'NONE', #379, #22958, #27831, .T. ) ;
#4779=CARTESIAN_POINT ( 'NONE',  ( 146.0476497308104058, 0.000000000000000000, -5.000000000000004441 ) ) ;
#4789=DIRECTION ( 'NONE',  ( 1.000000000000000000, -0.000000000000000000, -0.000000000000000000 ) ) ;
#4792=CARTESIAN_POINT ( 'NONE',  ( 142.7812500000000568, 2.485281374238585972, 6.000000000000005329 ) ) ;
#4796=CARTESIAN_POINT ( 'NONE',  ( 133.1250000000000284, 0.000000000000000000, -6.000000000000005329 ) ) ;
#4801=VECTOR ( 'NONE', #2571, 1000.000000000000000 ) ;
#4805=CARTESIAN_POINT ( 'NONE',  ( 140.2574251345947687, -2.278174593051702335, 5.500000000000323297 ) ) ;
#4807=EDGE_CURVE ( 'NONE', #27377, #27416, #12654, .T. ) ;
#4812=CARTESIAN_POINT ( 'NONE',  ( 140.5126539824821634, -11.05214782318283184, 4.674845224361170004 ) ) ;
#4824=CARTESIAN_POINT ( 'NONE',  ( 143.3586002691896226, 2.071067811865468400, 4.999999999999989342 ) ) ;
#4826=CARTESIAN_POINT ( 'NONE',  ( 155.3437500000000284, -6.000000000000005329, -2.485281374238556218 ) ) ;
#4827=SURFACE_SIDE_STYLE ('',( #2241 ) ) ;
#4829=PRESENTATION_STYLE_ASSIGNMENT (( #12095 ) ) ;
#4832=DIRECTION ( 'NONE',  ( 0.000000000000000000, 0.000000000000000000, -1.000000000000000000 ) ) ;
#4834=CARTESIAN_POINT ( 'NONE',  ( 152.3437500000000568, -6.000000000000005329, -2.485281374238555774 ) ) ;
#4837=CARTESIAN_POINT ( 'NONE',  ( 140.0255071013316410, -11.51275355066580453, 4.738782956804194590 ) ) ;
#4838=VERTEX_POINT ( 'NONE', #4499 ) ;
#4839=EDGE_CURVE ( 'NONE', #27076, #23117, #13922, .T. ) ;
#4844=CARTESIAN_POINT ( 'NONE',  ( 155.8913997308104342, -2.071067811865468400, 4.999999999999989342 ) ) ;
#4845=CARTESIAN_POINT ( 'NONE',  ( 159.5550748654052313, -5.500000000000012434, -2.278174593052012309 ) ) ;
#4846=CARTESIAN_POINT ( 'NONE',  ( 136.0000000000000284, -8.798545334315202027, 8.160000000000007248 ) ) ;
#4851=( BOUNDED_CURVE ( )  B_SPLINE_CURVE ( 2, ( #20667, #8990, #10861, #27244, #8366, #3590, #1758, #15791, #15476 ),
 .UNSPECIFIED., .F., .F. ) 
 B_SPLINE_CURVE_WITH_KNOTS ( ( 3, 2, 2, 2, 3 ),
 ( 0.1625000000000006162, 0.1687500000000003997, 0.1750000000000001554, 0.1812499999999999112, 0.1874999999999996947 ),
 .UNSPECIFIED. ) 
 CURVE ( )  GEOMETRIC_REPRESENTATION_ITEM ( )  RATIONAL_B_SPLINE_CURVE ( ( 0.9999999999999925615, 0.9238795325112941770, 1.000000000000000000, 0.9238795325112867385, 1.000000000000000000, 0.9238795325112867385, 1.000000000000000000, 0.9238795325112904022, 0.9999999999999963363 ) ) 
 REPRESENTATION_ITEM ( '' )  );
#4852=AXIS2_PLACEMENT_3D ( 'NONE', #279, #2295, #11699 ) ;
#4858=CARTESIAN_POINT ( 'NONE',  ( 0.000000000000000000, -9.500000000000008882, -5.000000000000004441 ) ) ;
#4867=CARTESIAN_POINT ( 'NONE',  ( -1.000000000000000888, 9.000000000000007105, -5.000000000000004441 ) ) ;
#4868=ORIENTED_EDGE ( 'NONE', *, *, #28138, .F. ) ;
#4870=EDGE_CURVE ( 'NONE', #13568, #21900, #23464, .T. ) ;
#4871=CARTESIAN_POINT ( 'NONE',  ( 153.1875000000000284, 4.242640687119269671, 4.242640687119298093 ) ) ;
#4880=FACE_OUTER_BOUND ( 'NONE', #7545, .T. ) ;
#4881=VECTOR ( 'NONE', #11006, 1000.000000000000000 ) ;
#4883=( NAMED_UNIT ( * ) SI_UNIT ( $, .STERADIAN. ) SOLID_ANGLE_UNIT ( ) );
#4888=CYLINDRICAL_SURFACE ( 'NONE', #1331, 0.5000000000000004441 ) ;
#4892=CARTESIAN_POINT ( 'NONE',  ( 135.0000000000000284, -7.345688489539636379, -8.346135564586871780 ) ) ;
#4897=AXIS2_PLACEMENT_3D ( 'NONE', #1680, #15552, #13248 ) ;
#4900=MECHANICAL_DESIGN_GEOMETRIC_PRESENTATION_REPRESENTATION('',(#10316),#16277);
#4901=EDGE_LOOP ( 'NONE', ( #19359, #27673, #23972, #12053 ) ) ;
#4902=FACE_OUTER_BOUND ( 'NONE', #2580, .T. ) ;
#4906=ADVANCED_FACE ( 'NONE', ( #929 ), #3284, .T. ) ;
#4911=CARTESIAN_POINT ( 'NONE',  ( 134.5312500000000568, -2.485281374238555774, -6.000000000000005329 ) ) ;
#4912=ORIENTED_EDGE ( 'NONE', *, *, #23390, .F. ) ;
#4914=SURFACE_STYLE_FILL_AREA ( #14199 ) ;
#4918=CARTESIAN_POINT ( 'NONE',  ( 137.7038997308103774, 2.071067811865468400, 4.999999999999989342 ) ) ;
#4923=CARTESIAN_POINT ( 'NONE',  ( -0.07769256095284393648, -15.23231281889969679, 7.500000000000007105 ) ) ;
#4927=FILL_AREA_STYLE ('',( #18798 ) ) ;
#4928=FILL_AREA_STYLE ('',( #4635 ) ) ;
#4935=VERTEX_POINT ( 'NONE', #24140 ) ;
#4937=CARTESIAN_POINT ( 'NONE',  ( 142.1250000000000284, 0.000000000000000000, -6.000000000000005329 ) ) ;
#4939=CARTESIAN_POINT ( 'NONE',  ( 138.8363248654052029, 0.000000000000000000, -5.500000000000005329 ) ) ;
#4942=CARTESIAN_POINT ( 'NONE',  ( 160.0163997308104342, 4.999999999999989342, 2.071067811865468400 ) ) ;
#4958=CARTESIAN_POINT ( 'NONE',  ( 139.9157253400916829, -9.546725596017704873, 7.785029603303435408 ) ) ;
#4961=DIRECTION ( 'NONE',  ( -6.938893903907222067E-15, 1.000000000000000000, 0.000000000000000000 ) ) ;
#4969=CARTESIAN_POINT ( 'NONE',  ( 160.3125000000000284, 4.242640687119298093, -4.242640687119298093 ) ) ;
#4970=LINE ( 'NONE', #3259, #20236 ) ;
#4975=ORIENTED_EDGE ( 'NONE', *, *, #23661, .T. ) ;
#4976=CARTESIAN_POINT ( 'NONE',  ( 151.6875000000000284, 4.242640687119269671, 4.242640687119298093 ) ) ;
#4979=AXIS2_PLACEMENT_3D ( 'NONE', #739, #14737, #16761 ) ;
#4980=CARTESIAN_POINT ( 'NONE',  ( 140.5000000000000284, -10.00000000000000888, -7.500000000000007105 ) ) ;
#4983=ORIENTED_EDGE ( 'NONE', *, *, #28715, .F. ) ;
#4985=ORIENTED_EDGE ( 'NONE', *, *, #4286, .T. ) ;
#4987=DIRECTION ( 'NONE',  ( -6.938893903907221278E-15, 1.000000000000000000, 0.000000000000000000 ) ) ;
#4988=CARTESIAN_POINT ( 'NONE',  ( 153.7351497308104342, 3.535533905932725318, -3.535533905932725318 ) ) ;
#4989=AXIS2_PLACEMENT_3D ( 'NONE', #29065, #3116, #2669 ) ;
#4990=FACE_OUTER_BOUND ( 'NONE', #6258, .T. ) ;
#4992=DIRECTION ( 'NONE',  ( -0.000000000000000000, 1.000000000000000000, -1.224646799147353207E-16 ) ) ;
#4997=EDGE_CURVE ( 'NONE', #19034, #2328, #21363, .T. ) ;
#5004=AXIS2_PLACEMENT_3D ( 'NONE', #3702, #27203, #10343 ) ;
#5005=UNCERTAINTY_MEASURE_WITH_UNIT (LENGTH_MEASURE( 1.000000000000000082E-05 ), #1107, 'distance_accuracy_value', 'NONE');
#5021=CARTESIAN_POINT ( 'NONE',  ( 158.5238248654052313, 3.889087296526011706, -3.889087296526011706 ) ) ;
#5024=CARTESIAN_POINT ( 'NONE',  ( 132.9226497308104058, 5.000000000000004441, 0.000000000000000000 ) ) ;
#5027=DIRECTION ( 'NONE',  ( -1.000000000000000000, 0.000000000000000000, 0.000000000000000000 ) ) ;
#5030=FACE_OUTER_BOUND ( 'NONE', #26849, .T. ) ;
#5035=CARTESIAN_POINT ( 'NONE',  ( 160.9323586472526699, -11.54909004507883452, -3.261009256920451627 ) ) ;
#5036=UNCERTAINTY_MEASURE_WITH_UNIT (LENGTH_MEASURE( 1.000000000000000082E-05 ), #25270, 'distance_accuracy_value', 'NONE');
#5037=ADVANCED_FACE ( 'NONE', ( #20154 ), #18122, .F. ) ;
#5039=LINE ( 'NONE', #7060, #23990 ) ;
#5041=ORIENTED_EDGE ( 'NONE', *, *, #15196, .F. ) ;
#5043=DIRECTION ( 'NONE',  ( 1.000000000000000000, 1.734723475976843579E-16, -0.000000000000000000 ) ) ;
#5046=ORIENTED_EDGE ( 'NONE', *, *, #22479, .T. ) ;
#5050=CARTESIAN_POINT ( 'NONE',  ( 162.0000000000000284, 0.000000000000000000, 0.000000000000000000 ) ) ;
#5051=VERTEX_POINT ( 'NONE', #8467 ) ;
#5052=CARTESIAN_POINT ( 'NONE',  ( 157.1324251345948539, -5.500000000000012434, -2.278174593052012309 ) ) ;
#5053=EDGE_LOOP ( 'NONE', ( #26689, #12890, #18667, #27412 ) ) ;
#5055=CARTESIAN_POINT ( 'NONE',  ( 138.0000000000000284, 6.000000000000005329, 0.000000000000000000 ) ) ;
#5063=EDGE_LOOP ( 'NONE', ( #5862, #29537, #1055, #3465 ) ) ;
#5066=DIRECTION ( 'NONE',  ( 1.000000000000000000, 0.000000000000000000, 0.000000000000000000 ) ) ;
#5068=CARTESIAN_POINT ( 'NONE',  ( -1.000000000000000888, -9.000000000000007105, 4.000000000000003553 ) ) ;
#5069=CARTESIAN_POINT ( 'NONE',  ( 135.7351497308104058, 3.535533905932725318, -3.535533905932725318 ) ) ;
#5078=CARTESIAN_POINT ( 'NONE',  ( -4.999999999999990230, -24.99999999999999289, 5.000000000000004441 ) ) ;
#5085=CARTESIAN_POINT ( 'NONE',  ( 133.3125000000000284, 4.242640687119298093, -4.242640687119298093 ) ) ;
#5090=B_SPLINE_CURVE_WITH_KNOTS ( 'NONE', 3,
 ( #26641, #15004, #7219, #10397 ),
 .UNSPECIFIED., .F., .F.,
 ( 4, 4 ),
 ( 0.000000000000000000, 0.0007771587456802753549 ),
 .UNSPECIFIED. ) ;
#5094=CARTESIAN_POINT ( 'NONE',  ( 124.9999999999999432, -70.00000000000000000, 5.000000000000004441 ) ) ;
#5108=CARTESIAN_POINT ( 'NONE',  ( 139.9892236744308889, -9.817200068377076150, 7.619547926460280785 ) ) ;
#5110=CARTESIAN_POINT ( 'NONE',  ( 146.6175748654052313, 5.500000000000012434, -2.278174593052012309 ) ) ;
#5112=CARTESIAN_POINT ( 'NONE',  ( 145.5863248654052313, 0.000000000000000000, 5.500000000000005329 ) ) ;
#5115=CARTESIAN_POINT ( 'NONE',  ( 144.6711002691896226, 4.999999999999989342, 2.071067811865468400 ) ) ;
#5117=CARTESIAN_POINT ( 'NONE',  ( 154.1250000000000284, 0.000000000000000000, -6.000000000000005329 ) ) ;
#5120=CARTESIAN_POINT ( 'NONE',  ( 149.8125000000000568, 4.242640687119298093, -4.242640687119298093 ) ) ;
#5122=VECTOR ( 'NONE', #14563, 1000.000000000000000 ) ;
#5123=UNCERTAINTY_MEASURE_WITH_UNIT (LENGTH_MEASURE( 1.000000000000000082E-05 ), #21918, 'distance_accuracy_value', 'NONE');
#5128=ORIENTED_EDGE ( 'NONE', *, *, #17146, .T. ) ;
#5129=ADVANCED_FACE ( 'NONE', ( #23525 ), #11883, .T. ) ;
#5135=SURFACE_SIDE_STYLE ('',( #16863 ) ) ;
#5139=DIRECTION ( 'NONE',  ( 1.000000000000000000, 1.067522139062651904E-16, -0.000000000000000000 ) ) ;
#5146=AXIS2_PLACEMENT_3D ( 'NONE', #12244, #24427, #15248 ) ;
#5151=CARTESIAN_POINT ( 'NONE',  ( 154.9836002691896510, 4.999999999999989342, -2.071067811865468400 ) ) ;
#5155=DIRECTION ( 'NONE',  ( 1.000000000000000000, -3.469446951953694061E-16, -0.000000000000000000 ) ) ;
#5157=DIRECTION ( 'NONE',  ( 0.000000000000000000, 0.8907235428302470170, 0.4545454545454539197 ) ) ;
#5158=( BOUNDED_CURVE ( )  B_SPLINE_CURVE ( 2, ( #1352, #10764, #20109, #29453, #17832, #1503, #6267, #5305, #404 ),
 .UNSPECIFIED., .F., .T. ) 
 B_SPLINE_CURVE_WITH_KNOTS ( ( 3, 2, 2, 2, 3 ),
 ( 0.3874999999999999001, 0.3937500000000000999, 0.4000000000000003553, 0.4062500000000006106, 0.4125000000000008105 ),
 .UNSPECIFIED. ) 
 CURVE ( )  GEOMETRIC_REPRESENTATION_ITEM ( )  RATIONAL_B_SPLINE_CURVE ( ( 1.000000000000001332, 0.9238795325112854062, 1.000000000000000000, 0.9238795325112867385, 1.000000000000000000, 0.9238795325112867385, 1.000000000000000000, 0.9238795325112766355, 1.000000000000010214 ) ) 
 REPRESENTATION_ITEM ( '' )  );
#5159=ORIENTED_EDGE ( 'NONE', *, *, #20144, .F. ) ;
#5165=EDGE_LOOP ( 'NONE', ( #20714, #9221, #6377, #25340 ) ) ;
#5167=ADVANCED_FACE ( 'NONE', ( #18620, #6915 ), #27942, .T. ) ;
#5175=CARTESIAN_POINT ( 'NONE',  ( 133.5788997308104058, -4.999999999999989342, 2.071067811865468400 ) ) ;
#5179=ADVANCED_FACE ( 'NONE', ( #7660 ), #26363, .T. ) ;
#5181=DIRECTION ( 'NONE',  ( 1.000000000000000000, 0.000000000000000000, 0.000000000000000000 ) ) ;
#5184=MECHANICAL_DESIGN_GEOMETRIC_PRESENTATION_REPRESENTATION('',(#12109),#6187);
#5188=DIRECTION ( 'NONE',  ( 0.000000000000000000, 0.000000000000000000, 1.000000000000000000 ) ) ;
#5190=CARTESIAN_POINT ( 'NONE',  ( 135.0000000000000568, -7.170799408905232042, 8.464366752364069768 ) ) ;
#5192=( NAMED_UNIT ( * ) PLANE_ANGLE_UNIT ( ) SI_UNIT ( $, .RADIAN. ) );
#5194=CARTESIAN_POINT ( 'NONE',  ( 148.5074251345948539, 2.278174593052012309, -5.500000000000012434 ) ) ;
#5196=AXIS2_PLACEMENT_3D ( 'NONE', #2001, #18314, #4450 ) ;
#5197=CARTESIAN_POINT ( 'NONE',  ( -19.49999999999998224, -54.99999999999992184, 8.000000000000007105 ) ) ;
#5206=CARTESIAN_POINT ( 'NONE',  ( 132.0000000000000284, 6.000000000000005329, 0.000000000000000000 ) ) ;
#5207=CARTESIAN_POINT ( 'NONE',  ( 133.1398502691896510, -3.535533905932752852, 3.535533905932725318 ) ) ;
#5210=EDGE_LOOP ( 'NONE', ( #11504, #24612, #26838, #16787 ) ) ;
#5219=CARTESIAN_POINT ( 'NONE',  ( 137.4226497308104058, 5.000000000000004441, 0.000000000000000000 ) ) ;
#5221=CARTESIAN_POINT ( 'NONE',  ( -4.999999999999879208, -14.50000000000001243, -8.000000000000007105 ) ) ;
#5240=VECTOR ( 'NONE', #5506, 1000.000000000000000 ) ;
#5241=CARTESIAN_POINT ( 'NONE',  ( 140.2902754521815325, -11.64513772609109132, 4.288736938852949265 ) ) ;
#5243=AXIS2_PLACEMENT_3D ( 'NONE', #9721, #19100, #477 ) ;
#5247=ORIENTED_EDGE ( 'NONE', *, *, #21909, .F. ) ;
#5254=DIRECTION ( 'NONE',  ( -6.938893903907222067E-15, 1.000000000000000000, 0.000000000000000000 ) ) ;
#5256=CARTESIAN_POINT ( 'NONE',  ( 160.0000000000000284, -59.99999999999980105, -3.000000000000002665 ) ) ;
#5257=CARTESIAN_POINT ( 'NONE',  ( 141.0000000000000284, -12.00000000000001066, -4.000000000000003553 ) ) ;
#5258=DIRECTION ( 'NONE',  ( 0.000000000000000000, 0.000000000000000000, -1.000000000000000000 ) ) ;
#5261=CARTESIAN_POINT ( 'NONE',  ( -1.000000000000000888, 9.000000000000007105, 3.000000000000002665 ) ) ;
#5266=CARTESIAN_POINT ( 'NONE',  ( 144.8363248654052029, 0.000000000000000000, -5.500000000000005329 ) ) ;
#5268=SURFACE_STYLE_FILL_AREA ( #28758 ) ;
#5269=CARTESIAN_POINT ( 'NONE',  ( 150.5625000000000568, -4.242640687119298093, 4.242640687119298093 ) ) ;
#5270=CARTESIAN_POINT ( 'NONE',  ( 135.0000000000000284, -8.851546142247588733, -7.500000000000097700 ) ) ;
#5276=CARTESIAN_POINT ( 'NONE',  ( 148.0312500000000284, -2.485281374238555774, -6.000000000000005329 ) ) ;
#5279=EDGE_CURVE ( 'NONE', #18627, #20260, #16968, .T. ) ;
#5288=CARTESIAN_POINT ( 'NONE',  ( 140.0252556714799823, -11.51262782845654620, 4.739386388448187937 ) ) ;
#5290=CARTESIAN_POINT ( 'NONE',  ( 160.6011751345948255, 3.889087296526011706, -3.889087296526011706 ) ) ;
#5294=CARTESIAN_POINT ( 'NONE',  ( 142.0238248654052029, 3.889087296526011706, -3.889087296526011706 ) ) ;
#5295=DIRECTION ( 'NONE',  ( 1.000000000000000000, 0.000000000000000000, -0.000000000000000000 ) ) ;
#5298=CARTESIAN_POINT ( 'NONE',  ( 155.8273502691896510, -5.000000000000004441, 0.000000000000000000 ) ) ;
#5305=CARTESIAN_POINT ( 'NONE',  ( 149.4300748654051745, 2.278174593051780050, -5.500000000000244249 ) ) ;
#5312=EDGE_CURVE ( 'NONE', #25253, #29814, #22573, .T. ) ;
#5314=CARTESIAN_POINT ( 'NONE',  ( 147.0937500000000284, 6.000000000000005329, 2.485281374238585972 ) ) ;
#5322=CARTESIAN_POINT ( 'NONE',  ( 132.4538997308104342, -2.071067811865468400, -4.999999999999989342 ) ) ;
#5326=CARTESIAN_POINT ( 'NONE',  ( 158.6324251345948824, -5.500000000000012434, -2.278174593052012309 ) ) ;
#5330=CARTESIAN_POINT ( 'NONE',  ( -0.08337014915864793263, -15.22335576789224199, 7.695802404352960480 ) ) ;
#5335=LINE ( 'NONE', #5485, #3091 ) ;
#5338=FILL_AREA_STYLE ('',( #10752 ) ) ;
#5343=CYLINDRICAL_SURFACE ( 'NONE', #2053, 12.00000000000000178 ) ;
#5344=EDGE_CURVE ( 'NONE', #13277, #21900, #29302, .T. ) ;
#5347=CARTESIAN_POINT ( 'NONE',  ( 15.00000000000000000, 0.000000000000000000, 0.000000000000000000 ) ) ;
#5349=AXIS2_PLACEMENT_3D ( 'NONE', #1363, #10772, #20121 ) ;
#5350=ORIENTED_EDGE ( 'NONE', *, *, #15454, .T. ) ;
#5353=CIRCLE ( 'NONE', #22550, 1.000000000000000000 ) ;
#5354=VERTEX_POINT ( 'NONE', #25145 ) ;
#5356=CARTESIAN_POINT ( 'NONE',  ( 133.0312500000000568, -2.485281374238555774, -6.000000000000005329 ) ) ;
#5357=CARTESIAN_POINT ( 'NONE',  ( 134.1711002691896510, 4.999999999999989342, 2.071067811865468400 ) ) ;
#5358=ORIENTED_EDGE ( 'NONE', *, *, #2216, .T. ) ;
#5362=B_SPLINE_CURVE_WITH_KNOTS ( 'NONE', 3,
 ( #3599, #17785, #29095, #3297, #8054, #12723, #22061, #24494, #5748, #1302 ),
 .UNSPECIFIED., .F., .F.,
 ( 4, 2, 2, 2, 4 ),
 ( 0.000000000000000000, 0.0005886548318705546240, 0.0008829822478058313396, 0.001030145955773469806, 0.001177309663741108164 ),
 .UNSPECIFIED. ) ;
#5363=EDGE_LOOP ( 'NONE', ( #27193, #19442, #20201, #1947 ) ) ;
#5365=CARTESIAN_POINT ( 'NONE',  ( 1.000000004113038354, -16.31584838240407720, -6.338213517867180791 ) ) ;
#5366=B_SPLINE_CURVE_WITH_KNOTS ( 'NONE', 3,
 ( #25247, #27549, #13484, #8250, #1044, #10285, #17366, #3338, #11167, #12918 ),
 .UNSPECIFIED., .F., .F.,
 ( 4, 2, 2, 2, 4 ),
 ( 0.000000000000000000, 0.0002749695263473663160, 0.0005499390526947326319, 0.001099878105389496489, 0.002199756210779025070 ),
 .UNSPECIFIED. ) ;
#5367=CARTESIAN_POINT ( 'NONE',  ( 137.0476497308104058, 0.000000000000000000, -5.000000000000004441 ) ) ;
#5368=DIRECTION ( 'NONE',  ( -1.000000000000000000, -0.000000000000000000, -0.000000000000000000 ) ) ;
#5375=FACE_OUTER_BOUND ( 'NONE', #12474, .T. ) ;
#5378=EDGE_CURVE ( 'NONE', #2984, #9337, #13230, .T. ) ;
#5382=EDGE_CURVE ( 'NONE', #14866, #25911, #18074, .T. ) ;
#5384=VERTEX_POINT ( 'NONE', #15535 ) ;
#5389=CARTESIAN_POINT ( 'NONE',  ( 135.0000000000000284, 5.961779907188299532, -0.5849724307333836748 ) ) ;
#5390=CARTESIAN_POINT ( 'NONE',  ( 157.4136751345948539, 0.000000000000000000, -5.500000000000005329 ) ) ;
#5392=CARTESIAN_POINT ( 'NONE',  ( 140.4088296780374492, -11.40882967803873171, 4.170790813163523403 ) ) ;
#5397=CARTESIAN_POINT ( 'NONE',  ( 161.0000000000000284, -11.67610212985248452, 2.769230769230773603 ) ) ;
#5406=CARTESIAN_POINT ( 'NONE',  ( 140.4784473477112670, -9.424512066737543492, 7.429532019273854537 ) ) ;
#5409=AXIS2_PLACEMENT_3D ( 'NONE', #16009, #4987, #9775 ) ;
#5411=CARTESIAN_POINT ( 'NONE',  ( 145.3988248654052313, 3.889087296526011706, 3.889087296526011706 ) ) ;
#5413=EDGE_CURVE ( 'NONE', #13346, #20809, #5158, .T. ) ;
#5414=( NAMED_UNIT ( * ) PLANE_ANGLE_UNIT ( ) SI_UNIT ( $, .RADIAN. ) );
#5416=CARTESIAN_POINT ( 'NONE',  ( 144.4836002691896795, 4.999999999999989342, -2.071067811865468400 ) ) ;
#5417=CARTESIAN_POINT ( 'NONE',  ( 152.2500000000000284, -6.000000000000005329, 0.000000000000000000 ) ) ;
#5424=CARTESIAN_POINT ( 'NONE',  ( 144.2812500000000284, 2.485281374238585972, 6.000000000000005329 ) ) ;
#5428=ORIENTED_EDGE ( 'NONE', *, *, #24962, .T. ) ;
#5431=AXIS2_PLACEMENT_3D ( 'NONE', #5347, #23964, #18926 ) ;
#5436=CARTESIAN_POINT ( 'NONE',  ( 116.0000000000000142, 0.000000000000000000, 0.000000000000000000 ) ) ;
#5437=CARTESIAN_POINT ( 'NONE',  ( 140.1363996827915059, -11.13639968279144910, 4.472640761300569423 ) ) ;
#5439=CARTESIAN_POINT ( 'NONE',  ( -19.99999999999998224, -54.99999999999990763, -7.500000000000007105 ) ) ;
#5441=CARTESIAN_POINT ( 'NONE',  ( 135.0000000000000000, 5.732128757725034163, 1.428824620004477630 ) ) ;
#5443=DIRECTION ( 'NONE',  ( -1.000000000000000000, 3.469446951953694061E-16, 0.000000000000000000 ) ) ;
#5452=CYLINDRICAL_SURFACE ( 'NONE', #26850, 5.500000000000000000 ) ;
#5455=CARTESIAN_POINT ( 'NONE',  ( 161.2500000000000284, -6.000000000000005329, 0.000000000000000000 ) ) ;
#5459=ORIENTED_EDGE ( 'NONE', *, *, #18431, .F. ) ;
#5469=CIRCLE ( 'NONE', #25605, 0.9999999999999993339 ) ;
#5471=EDGE_CURVE ( 'NONE', #7029, #9852, #28313, .T. ) ;
#5477=SURFACE_STYLE_USAGE ( .BOTH. , #10122 ) ;
#5480=CARTESIAN_POINT ( 'NONE',  ( 152.7113248654052313, 5.500000000000005329, 0.000000000000000000 ) ) ;
#5482=CARTESIAN_POINT ( 'NONE',  ( 140.5000000000000284, -11.45643923738959202, -5.000000000000004441 ) ) ;
#5485=CARTESIAN_POINT ( 'NONE',  ( 0.000000000000000000, -10.00000000000000888, -8.500000000000007105 ) ) ;
#5486=EDGE_CURVE ( 'NONE', #9495, #7022, #15103, .T. ) ;
#5490=ORIENTED_EDGE ( 'NONE', *, *, #10200, .T. ) ;
#5499=CARTESIAN_POINT ( 'NONE',  ( 159.7500000000000284, -6.000000000000005329, 0.000000000000000000 ) ) ;
#5502=ORIENTED_EDGE ( 'NONE', *, *, #24632, .F. ) ;
#5503=CARTESIAN_POINT ( 'NONE',  ( -0.5000000000000004441, -14.50000000000001243, -7.500000000000007105 ) ) ;
#5506=DIRECTION ( 'NONE',  ( 1.000000000000000000, -3.469446951953694061E-16, 0.000000000000000000 ) ) ;
#5512=CARTESIAN_POINT ( 'NONE',  ( 149.9136751345948539, 0.000000000000000000, -5.500000000000005329 ) ) ;
#5515=CARTESIAN_POINT ( 'NONE',  ( 139.1101497308104342, 3.535533905932725318, 3.535533905932725318 ) ) ;
#5516=CARTESIAN_POINT ( 'NONE',  ( -4.999999999999990230, -24.99999999999999289, 7.500000000000007105 ) ) ;
#5517=DIRECTION ( 'NONE',  ( 1.000000000000000000, 0.000000000000000000, 0.000000000000000000 ) ) ;
#5521=EDGE_CURVE ( 'NONE', #17667, #11814, #19527, .T. ) ;
#5523=TOROIDAL_SURFACE ( 'NONE', #18815, 14.49999999999999822, 0.5000000000000000000 ) ;
#5525=CARTESIAN_POINT ( 'NONE',  ( 153.9449251345948539, -5.500000000000012434, 2.278174593052012309 ) ) ;
#5526=ORIENTED_EDGE ( 'NONE', *, *, #12260, .F. ) ;
#5531=VERTEX_POINT ( 'NONE', #17026 ) ;
#5533=CARTESIAN_POINT ( 'NONE',  ( 136.9687500000000284, -2.485281374238585972, 6.000000000000005329 ) ) ;
#5543=EDGE_LOOP ( 'NONE', ( #2541, #26500, #2838, #7618 ) ) ;
#5544=CARTESIAN_POINT ( 'NONE',  ( 124.9999999999999432, -69.50000000000000000, -8.000000000000007105 ) ) ;
#5546=ADVANCED_FACE ( 'NONE', ( #9793 ), #5452, .F. ) ;
#5551=CARTESIAN_POINT ( 'NONE',  ( 156.9226497308104058, 5.000000000000004441, 0.000000000000000000 ) ) ;
#5554=CARTESIAN_POINT ( 'NONE',  ( 134.9999999999952536, -7.159935056834823008, 8.454462315789898597 ) ) ;
#5555=EDGE_CURVE ( 'NONE', #15347, #23700, #25107, .T. ) ;
#5563=( LENGTH_UNIT ( ) NAMED_UNIT ( * ) SI_UNIT ( .MILLI., .METRE. ) );
#5565=CARTESIAN_POINT ( 'NONE',  ( 138.6711002691896510, 4.999999999999989342, 2.071067811865468400 ) ) ;
#5566=CARTESIAN_POINT ( 'NONE',  ( 151.5000000000000284, 6.000000000000005329, 0.000000000000000000 ) ) ;
#5569=ORIENTED_EDGE ( 'NONE', *, *, #28138, .T. ) ;
#5570=CARTESIAN_POINT ( 'NONE',  ( 141.6562500000000284, -6.000000000000005329, 2.485281374238555774 ) ) ;
#5571=CARTESIAN_POINT ( 'NONE',  ( 142.5863248654052313, 0.000000000000000000, 5.500000000000005329 ) ) ;
#5572=DIRECTION ( 'NONE',  ( 1.000000000000000000, 0.000000000000000000, -0.000000000000000000 ) ) ;
#5580=EDGE_CURVE ( 'NONE', #9387, #24844, #6225, .T. ) ;
#5583=FILL_AREA_STYLE_COLOUR ( '', #28917 ) ;
#5587=CIRCLE ( 'NONE', #17413, 14.99999999999998579 ) ;
#5589=CARTESIAN_POINT ( 'NONE',  ( 144.8363248654052029, 0.000000000000000000, -5.500000000000005329 ) ) ;
#5592=CARTESIAN_POINT ( 'NONE',  ( 149.1488248654052029, -3.889087296526011706, -3.889087296526011706 ) ) ;
#5598=CARTESIAN_POINT ( 'NONE',  ( 153.0148502691896510, -3.535533905932725318, -3.535533905932725318 ) ) ;
#5605=CARTESIAN_POINT ( 'NONE',  ( 159.3750000000000568, 0.000000000000000000, 6.000000000000005329 ) ) ;
#5607=CARTESIAN_POINT ( 'NONE',  ( 145.9761751345948255, 3.889087296526011706, 3.889087296526011706 ) ) ;
#5611=ORIENTED_EDGE ( 'NONE', *, *, #17707, .T. ) ;
#5614=EDGE_CURVE ( 'NONE', #20028, #13346, #28130, .T. ) ;
#5623=CARTESIAN_POINT ( 'NONE',  ( 0.000000000000000000, -14.14213562373095634, -8.500000000000007105 ) ) ;
#5629=CARTESIAN_POINT ( 'NONE',  ( -0.04562205425674009662, -14.50000000000001243, 8.291335958003937634 ) ) ;
#5631=CARTESIAN_POINT ( 'NONE',  ( 154.8675748654052313, -5.500000000000012434, 2.278174593052012309 ) ) ;
#5635=CARTESIAN_POINT ( 'NONE',  ( 135.6334262937400013, -8.691027319329242218, 8.179640144927386558 ) ) ;
#5637=CARTESIAN_POINT ( 'NONE',  ( -1.000000000000000888, 10.00000000000000888, -4.000000000000003553 ) ) ;
#5638=AXIS2_PLACEMENT_3D ( 'NONE', #16043, #22617, #15424 ) ;
#5640=CARTESIAN_POINT ( 'NONE',  ( 148.7886751345948255, 5.500000000000005329, 0.000000000000000000 ) ) ;
#5645=EDGE_LOOP ( 'NONE', ( #15543, #29532, #5350 ) ) ;
#5646=MECHANICAL_DESIGN_GEOMETRIC_PRESENTATION_REPRESENTATION('',(#21389),#3696);
#5647=EDGE_CURVE ( 'NONE', #4838, #11174, #15800, .T. ) ;
#5650=PRESENTATION_STYLE_ASSIGNMENT (( #3193 ) ) ;
#5651=EDGE_LOOP ( 'NONE', ( #3875, #16494, #24039, #26726 ) ) ;
#5653=CARTESIAN_POINT ( 'NONE',  ( 161.3437500000000568, -6.000000000000005329, -2.485281374238555774 ) ) ;
#5654=EDGE_CURVE ( 'NONE', #5729, #4566, #8533, .T. ) ;
#5656=CIRCLE ( 'NONE', #13573, 9.999999999999980460 ) ;
#5658=DIRECTION ( 'NONE',  ( 1.000000000000000000, -0.000000000000000000, -0.000000000000000000 ) ) ;
#5664=CARTESIAN_POINT ( 'NONE',  ( 134.8913997308104342, -2.071067811865468400, 4.999999999999989342 ) ) ;
#5677=CARTESIAN_POINT ( 'NONE',  ( -39.99999999999998579, -59.99999999999980105, 3.000000000000002665 ) ) ;
#5678=LINE ( 'NONE', #9754, #22340 ) ;
#5681=CARTESIAN_POINT ( 'NONE',  ( 135.1875000000000568, 4.242640687119269671, 4.242640687119298093 ) ) ;
#5686=( BOUNDED_CURVE ( )  B_SPLINE_CURVE ( 2, ( #12640, #632, #9870, #5525, #16949, #19683, #7688, #28422, #12797 ),
 .UNSPECIFIED., .F., .T. ) 
 B_SPLINE_CURVE_WITH_KNOTS ( ( 3, 2, 2, 2, 3 ),
 ( 0.7124999999999992450, 0.7187499999999994449, 0.7249999999999996447, 0.7312499999999999556, 0.7375000000000002665 ),
 .UNSPECIFIED. ) 
 CURVE ( )  GEOMETRIC_REPRESENTATION_ITEM ( )  RATIONAL_B_SPLINE_CURVE ( ( 1.000000000000009548, 0.9238795325112773016, 1.000000000000000000, 0.9238795325112867385, 1.000000000000000000, 0.9238795325112867385, 1.000000000000000000, 0.9238795325112840739, 1.000000000000002665 ) ) 
 REPRESENTATION_ITEM ( '' )  );
#5687=CARTESIAN_POINT ( 'NONE',  ( 155.4449251345948255, -5.500000000000012434, 2.278174593052012309 ) ) ;
#5689=EDGE_LOOP ( 'NONE', ( #29303, #21241, #25951, #7152 ) ) ;
#5690=CARTESIAN_POINT ( 'NONE',  ( 141.0000000000000284, -12.00000000000001066, 4.000000000000003553 ) ) ;
#5694=ORIENTED_EDGE ( 'NONE', *, *, #12743, .T. ) ;
#5699=CARTESIAN_POINT ( 'NONE',  ( -4.999999999999990230, -24.99999999999999289, -5.000000000000004441 ) ) ;
#5703=CARTESIAN_POINT ( 'NONE',  ( 157.2038997308104058, 2.071067811865468400, 4.999999999999989342 ) ) ;
#5713=DIRECTION ( 'NONE',  ( 1.000000000000000000, 1.794541526872559254E-15, 0.000000000000000000 ) ) ;
#5715=CARTESIAN_POINT ( 'NONE',  ( 151.8750000000000284, 0.000000000000000000, 6.000000000000005329 ) ) ;
#5722=CARTESIAN_POINT ( 'NONE',  ( 145.8750000000000284, 0.000000000000000000, 6.000000000000005329 ) ) ;
#5723=CARTESIAN_POINT ( 'NONE',  ( 161.3386106984802097, -5.845894788924955954, 0.1212874700761470553 ) ) ;
#5724=COLOUR_RGB ( '', 0.09019608, 0.27058824, 0.51372549) ;
#5729=VERTEX_POINT ( 'NONE', #13932 ) ;
#5735=DIRECTION ( 'NONE',  ( -1.000000000000000000, -1.387778780781444413E-14, 0.000000000000000000 ) ) ;
#5737=CARTESIAN_POINT ( 'NONE',  ( 135.0000000000000284, -12.00000000000001066, 5.000000000000004441 ) ) ;
#5740=COLOUR_RGB ( '', 0.08235294, 0.09019608, 0.10196078) ;
#5745=FACE_OUTER_BOUND ( 'NONE', #2945, .T. ) ;
#5747=CARTESIAN_POINT ( 'NONE',  ( 150.1011751345948539, 3.889087296526011706, -3.889087296526011706 ) ) ;
#5748=CARTESIAN_POINT ( 'NONE',  ( 139.5500150635274963, -9.165151389911695645, -8.000000000000007105 ) ) ;
#5760=MECHANICAL_DESIGN_GEOMETRIC_PRESENTATION_REPRESENTATION('',(#20501),#12682);
#5767=EDGE_LOOP ( 'NONE', ( #10076, #17347, #26510, #3605, #22654 ) ) ;
#5771=CARTESIAN_POINT ( 'NONE',  ( 147.6636751345948255, 0.000000000000000000, 5.500000000000005329 ) ) ;
#5773=CARTESIAN_POINT ( 'NONE',  ( 124.9999999999999432, -65.00000000000000000, 7.500000000000007105 ) ) ;
#5776=DIRECTION ( 'NONE',  ( -1.000000000000000000, 0.000000000000000000, 0.000000000000000000 ) ) ;
#5780=CARTESIAN_POINT ( 'NONE',  ( -9.757819552369539906E-16, -9.500000000000008882, 5.000000000000004441 ) ) ;
#5783=FILL_AREA_STYLE_COLOUR ( '', #9016 ) ;
#5790=CARTESIAN_POINT ( 'NONE',  ( -4.999999999999886313, -9.000000000000007105, -5.000000000000004441 ) ) ;
#5797=CARTESIAN_POINT ( 'NONE',  ( 135.8257310488615133, -9.165151389911695645, 8.000000000000007105 ) ) ;
#5798=VERTEX_POINT ( 'NONE', #6508 ) ;
#5800=ORIENTED_EDGE ( 'NONE', *, *, #30256, .T. ) ;
#5802=CARTESIAN_POINT ( 'NONE',  ( 158.6250000000000568, 0.000000000000000000, -6.000000000000005329 ) ) ;
#5804=ORIENTED_EDGE ( 'NONE', *, *, #1779, .F. ) ;
#5811=CARTESIAN_POINT ( 'NONE',  ( 0.07037525868249273897, -16.32901554376975994, -6.302134984203353163 ) ) ;
#5813=DIRECTION ( 'NONE',  ( 1.000000000000000000, -0.000000000000000000, -0.000000000000000000 ) ) ;
#5822=CYLINDRICAL_SURFACE ( 'NONE', #17218, 0.5000000000000004441 ) ;
#5829=CIRCLE ( 'NONE', #25955, 11.00000000000000355 ) ;
#5834=EDGE_CURVE ( 'NONE', #11662, #18727, #29261, .T. ) ;
#5841=DIRECTION ( 'NONE',  ( -1.000000000000000000, -0.000000000000000000, 0.000000000000000000 ) ) ;
#5844=ORIENTED_EDGE ( 'NONE', *, *, #22214, .T. ) ;
#5845=CARTESIAN_POINT ( 'NONE',  ( 159.6346307794920563, -11.11465906960594552, 4.524012694217853792 ) ) ;
#5848=CARTESIAN_POINT ( 'NONE',  ( 140.6324251345948824, -5.500000000000012434, -2.278174593052012309 ) ) ;
#5849=CARTESIAN_POINT ( 'NONE',  ( -39.99999999999998579, -59.99999999999980105, 4.000000000000003553 ) ) ;
#5851=CARTESIAN_POINT ( 'NONE',  ( 150.6636751345948255, 0.000000000000000000, 5.500000000000005329 ) ) ;
#5852=AXIS2_PLACEMENT_3D ( 'NONE', #906, #2917, #17236 ) ;
#5853=CARTESIAN_POINT ( 'NONE',  ( 149.7038997308104058, 2.071067811865468400, 4.999999999999989342 ) ) ;
#5854=CARTESIAN_POINT ( 'NONE',  ( 129.9999999999998010, -89.00000000000001421, -3.000000000000002665 ) ) ;
#5858=( NAMED_UNIT ( * ) PLANE_ANGLE_UNIT ( ) SI_UNIT ( $, .RADIAN. ) );
#5862=ORIENTED_EDGE ( 'NONE', *, *, #5654, .F. ) ;
#5869=CARTESIAN_POINT ( 'NONE',  ( 144.0937500000000284, 6.000000000000005329, 2.485281374238585972 ) ) ;
#5870=CARTESIAN_POINT ( 'NONE',  ( 141.8511751345948255, -3.889087296526011706, 3.889087296526011706 ) ) ;
#5874=EDGE_LOOP ( 'NONE', ( #19766, #26472 ) ) ;
#5876=CARTESIAN_POINT ( 'NONE',  ( 146.3437500000000568, -6.000000000000005329, -2.485281374238555774 ) ) ;
#5877=CARTESIAN_POINT ( 'NONE',  ( 161.2383870809328528, -4.478016635995236250, 3.602319577417127050 ) ) ;
#5878=ORIENTED_EDGE ( 'NONE', *, *, #17363, .T. ) ;
#5899=CYLINDRICAL_SURFACE ( 'NONE', #15788, 5.500000000000000000 ) ;
#5900=ADVANCED_FACE ( 'NONE', ( #28589 ), #26295, .F. ) ;
#5904=CARTESIAN_POINT ( 'NONE',  ( 151.6949251345948255, 5.500000000000012434, -2.278174593052012309 ) ) ;
#5908=DIRECTION ( 'NONE',  ( -0.000000000000000000, -1.000000000000000000, 0.000000000000000000 ) ) ;
#5910=ORIENTED_EDGE ( 'NONE', *, *, #4807, .T. ) ;
#5911=CARTESIAN_POINT ( 'NONE',  ( 159.9375000000000284, -4.242640687119298093, -4.242640687119298093 ) ) ;
#5916=EDGE_LOOP ( 'NONE', ( #5968, #1938, #14192, #20015 ) ) ;
#5918=( GEOMETRIC_REPRESENTATION_CONTEXT ( 3 ) GLOBAL_UNCERTAINTY_ASSIGNED_CONTEXT ( ( #26215 ) ) GLOBAL_UNIT_ASSIGNED_CONTEXT ( ( #8737, #30223, #4575 ) ) REPRESENTATION_CONTEXT ( 'NONE', 'WORKASPACE' ) );
#5919=UNCERTAINTY_MEASURE_WITH_UNIT (LENGTH_MEASURE( 1.000000000000000082E-05 ), #21653, 'distance_accuracy_value', 'NONE');
#5920=VERTEX_POINT ( 'NONE', #5094 ) ;
#5927=AXIS2_PLACEMENT_3D ( 'NONE', #29176, #10634, #19983 ) ;
#5928=EDGE_CURVE ( 'NONE', #2252, #2328, #27800, .T. ) ;
#5933=DIRECTION ( 'NONE',  ( 1.000000000000000000, -0.000000000000000000, -0.000000000000000000 ) ) ;
#5935=CARTESIAN_POINT ( 'NONE',  ( 155.5238248654052313, 3.889087296526011706, -3.889087296526011706 ) ) ;
#5940=CARTESIAN_POINT ( 'NONE',  ( -1.000000000000002665, -9.000000000000007105, 4.000000000000005329 ) ) ;
#5943=DIRECTION ( 'NONE',  ( 1.000000000000000000, -0.000000000000000000, -0.000000000000000000 ) ) ;
#5947=CARTESIAN_POINT ( 'NONE',  ( 135.0000000000000284, -8.296337134229657906, 7.693139387096130655 ) ) ;
#5948=CIRCLE ( 'NONE', #21679, 28.99999999999999645 ) ;
#5951=CARTESIAN_POINT ( 'NONE',  ( 130.0000000000000284, -60.00000000000001421, -4.000000000000003553 ) ) ;
#5952=CARTESIAN_POINT ( 'NONE',  ( 161.2500000000000284, -6.000000000000005329, 0.000000000000000000 ) ) ;
#5963=CARTESIAN_POINT ( 'NONE',  ( 154.7812500000000568, 2.485281374238585972, 6.000000000000005329 ) ) ;
#5968=ORIENTED_EDGE ( 'NONE', *, *, #610, .T. ) ;
#5969=CARTESIAN_POINT ( 'NONE',  ( 151.1324251345948255, -5.500000000000012434, -2.278174593052012309 ) ) ;
#5971=DIRECTION ( 'NONE',  ( 0.000000000000000000, 0.000000000000000000, -1.000000000000000000 ) ) ;
#5973=CIRCLE ( 'NONE', #5004, 1.000000000000000888 ) ;
#5975=CARTESIAN_POINT ( 'NONE',  ( 116.0000000000000142, 0.000000000000000000, -5.500000000000000000 ) ) ;
#5979=CARTESIAN_POINT ( 'NONE',  ( 0.7669223171414771834, -15.58766199952933107, -7.954545454545431049 ) ) ;
#5981=DIRECTION ( 'NONE',  ( 0.000000000000000000, 0.000000000000000000, 1.000000000000000000 ) ) ;
#5983=CARTESIAN_POINT ( 'NONE',  ( 0.8032275580764794976, -15.44744712271809739, -8.223858897419269454 ) ) ;
#5987=CARTESIAN_POINT ( 'NONE',  ( -39.00000000000000000, -20.00000000000021316, -3.000000000000002665 ) ) ;
#5989=CARTESIAN_POINT ( 'NONE',  ( -9.999999999999994671, -9.000000000000007105, 4.000000000000003553 ) ) ;
#5990=LINE ( 'NONE', #8286, #19631 ) ;
#6006=CARTESIAN_POINT ( 'NONE',  ( 138.1949251345948255, 5.500000000000012434, -2.278174593052012309 ) ) ;
#6008=CARTESIAN_POINT ( 'NONE',  ( 139.9687500000000284, -2.485281374238585972, 6.000000000000005329 ) ) ;
#6010=CARTESIAN_POINT ( 'NONE',  ( 136.3050748654052882, 5.500000000000012434, 2.278174593052012309 ) ) ;
#6012=CARTESIAN_POINT ( 'NONE',  ( 136.9761751345948539, 3.889087296526011706, 3.889087296526011706 ) ) ;
#6018=VECTOR ( 'NONE', #4063, 1000.000000000000000 ) ;
#6019=CARTESIAN_POINT ( 'NONE',  ( 148.9538997308104342, -2.071067811865468400, -4.999999999999989342 ) ) ;
#6033=CARTESIAN_POINT ( 'NONE',  ( 143.6250000000000284, 0.000000000000000000, -6.000000000000005329 ) ) ;
#6034=FACE_OUTER_BOUND ( 'NONE', #27641, .T. ) ;
#6036=( NAMED_UNIT ( * ) PLANE_ANGLE_UNIT ( ) SI_UNIT ( $, .RADIAN. ) );
#6038=EDGE_LOOP ( 'NONE', ( #30235, #7805, #24541, #27449 ) ) ;
#6039=CARTESIAN_POINT ( 'NONE',  ( 145.6875000000000284, 4.242640687119269671, 4.242640687119298093 ) ) ;
#6040=CARTESIAN_POINT ( 'NONE',  ( 143.2425748654052313, -2.278174593052290753, -5.499999999999732658 ) ) ;
#6042=AXIS2_PLACEMENT_3D ( 'NONE', #1295, #22208, #19898 ) ;
#6044=EDGE_CURVE ( 'NONE', #12501, #19344, #852, .T. ) ;
#6051=EDGE_CURVE ( 'NONE', #19511, #3951, #6165, .T. ) ;
#6059=SHAPE_DEFINITION_REPRESENTATION ( #8682, #15661 ) ;
#6065=UNCERTAINTY_MEASURE_WITH_UNIT (LENGTH_MEASURE( 1.000000000000000082E-05 ), #12500, 'distance_accuracy_value', 'NONE');
#6069=CARTESIAN_POINT ( 'NONE',  ( 153.5773502691896510, 5.000000000000004441, 0.000000000000000000 ) ) ;
#6072=DIRECTION ( 'NONE',  ( 0.000000000000000000, 0.000000000000000000, -1.000000000000000000 ) ) ;
#6077=CARTESIAN_POINT ( 'NONE',  ( 159.7500000000000284, -6.000000000000005329, 0.000000000000000000 ) ) ;
#6078=CARTESIAN_POINT ( 'NONE',  ( -4.999999999999990230, -24.99999999999999289, 8.000000000000007105 ) ) ;
#6079=CARTESIAN_POINT ( 'NONE',  ( 145.4136751345948539, 0.000000000000000000, -5.500000000000005329 ) ) ;
#6081=EDGE_CURVE ( 'NONE', #4935, #25253, #2832, .T. ) ;
#6089=ADVANCED_FACE ( 'NONE', ( #940 ), #13156, .F. ) ;
#6095=ORIENTED_EDGE ( 'NONE', *, *, #18510, .T. ) ;
#6096=DIRECTION ( 'NONE',  ( 1.000000000000000000, -0.000000000000000000, -0.000000000000000000 ) ) ;
#6097=LINE ( 'NONE', #29429, #10922 ) ;
#6099=CARTESIAN_POINT ( 'NONE',  ( 0.9868033348211120437, -16.18260772123499081, -6.670819112052091882 ) ) ;
#6104=CARTESIAN_POINT ( 'NONE',  ( -0.05236263670367936190, -9.947637363296344404, 4.619711369386890532 ) ) ;
#6106=CARTESIAN_POINT ( 'NONE',  ( 160.2261751345948539, -3.889087296526011706, -3.889087296526011706 ) ) ;
#6109=CARTESIAN_POINT ( 'NONE',  ( 141.2886751345948539, 5.500000000000005329, 0.000000000000000000 ) ) ;
#6119=DIRECTION ( 'NONE',  ( 1.000000000000000000, -0.000000000000000000, -0.000000000000000000 ) ) ;
#6122=STYLED_ITEM ( 'NONE', ( #6220 ), #17033 ) ;
#6124=EDGE_LOOP ( 'NONE', ( #29773, #29411, #4613, #24956 ) ) ;
#6125=CARTESIAN_POINT ( 'NONE',  ( 155.7187500000000568, 2.485281374238555774, -6.000000000000005329 ) ) ;
#6126=VECTOR ( 'NONE', #22714, 1000.000000000000000 ) ;
#6130=VERTEX_POINT ( 'NONE', #171 ) ;
#6131=DIRECTION ( 'NONE',  ( 0.000000000000000000, 0.000000000000000000, -1.000000000000000000 ) ) ;
#6139=CARTESIAN_POINT ( 'NONE',  ( 160.5991965838383351, -11.35444276374069617, -3.884274201564634765 ) ) ;
#6142=CARTESIAN_POINT ( 'NONE',  ( 0.8631338372297875372, -15.37878787878789133, -8.351220472436782671 ) ) ;
#6148=CARTESIAN_POINT ( 'NONE',  ( -4.999999999999990230, -55.00000000000002132, -5.000000000000004441 ) ) ;
#6153=AXIS2_PLACEMENT_3D ( 'NONE', #25413, #4534, #13490 ) ;
#6155=CYLINDRICAL_SURFACE ( 'NONE', #5927, 1.000000000000000000 ) ;
#6156=CARTESIAN_POINT ( 'NONE',  ( 142.1398502691896510, -3.535533905932752852, 3.535533905932725318 ) ) ;
#6163=CARTESIAN_POINT ( 'NONE',  ( 135.0000000000000284, 3.755552545897461236, -4.233421981095762732 ) ) ;
#6165=( BOUNDED_CURVE ( )  B_SPLINE_CURVE ( 2, ( #12975, #8152, #8476, #6175, #8011, #13129, #6012, #12521, #15267 ),
 .UNSPECIFIED., .F., .T. ) 
 B_SPLINE_CURVE_WITH_KNOTS ( ( 3, 2, 2, 2, 3 ),
 ( 0.1374999999999996780, 0.1437499999999995448, 0.1499999999999992728, 0.1562499999999990008, 0.1624999999999987566 ),
 .UNSPECIFIED. ) 
 CURVE ( )  GEOMETRIC_REPRESENTATION_ITEM ( )  RATIONAL_B_SPLINE_CURVE ( ( 1.000000000000003331, 0.9238795325112834078, 1.000000000000000000, 0.9238795325112867385, 1.000000000000000000, 0.9238795325112867385, 1.000000000000000000, 0.9238795325113016155, 0.9999999999999851230 ) ) 
 REPRESENTATION_ITEM ( '' )  );
#6168=CIRCLE ( 'NONE', #6653, 1.000000000000000888 ) ;
#6170=CARTESIAN_POINT ( 'NONE',  ( 137.9136751345948539, 0.000000000000000000, -5.500000000000005329 ) ) ;
#6171=CARTESIAN_POINT ( 'NONE',  ( 141.5625000000000284, -4.242640687119298093, 4.242640687119298093 ) ) ;
#6172=ORIENTED_EDGE ( 'NONE', *, *, #9983, .F. ) ;
#6175=CARTESIAN_POINT ( 'NONE',  ( 136.6949251345948255, 5.500000000000012434, -2.278174593052012309 ) ) ;
#6179=CARTESIAN_POINT ( 'NONE',  ( 147.6413997308104058, 2.071067811865468400, -4.999999999999989342 ) ) ;
#6187=( GEOMETRIC_REPRESENTATION_CONTEXT ( 3 ) GLOBAL_UNCERTAINTY_ASSIGNED_CONTEXT ( ( #16752 ) ) GLOBAL_UNIT_ASSIGNED_CONTEXT ( ( #17509, #20096, #22250 ) ) REPRESENTATION_CONTEXT ( 'NONE', 'WORKASPACE' ) );
#6190=CYLINDRICAL_SURFACE ( 'NONE', #23881, 0.5000000000000004441 ) ;
#6193=CARTESIAN_POINT ( 'NONE',  ( 146.2500000000000568, -6.000000000000005329, 0.000000000000000000 ) ) ;
#6194=TOROIDAL_SURFACE ( 'NONE', #1759, 1.000000000000000000, 0.5000000000000000000 ) ;
#6197=CARTESIAN_POINT ( 'NONE',  ( 137.6250000000000284, 0.000000000000000000, -6.000000000000005329 ) ) ;
#6198=CARTESIAN_POINT ( 'NONE',  ( 161.1892173070653200, -3.029880711177796115, 4.825706568618548964 ) ) ;
#6210=DIRECTION ( 'NONE',  ( 0.3742395684072007955, 0.4425345409093102700, 0.8149281720130788775 ) ) ;
#6217=PRODUCT ( 'Fixed Jaw', 'Fixed Jaw', '', ( #4206 ) ) ;
#6219=TOROIDAL_SURFACE ( 'NONE', #7686, 11.00000000000000355, 1.000000000000000000 ) ;
#6220=PRESENTATION_STYLE_ASSIGNMENT (( #25403 ) ) ;
#6222=CARTESIAN_POINT ( 'NONE',  ( 116.0000000000000142, 6.735557395310442023E-16, 5.500000000000000000 ) ) ;
#6225=LINE ( 'NONE', #18235, #19065 ) ;
#6227=EDGE_CURVE ( 'NONE', #15395, #28093, #10429, .T. ) ;
#6229=CARTESIAN_POINT ( 'NONE',  ( 156.7500000000000284, -6.000000000000005329, 0.000000000000000000 ) ) ;
#6232=VERTEX_POINT ( 'NONE', #7672 ) ;
#6233=CIRCLE ( 'NONE', #18054, 11.00000000000000355 ) ;
#6234=ORIENTED_EDGE ( 'NONE', *, *, #6051, .T. ) ;
#6237=( BOUNDED_CURVE ( )  B_SPLINE_CURVE ( 2, ( #23203, #4589, #23654, #11552, #20894, #28076, #14015, #21343, #23358 ),
 .UNSPECIFIED., .F., .T. ) 
 B_SPLINE_CURVE_WITH_KNOTS ( ( 3, 2, 2, 2, 3 ),
 ( 0.6875000000000002220, 0.6937499999999999778, 0.6999999999999997335, 0.7062499999999994893, 0.7124999999999992450 ),
 .UNSPECIFIED. ) 
 CURVE ( )  GEOMETRIC_REPRESENTATION_ITEM ( )  RATIONAL_B_SPLINE_CURVE ( ( 0.9999999999999973355, 0.9238795325112894030, 1.000000000000000000, 0.9238795325112867385, 1.000000000000000000, 0.9238795325112867385, 1.000000000000000000, 0.9238795325112961754, 0.9999999999999905631 ) ) 
 REPRESENTATION_ITEM ( '' )  );
#6241=CARTESIAN_POINT ( 'NONE',  ( -1.000000000000000888, -9.000000000000007105, -4.000000000000003553 ) ) ;
#6246=AXIS2_PLACEMENT_3D ( 'NONE', #5503, #29002, #9999 ) ;
#6248=CIRCLE ( 'NONE', #22455, 1.000000000000000888 ) ;
#6251=CARTESIAN_POINT ( 'NONE',  ( 140.5384615384615756, -11.07692307692306777, 4.615384615384604317 ) ) ;
#6258=EDGE_LOOP ( 'NONE', ( #22547, #14035, #21215, #15731 ) ) ;
#6267=CARTESIAN_POINT ( 'NONE',  ( 149.5238248654052313, 3.889087296526011706, -3.889087296526011706 ) ) ;
#6268=ORIENTED_EDGE ( 'NONE', *, *, #11622, .F. ) ;
#6272=CARTESIAN_POINT ( 'NONE',  ( 153.6562500000000568, -6.000000000000005329, 2.485281374238555774 ) ) ;
#6276=CARTESIAN_POINT ( 'NONE',  ( 157.0238248654052313, 3.889087296526011706, -3.889087296526011706 ) ) ;
#6280=DIRECTION ( 'NONE',  ( -1.000000000000000000, 0.000000000000000000, 0.000000000000000000 ) ) ;
#6283=CARTESIAN_POINT ( 'NONE',  ( -9.999999999999793943, 10.00000000000000888, 4.000000000000003553 ) ) ;
#6284=CARTESIAN_POINT ( 'NONE',  ( 139.9613248654052313, -5.500000000000005329, 0.000000000000000000 ) ) ;
#6289=DIRECTION ( 'NONE',  ( 6.938893903907222067E-15, 1.000000000000000000, 0.000000000000000000 ) ) ;
#6296=CARTESIAN_POINT ( 'NONE',  ( 124.9999999999999432, -70.00000000000000000, 8.000000000000007105 ) ) ;
#6301=EDGE_CURVE ( 'NONE', #1053, #17791, #7817, .T. ) ;
#6302=CARTESIAN_POINT ( 'NONE',  ( 142.6086002691896226, -2.071067811865468400, -4.999999999999989342 ) ) ;
#6303=ORIENTED_EDGE ( 'NONE', *, *, #22118, .F. ) ;
#6306=CARTESIAN_POINT ( 'NONE',  ( 135.0000000000000568, 5.527055845544526669, -1.966580164914623952 ) ) ;
#6308=ORIENTED_EDGE ( 'NONE', *, *, #17222, .T. ) ;
#6310=CARTESIAN_POINT ( 'NONE',  ( 140.2500000000000284, -6.000000000000005329, 0.000000000000000000 ) ) ;
#6311=VERTEX_POINT ( 'NONE', #12625 ) ;
#6313=CARTESIAN_POINT ( 'NONE',  ( -4.999999999999990230, -24.99999999999999289, -8.000000000000007105 ) ) ;
#6318=CARTESIAN_POINT ( 'NONE',  ( 152.7976497308104058, 0.000000000000000000, 5.000000000000004441 ) ) ;
#6322=EDGE_CURVE ( 'NONE', #25961, #13568, #2313, .T. ) ;
#6324=ADVANCED_FACE ( 'NONE', ( #13244 ), #20278, .T. ) ;
#6328=VERTEX_POINT ( 'NONE', #16008 ) ;
#6331=DIRECTION ( 'NONE',  ( 0.000000000000000000, 0.000000000000000000, -1.000000000000000000 ) ) ;
#6333=ORIENTED_EDGE ( 'NONE', *, *, #7383, .T. ) ;
#6334=CARTESIAN_POINT ( 'NONE',  ( 143.7187500000000284, 2.485281374238556218, -6.000000000000005329 ) ) ;
#6335=CARTESIAN_POINT ( 'NONE',  ( 141.6636751345948255, 0.000000000000000000, 5.500000000000005329 ) ) ;
#6336=DIRECTION ( 'NONE',  ( 1.000000000000000000, 1.067522139062651904E-16, -0.000000000000000000 ) ) ;
#6337=CARTESIAN_POINT ( 'NONE',  ( 140.1562500000000853, -6.000000000000005329, 2.485281374238555774 ) ) ;
#6338=DIRECTION ( 'NONE',  ( 1.000000000000000000, 0.000000000000000000, 0.000000000000000000 ) ) ;
#6339=VERTEX_POINT ( 'NONE', #29467 ) ;
#6343=VERTEX_POINT ( 'NONE', #18141 ) ;
#6347=ORIENTED_EDGE ( 'NONE', *, *, #25651, .T. ) ;
#6349=( NAMED_UNIT ( * ) PLANE_ANGLE_UNIT ( ) SI_UNIT ( $, .RADIAN. ) );
#6354=ADVANCED_FACE ( 'NONE', ( #11071 ), #20418, .F. ) ;
#6356=CARTESIAN_POINT ( 'NONE',  ( 139.5000000000000284, -8.798545334315209132, -8.160000000000007248 ) ) ;
#6358=AXIS2_PLACEMENT_3D ( 'NONE', #12044, #2916, #14051 ) ;
#6363=CARTESIAN_POINT ( 'NONE',  ( 148.4211002691896226, -4.999999999999989342, -2.071067811865468400 ) ) ;
#6366=CARTESIAN_POINT ( 'NONE',  ( 135.5000000000000284, -8.500000000000007105, -7.500000000000007105 ) ) ;
#6369=CARTESIAN_POINT ( 'NONE',  ( 138.6636751345948255, 0.000000000000000000, 5.500000000000005329 ) ) ;
#6370=CARTESIAN_POINT ( 'NONE',  ( 150.0863248654052313, 0.000000000000000000, 5.500000000000005329 ) ) ;
#6373=CARTESIAN_POINT ( 'NONE',  ( 155.6250000000000284, 0.000000000000000000, -6.000000000000005329 ) ) ;
#6377=ORIENTED_EDGE ( 'NONE', *, *, #25421, .F. ) ;
#6378=ORIENTED_EDGE ( 'NONE', *, *, #25394, .T. ) ;
#6379=ADVANCED_FACE ( 'NONE', ( #10929 ), #17579, .F. ) ;
#6385=CIRCLE ( 'NONE', #10336, 14.99999999999998579 ) ;
#6386=CARTESIAN_POINT ( 'NONE',  ( 0.7560853098879504186, -15.51667758746989989, 8.092232509380407279 ) ) ;
#6387=( NAMED_UNIT ( * ) SI_UNIT ( $, .STERADIAN. ) SOLID_ANGLE_UNIT ( ) );
#6388=ORIENTED_EDGE ( 'NONE', *, *, #18893, .T. ) ;
#6390=DIRECTION ( 'NONE',  ( 0.000000000000000000, -1.000000000000000000, 0.000000000000000000 ) ) ;
#6397=CARTESIAN_POINT ( 'NONE',  ( 160.1324251345948255, -5.500000000000012434, -2.278174593052012309 ) ) ;
#6407=ORIENTED_EDGE ( 'NONE', *, *, #7034, .F. ) ;
#6410=CARTESIAN_POINT ( 'NONE',  ( 116.0000000000000142, 6.735557395310442023E-16, 5.500000000000000000 ) ) ;
#6417=CARTESIAN_POINT ( 'NONE',  ( 158.5312500000000284, -2.485281374238555774, -6.000000000000005329 ) ) ;
#6421=VERTEX_POINT ( 'NONE', #22227 ) ;
#6425=CARTESIAN_POINT ( 'NONE',  ( 159.1341896120059687, -12.00570085348640603, 3.993189331442730250 ) ) ;
#6427=CIRCLE ( 'NONE', #15281, 15.00000000000000000 ) ;
#6428=ORIENTED_EDGE ( 'NONE', *, *, #7414, .F. ) ;
#6431=DIRECTION ( 'NONE',  ( 0.000000000000000000, 0.000000000000000000, 1.000000000000000000 ) ) ;
#6434=DIRECTION ( 'NONE',  ( 1.000000000000000000, 0.000000000000000000, 0.000000000000000000 ) ) ;
#6444=DIRECTION ( 'NONE',  ( -0.000000000000000000, -1.000000000000000000, -0.000000000000000000 ) ) ;
#6451=CARTESIAN_POINT ( 'NONE',  ( 124.9999999999999432, -65.50000000000000000, -7.500000000000007105 ) ) ;
#6453=CARTESIAN_POINT ( 'NONE',  ( 140.6398502691896510, -3.535533905932752852, 3.535533905932725318 ) ) ;
#6454=CARTESIAN_POINT ( 'NONE',  ( -4.999999999999984013, -65.50000000000001421, 7.500000000000007105 ) ) ;
#6461=CARTESIAN_POINT ( 'NONE',  ( 135.0000000000000000, 1.949781249179272091, -5.142796231657337458 ) ) ;
#6465=CARTESIAN_POINT ( 'NONE',  ( 138.2886751345948539, 5.500000000000005329, 0.000000000000000000 ) ) ;
#6466=CARTESIAN_POINT ( 'NONE',  ( 143.7187500000000284, 2.485281374238555774, -6.000000000000005329 ) ) ;
#6470=ORIENTED_EDGE ( 'NONE', *, *, #16069, .F. ) ;
#6472=CARTESIAN_POINT ( 'NONE',  ( -1.000000000000000888, 9.000000000000007105, 3.000000000000002665 ) ) ;
#6473=SURFACE_SIDE_STYLE ('',( #13739 ) ) ;
#6477=EDGE_CURVE ( 'NONE', #3318, #9839, #10884, .T. ) ;
#6481=CARTESIAN_POINT ( 'NONE',  ( 151.4851497308104342, -3.535533905932725318, 3.535533905932725318 ) ) ;
#6485=FACE_OUTER_BOUND ( 'NONE', #28227, .T. ) ;
#6490=ORIENTED_EDGE ( 'NONE', *, *, #8809, .T. ) ;
#6494=DIRECTION ( 'NONE',  ( 0.000000000000000000, 1.000000000000000000, 0.000000000000000000 ) ) ;
#6497=CARTESIAN_POINT ( 'NONE',  ( 146.5312500000000284, -2.485281374238556218, -6.000000000000005329 ) ) ;
#6498=CARTESIAN_POINT ( 'NONE',  ( 160.0296263098200313, -11.64871681939485093, -2.884697388352327252 ) ) ;
#6499=SURFACE_STYLE_FILL_AREA ( #10680 ) ;
#6500=CARTESIAN_POINT ( 'NONE',  ( 137.9062500000000568, 6.000000000000005329, -2.485281374238555774 ) ) ;
#6501=CARTESIAN_POINT ( 'NONE',  ( -14.99999999999999289, -54.99999999999990763, 8.000000000000007105 ) ) ;
#6508=CARTESIAN_POINT ( 'NONE',  ( -0.07769256095283699759, -15.23231281889969679, -7.500000000000007105 ) ) ;
#6517=CARTESIAN_POINT ( 'NONE',  ( 139.5000000000000000, -8.798545334315230448, 8.160000000000007248 ) ) ;
#6520=CARTESIAN_POINT ( 'NONE',  ( 148.4136751345948539, 0.000000000000000000, -5.500000000000005329 ) ) ;
#6523=CARTESIAN_POINT ( 'NONE',  ( 150.1086002691896510, -2.071067811865468400, -4.999999999999989342 ) ) ;
#6524=CARTESIAN_POINT ( 'NONE',  ( 116.0000000000000142, 0.000000000000000000, -5.500000000000000000 ) ) ;
#6528=CYLINDRICAL_SURFACE ( 'NONE', #15904, 5.500000000000000000 ) ;
#6530=DIRECTION ( 'NONE',  ( -1.000000000000000000, -0.000000000000000000, -0.000000000000000000 ) ) ;
#6531=PRODUCT_DEFINITION_FORMATION_WITH_SPECIFIED_SOURCE ( 'ANY', '', #6217, .NOT_KNOWN. ) ;
#6533=CARTESIAN_POINT ( 'NONE',  ( 157.6875000000000284, 4.242640687119269671, 4.242640687119298093 ) ) ;
#6537=ORIENTED_EDGE ( 'NONE', *, *, #12008, .T. ) ;
#6538=EDGE_LOOP ( 'NONE', ( #29998, #2210, #9833, #22490 ) ) ;
#6540=ORIENTED_EDGE ( 'NONE', *, *, #12614, .T. ) ;
#6544=ORIENTED_EDGE ( 'NONE', *, *, #3538, .T. ) ;
#6545=FILL_AREA_STYLE ('',( #29591 ) ) ;
#6546=STYLED_ITEM ( 'NONE', ( #19783 ), #10017 ) ;
#6550=ORIENTED_EDGE ( 'NONE', *, *, #21919, .F. ) ;
#6553=CARTESIAN_POINT ( 'NONE',  ( 140.4121221836153950, -9.236957375441377849, 7.663966194509516328 ) ) ;
#6561=CARTESIAN_POINT ( 'NONE',  ( 0.2138740463844765738, -15.56974731274248391, 7.989747270033618953 ) ) ;
#6562=EDGE_LOOP ( 'NONE', ( #4466, #20532, #25146, #24103 ) ) ;
#6567=FACE_OUTER_BOUND ( 'NONE', #10284, .T. ) ;
#6569=SURFACE_STYLE_FILL_AREA ( #29612 ) ;
#6577=CARTESIAN_POINT ( 'NONE',  ( 150.8437500000000284, -6.000000000000005329, -2.485281374238555774 ) ) ;
#6582=ORIENTED_EDGE ( 'NONE', *, *, #29523, .F. ) ;
#6583=DIRECTION ( 'NONE',  ( -1.000000000000000000, -1.734723475976843579E-16, 0.000000000000000000 ) ) ;
#6586=CARTESIAN_POINT ( 'NONE',  ( 159.5122198478899804, -12.10635047839714673, 3.869002046573032150 ) ) ;
#6591=FACE_OUTER_BOUND ( 'NONE', #21523, .T. ) ;
#6609=DIRECTION ( 'NONE',  ( 0.000000000000000000, -1.000000000000000000, 0.000000000000000000 ) ) ;
#6610=CARTESIAN_POINT ( 'NONE',  ( 140.5461002691896510, -2.071067811865468400, 4.999999999999989342 ) ) ;
#6612=ORIENTED_EDGE ( 'NONE', *, *, #18715, .F. ) ;
#6618=EDGE_CURVE ( 'NONE', #11567, #13346, #14657, .T. ) ;
#6622=CARTESIAN_POINT ( 'NONE',  ( 143.4375000000000284, -4.242640687119298093, -4.242640687119298093 ) ) ;
#6623=ORIENTED_EDGE ( 'NONE', *, *, #26599, .T. ) ;
#6624=STYLED_ITEM ( 'NONE', ( #18725 ), #7544 ) ;
#6626=VERTEX_POINT ( 'NONE', #18817 ) ;
#6629=CYLINDRICAL_SURFACE ( 'NONE', #8825, 14.99999999999998579 ) ;
#6632=CARTESIAN_POINT ( 'NONE',  ( 143.4226497308104342, 5.000000000000004441, 0.000000000000000000 ) ) ;
#6634=DIRECTION ( 'NONE',  ( 1.000000000000000000, 0.000000000000000000, 0.000000000000000000 ) ) ;
#6638=PLANE ( 'NONE',  #11143 ) ;
#6641=LINE ( 'NONE', #11119, #3953 ) ;
#6645=DIRECTION ( 'NONE',  ( 0.000000000000000000, 0.000000000000000000, -1.000000000000000000 ) ) ;
#6651=DIRECTION ( 'NONE',  ( -1.000000000000000000, -1.067522139062651904E-16, 0.000000000000000000 ) ) ;
#6653=AXIS2_PLACEMENT_3D ( 'NONE', #9838, #10446, #896 ) ;
#6655=CARTESIAN_POINT ( 'NONE',  ( 140.9062500000000284, 6.000000000000005329, -2.485281374238556218 ) ) ;
#6657=FACE_OUTER_BOUND ( 'NONE', #21146, .T. ) ;
#6659=EDGE_CURVE ( 'NONE', #13568, #11692, #23601, .T. ) ;
#6660=CARTESIAN_POINT ( 'NONE',  ( 141.0000000000000284, 6.000000000000005329, 0.000000000000000000 ) ) ;
#6661=DIRECTION ( 'NONE',  ( 0.000000000000000000, 0.000000000000000000, 1.000000000000000000 ) ) ;
#6673=CARTESIAN_POINT ( 'NONE',  ( -0.5000000000000004441, -10.00000000000000888, -7.500000000000007105 ) ) ;
#6675=CARTESIAN_POINT ( 'NONE',  ( -0.7481905315629638897, -9.503618936874122625, 4.126213593628786924 ) ) ;
#6677=EDGE_CURVE ( 'NONE', #25878, #1389, #27139, .T. ) ;
#6679=SURFACE_SIDE_STYLE ('',( #29863 ) ) ;
#6682=CARTESIAN_POINT ( 'NONE',  ( 160.8675748654052029, -5.500000000000012434, 2.278174593052012309 ) ) ;
#6690=CYLINDRICAL_SURFACE ( 'NONE', #7624, 5.500000000000000000 ) ;
#6691=ORIENTED_EDGE ( 'NONE', *, *, #12855, .T. ) ;
#6692=CARTESIAN_POINT ( 'NONE',  ( 157.1250000000000284, 0.000000000000000000, -6.000000000000005329 ) ) ;
#6703=( NAMED_UNIT ( * ) PLANE_ANGLE_UNIT ( ) SI_UNIT ( $, .RADIAN. ) );
#6704=CARTESIAN_POINT ( 'NONE',  ( 0.8033614493835260495, -15.44729320518831805, 8.224148781931267749 ) ) ;
#6716=CARTESIAN_POINT ( 'NONE',  ( 145.7738248654052313, -3.889087296526011706, 3.889087296526011706 ) ) ;
#6720=CARTESIAN_POINT ( 'NONE',  ( 162.4836002691897079, 4.999999999999989342, -2.071067811865468400 ) ) ;
#6721=CARTESIAN_POINT ( 'NONE',  ( 135.0000000000000284, -7.706858840103492092, 8.197103070889301790 ) ) ;
#6725=DIRECTION ( 'NONE',  ( -0.000000000000000000, -0.000000000000000000, -1.000000000000000000 ) ) ;
#6727=FILL_AREA_STYLE_COLOUR ( '', #19203 ) ;
#6730=DIRECTION ( 'NONE',  ( 1.000000000000000000, 0.000000000000000000, 0.000000000000000000 ) ) ;
#6731=CARTESIAN_POINT ( 'NONE',  ( 150.3750000000000284, 0.000000000000000000, 6.000000000000005329 ) ) ;
#6732=VERTEX_POINT ( 'NONE', #5544 ) ;
#6737=SURFACE_STYLE_FILL_AREA ( #28369 ) ;
#6740=VECTOR ( 'NONE', #14599, 1000.000000000000000 ) ;
#6742=SURFACE_STYLE_FILL_AREA ( #27764 ) ;
#6753=CARTESIAN_POINT ( 'NONE',  ( -0.6001665993698070967, -9.799666801260325855, -4.385453238887226490 ) ) ;
#6757=CARTESIAN_POINT ( 'NONE',  ( 135.0000000000000284, -8.852647312720215211, -7.500000050752666958 ) ) ;
#6759=EDGE_LOOP ( 'NONE', ( #11136, #27828, #27434, #15462, #5526 ) ) ;
#6761=CARTESIAN_POINT ( 'NONE',  ( -4.999999999999886313, -70.00000000000001421, 8.000000000000007105 ) ) ;
#6765=CARTESIAN_POINT ( 'NONE',  ( 150.9300748654052313, 2.278174593051795149, -5.500000000000228262 ) ) ;
#6774=CARTESIAN_POINT ( 'NONE',  ( 137.0625000000000284, -4.242640687119298093, 4.242640687119298093 ) ) ;
#6775=EDGE_LOOP ( 'NONE', ( #21520, #2262, #6792, #1009 ) ) ;
#6777=DIRECTION ( 'NONE',  ( 1.000000000000000000, 0.000000000000000000, 0.000000000000000000 ) ) ;
#6782=CARTESIAN_POINT ( 'NONE',  ( 145.3913997308104058, -2.071067811865468400, 4.999999999999989342 ) ) ;
#6788=ADVANCED_FACE ( 'NONE', ( #25506 ), #23886, .F. ) ;
#6792=ORIENTED_EDGE ( 'NONE', *, *, #23791, .F. ) ;
#6798=CARTESIAN_POINT ( 'NONE',  ( 138.3750000000000284, 0.000000000000000000, 6.000000000000005329 ) ) ;
#6802=CARTESIAN_POINT ( 'NONE',  ( 137.1562500000000284, -6.000000000000005329, 2.485281374238555774 ) ) ;
#6803=DIRECTION ( 'NONE',  ( -1.000000000000000000, 0.000000000000000000, 0.000000000000000000 ) ) ;
#6809=EDGE_CURVE ( 'NONE', #22830, #4838, #9171, .T. ) ;
#6815=CARTESIAN_POINT ( 'NONE',  ( 140.5828481527998974, -11.16569630559845017, -4.440052304731437083 ) ) ;
#6817=ADVANCED_FACE ( 'NONE', ( #13738 ), #29815, .F. ) ;
#6819=CARTESIAN_POINT ( 'NONE',  ( 139.6521270721804342, -8.798545340575019580, -8.159999993250346861 ) ) ;
#6827=CARTESIAN_POINT ( 'NONE',  ( 149.1711002691896795, 4.999999999999989342, 2.071067811865468400 ) ) ;
#6828=CARTESIAN_POINT ( 'NONE',  ( 160.6800748654052029, -2.278174593052130881, 5.499999999999894307 ) ) ;
#6830=CARTESIAN_POINT ( 'NONE',  ( 155.7187500000000568, 2.485281374238556218, -6.000000000000005329 ) ) ;
#6832=CARTESIAN_POINT ( 'NONE',  ( 140.5384615384615756, -11.07692307692306777, -4.615384615384604317 ) ) ;
#6833=( BOUNDED_SURFACE ( )  B_SPLINE_SURFACE ( 3, 2, ( 
 ( #9779, #7458, #17009 ),
 ( #17158, #16867, #26190 ),
 ( #26338, #23901, #5288 ),
 ( #26478, #5437, #24191 ) ),
 .UNSPECIFIED., .F., .F., .F. ) 
 B_SPLINE_SURFACE_WITH_KNOTS ( ( 4, 4 ),
 ( 3, 3 ),
 ( 0.000000000000000000, 0.0002125775066526910278 ),
 ( 0.000000000000000000, 1.000000000000000000 ),
 .UNSPECIFIED. ) 
 GEOMETRIC_REPRESENTATION_ITEM ( )  RATIONAL_B_SPLINE_SURFACE ( (
 ( 1.000000000000000000, 0.7071067811865475727, 1.000000000000000000),
 ( 1.000000000000000000, 0.7257758655053210273, 1.000000000000000000),
 ( 1.000000000000000000, 0.7424605758826430257, 1.000000000000000000),
 ( 1.000000000000000000, 0.7576044462920076272, 1.000000000000000000) ) ) 
 REPRESENTATION_ITEM ( '' )  SURFACE ( )  );
#6834=MECHANICAL_DESIGN_GEOMETRIC_PRESENTATION_REPRESENTATION('',(#9785),#12745);
#6840=CARTESIAN_POINT ( 'NONE',  ( 158.1562500000000284, -6.000000000000005329, 2.485281374238555774 ) ) ;
#6845=ORIENTED_EDGE ( 'NONE', *, *, #18471, .T. ) ;
#6846=EDGE_CURVE ( 'NONE', #25883, #16005, #10964, .T. ) ;
#6851=CARTESIAN_POINT ( 'NONE',  ( -0.5000000000000004441, -24.99999999999999289, 8.000000000000007105 ) ) ;
#6853=AXIS2_PLACEMENT_3D ( 'NONE', #17194, #14732, #14877 ) ;
#6854=ORIENTED_EDGE ( 'NONE', *, *, #15664, .T. ) ;
#6855=EDGE_CURVE ( 'NONE', #8188, #17667, #27651, .T. ) ;
#6856=CARTESIAN_POINT ( 'NONE',  ( 13.99999999999999822, 0.000000000000000000, -16.50000000000000355 ) ) ;
#6857=AXIS2_PLACEMENT_3D ( 'NONE', #13284, #22627, #15742 ) ;
#6863=( GEOMETRIC_REPRESENTATION_CONTEXT ( 3 ) GLOBAL_UNCERTAINTY_ASSIGNED_CONTEXT ( ( #8387 ) ) GLOBAL_UNIT_ASSIGNED_CONTEXT ( ( #22279, #15822, #6387 ) ) REPRESENTATION_CONTEXT ( 'NONE', 'WORKASPACE' ) );
#6864=CYLINDRICAL_SURFACE ( 'NONE', #14445, 5.500000000000000000 ) ;
#6868=CARTESIAN_POINT ( 'NONE',  ( 161.1711002691896795, 4.999999999999989342, 2.071067811865468400 ) ) ;
#6876=( BOUNDED_CURVE ( )  B_SPLINE_CURVE ( 2, ( #28400, #308, #23675, #7075, #28253, #6916, #11885, #16489, #4763 ),
 .UNSPECIFIED., .F., .T. ) 
 B_SPLINE_CURVE_WITH_KNOTS ( ( 3, 2, 2, 2, 3 ),
 ( 0.6875000000000002220, 0.6937500000000004219, 0.7000000000000006217, 0.7062500000000009326, 0.7125000000000011324 ),
 .UNSPECIFIED. ) 
 CURVE ( )  GEOMETRIC_REPRESENTATION_ITEM ( )  RATIONAL_B_SPLINE_CURVE ( ( 0.9999999999999973355, 0.9238795325112894030, 1.000000000000000000, 0.9238795325112867385, 1.000000000000000000, 0.9238795325112867385, 1.000000000000000000, 0.9238795325112731938, 1.000000000000013545 ) ) 
 REPRESENTATION_ITEM ( '' )  );
#6877=ORIENTED_EDGE ( 'NONE', *, *, #29535, .T. ) ;
#6880=CIRCLE ( 'NONE', #12320, 1.000000000000000444 ) ;
#6881=CARTESIAN_POINT ( 'NONE',  ( 149.4375000000000284, -4.242640687119298093, -4.242640687119298093 ) ) ;
#6882=AXIS2_PLACEMENT_3D ( 'NONE', #8130, #10164, #17245 ) ;
#6883=EDGE_LOOP ( 'NONE', ( #816, #17084, #14307, #5247 ) ) ;
#6884=ADVANCED_FACE ( 'NONE', ( #23081 ), #2319, .F. ) ;
#6887=EDGE_CURVE ( 'NONE', #24855, #10410, #12510, .T. ) ;
#6890=FILL_AREA_STYLE_COLOUR ( '', #25460 ) ;
#6894=ORIENTED_EDGE ( 'NONE', *, *, #8693, .F. ) ;
#6904=CARTESIAN_POINT ( 'NONE',  ( 160.7244614532509672, -11.41189565439133879, -3.712099293216823970 ) ) ;
#6911=DIRECTION ( 'NONE',  ( 1.000000000000000000, 0.000000000000000000, 0.000000000000000000 ) ) ;
#6912=VERTEX_POINT ( 'NONE', #26880 ) ;
#6915=FACE_BOUND ( 'NONE', #5874, .T. ) ;
#6916=CARTESIAN_POINT ( 'NONE',  ( 140.6175748654052313, 5.500000000000012434, -2.278174593052012309 ) ) ;
#6918=VERTEX_POINT ( 'NONE', #12655 ) ;
#6919=CARTESIAN_POINT ( 'NONE',  ( 152.1488248654052029, -3.889087296526011706, -3.889087296526011706 ) ) ;
#6921=CARTESIAN_POINT ( 'NONE',  ( 133.5937500000000284, 6.000000000000005329, 2.485281374238585972 ) ) ;
#6922=EDGE_CURVE ( 'NONE', #18576, #3582, #23845, .T. ) ;
#6923=EDGE_CURVE ( 'NONE', #6626, #9180, #4759, .T. ) ;
#6927=CARTESIAN_POINT ( 'NONE',  ( 142.4136751345948539, 0.000000000000000000, -5.500000000000005329 ) ) ;
#6931=CARTESIAN_POINT ( 'NONE',  ( 135.0000273856246622, -6.966962943893147298, -8.502862253537376347 ) ) ;
#6932=CARTESIAN_POINT ( 'NONE',  ( 143.5163997308104058, 4.999999999999989342, 2.071067811865468400 ) ) ;
#6934=COLOUR_RGB ( '', 0.09019608, 0.27058824, 0.51372549) ;
#6936=DIRECTION ( 'NONE',  ( -1.000000000000000000, 0.000000000000000000, 0.000000000000000000 ) ) ;
#6937=CIRCLE ( 'NONE', #1049, 12.00000000000000178 ) ;
#6938=DIRECTION ( 'NONE',  ( 0.000000000000000000, 1.000000000000000000, 0.000000000000000000 ) ) ;
#6943=( NAMED_UNIT ( * ) PLANE_ANGLE_UNIT ( ) SI_UNIT ( $, .RADIAN. ) );
#6945=AXIS2_PLACEMENT_3D ( 'NONE', #20896, #1832, #11236 ) ;
#6948=CARTESIAN_POINT ( 'NONE',  ( 116.0000000000000142, 6.735557395310442023E-16, 5.500000000000000000 ) ) ;
#6949=ORIENTED_EDGE ( 'NONE', *, *, #5471, .T. ) ;
#6951=CARTESIAN_POINT ( 'NONE',  ( 141.4687500000000853, -2.485281374238585972, 6.000000000000005329 ) ) ;
#6953=CARTESIAN_POINT ( 'NONE',  ( 142.6949251345948539, 5.500000000000012434, -2.278174593052012309 ) ) ;
#6954=CARTESIAN_POINT ( 'NONE',  ( 132.2812500000000000, 2.485281374238585972, 6.000000000000005329 ) ) ;
#6959=EDGE_CURVE ( 'NONE', #16005, #10874, #21463, .T. ) ;
#6960=ORIENTED_EDGE ( 'NONE', *, *, #23349, .T. ) ;
#6966=CARTESIAN_POINT ( 'NONE',  ( -4.999999999999920952, -65.50000000000001421, -7.500000000000007105 ) ) ;
#6982=CYLINDRICAL_SURFACE ( 'NONE', #11669, 5.500000000000000000 ) ;
#6985=CARTESIAN_POINT ( 'NONE',  ( 157.8750000000000568, 0.000000000000000000, 6.000000000000005329 ) ) ;
#6988=CARTESIAN_POINT ( 'NONE',  ( 139.0386751345948255, -5.500000000000005329, 0.000000000000000000 ) ) ;
#6992=ORIENTED_EDGE ( 'NONE', *, *, #3538, .F. ) ;
#6993=CARTESIAN_POINT ( 'NONE',  ( 148.3125000000000284, 4.242640687119298093, -4.242640687119298093 ) ) ;
#7005=CARTESIAN_POINT ( 'NONE',  ( 154.9538997308104058, -2.071067811865468400, -4.999999999999989342 ) ) ;
#7007=VERTEX_POINT ( 'NONE', #5390 ) ;
#7012=CARTESIAN_POINT ( 'NONE',  ( -4.999999999999886313, -10.50000000000000888, -8.000000000000007105 ) ) ;
#7021=CARTESIAN_POINT ( 'NONE',  ( 135.0581880922677556, -7.766452621457742289, 8.294963418928750443 ) ) ;
#7022=VERTEX_POINT ( 'NONE', #3382 ) ;
#7025=EDGE_CURVE ( 'NONE', #11375, #18429, #8691, .T. ) ;
#7029=VERTEX_POINT ( 'NONE', #17261 ) ;
#7033=ORIENTED_EDGE ( 'NONE', *, *, #13180, .F. ) ;
#7034=EDGE_CURVE ( 'NONE', #278, #18461, #19837, .T. ) ;
#7038=MECHANICAL_DESIGN_GEOMETRIC_PRESENTATION_REPRESENTATION('',(#7531),#4082);
#7039=EDGE_LOOP ( 'NONE', ( #21815, #7936, #29112, #12594 ) ) ;
#7040=CARTESIAN_POINT ( 'NONE',  ( 153.3750000000000284, 0.000000000000000000, 6.000000000000005329 ) ) ;
#7047=CARTESIAN_POINT ( 'NONE',  ( 141.0000000000000284, -11.31370849898477537, -4.000000000000003553 ) ) ;
#7051=CARTESIAN_POINT ( 'NONE',  ( -0.07773410149728489371, -14.92045216308241073, -8.102832156385545659 ) ) ;
#7058=( BOUNDED_CURVE ( )  B_SPLINE_CURVE ( 2, ( #25759, #253, #7606, #2854, #12418, #12273, #28792, #9636, #550 ),
 .UNSPECIFIED., .F., .T. ) 
 B_SPLINE_CURVE_WITH_KNOTS ( ( 3, 2, 2, 2, 3 ),
 ( 0.4124999999999989786, 0.4187499999999991784, 0.4249999999999994893, 0.4312499999999997446, 0.4374999999999999445 ),
 .UNSPECIFIED. ) 
 CURVE ( )  GEOMETRIC_REPRESENTATION_ITEM ( )  RATIONAL_B_SPLINE_CURVE ( ( 1.000000000000012212, 0.9238795325112745260, 1.000000000000000000, 0.9238795325112867385, 1.000000000000000000, 0.9238795325112867385, 1.000000000000000000, 0.9238795325112874046, 0.9999999999999993339 ) ) 
 REPRESENTATION_ITEM ( '' )  );
#7060=CARTESIAN_POINT ( 'NONE',  ( -9.999999999999772626, -90.00000000000001421, 4.000000000000003553 ) ) ;
#7061=CARTESIAN_POINT ( 'NONE',  ( 154.0238248654052313, 3.889087296526011706, -3.889087296526011706 ) ) ;
#7062=ORIENTED_EDGE ( 'NONE', *, *, #11589, .F. ) ;
#7064=FACE_OUTER_BOUND ( 'NONE', #20449, .T. ) ;
#7065=ADVANCED_FACE ( 'NONE', ( #1464 ), #13037, .F. ) ;
#7066=CARTESIAN_POINT ( 'NONE',  ( 135.5000000000000000, -54.99999999999993605, 8.000000000000007105 ) ) ;
#7072=DIRECTION ( 'NONE',  ( -1.000000000000000000, 0.000000000000000000, 0.000000000000000000 ) ) ;
#7074=ADVANCED_FACE ( 'NONE', ( #3765 ), #30114, .T. ) ;
#7075=CARTESIAN_POINT ( 'NONE',  ( 140.8050748654052029, 5.500000000000012434, 2.278174593052012309 ) ) ;
#7076=ORIENTED_EDGE ( 'NONE', *, *, #6618, .T. ) ;
#7077=ORIENTED_EDGE ( 'NONE', *, *, #17946, .T. ) ;
#7079=CARTESIAN_POINT ( 'NONE',  ( 138.8437500000000568, -6.000000000000005329, -2.485281374238555774 ) ) ;
#7081=FILL_AREA_STYLE_COLOUR ( '', #26960 ) ;
#7087=CARTESIAN_POINT ( 'NONE',  ( 145.2038997308104342, 2.071067811865468400, 4.999999999999989342 ) ) ;
#7093=SURFACE_SIDE_STYLE ('',( #28125 ) ) ;
#7094=CARTESIAN_POINT ( 'NONE',  ( 156.0863248654052597, 0.000000000000000000, 5.500000000000005329 ) ) ;
#7096=EDGE_CURVE ( 'NONE', #25843, #19300, #18753, .T. ) ;
#7103=CARTESIAN_POINT ( 'NONE',  ( 140.6250000000000284, 0.000000000000000000, -6.000000000000005329 ) ) ;
#7105=( GEOMETRIC_REPRESENTATION_CONTEXT ( 3 ) GLOBAL_UNCERTAINTY_ASSIGNED_CONTEXT ( ( #20074 ) ) GLOBAL_UNIT_ASSIGNED_CONTEXT ( ( #1701, #27034, #24744 ) ) REPRESENTATION_CONTEXT ( 'NONE', 'WORKASPACE' ) );
#7107=CARTESIAN_POINT ( 'NONE',  ( 159.6413997308104058, 2.071067811865468400, -4.999999999999989342 ) ) ;
#7109=ORIENTED_EDGE ( 'NONE', *, *, #12342, .F. ) ;
#7111=VECTOR ( 'NONE', #4218, 1000.000000000000000 ) ;
#7120=CARTESIAN_POINT ( 'NONE',  ( 1.000000000000000888, 0.000000000000000000, 0.000000000000000000 ) ) ;
#7131=ADVANCED_FACE ( 'NONE', ( #4880 ), #7177, .T. ) ;
#7132=PRESENTATION_STYLE_ASSIGNMENT (( #28162 ) ) ;
#7133=CARTESIAN_POINT ( 'NONE',  ( 143.8273502691896510, -5.000000000000004441, 0.000000000000000000 ) ) ;
#7134=CARTESIAN_POINT ( 'NONE',  ( 160.5863248654052597, 0.000000000000000000, 5.500000000000005329 ) ) ;
#7136=CARTESIAN_POINT ( 'NONE',  ( 156.4687500000000568, -2.485281374238585972, 6.000000000000005329 ) ) ;
#7137=FILL_AREA_STYLE_COLOUR ( '', #28092 ) ;
#7143=CARTESIAN_POINT ( 'NONE',  ( 147.4687500000000853, -2.485281374238585972, 6.000000000000005329 ) ) ;
#7144=DIRECTION ( 'NONE',  ( -0.000000000000000000, -0.000000000000000000, -1.000000000000000000 ) ) ;
#7146=DIRECTION ( 'NONE',  ( 0.000000000000000000, 0.000000000000000000, -1.000000000000000000 ) ) ;
#7147=ORIENTED_EDGE ( 'NONE', *, *, #10130, .T. ) ;
#7152=ORIENTED_EDGE ( 'NONE', *, *, #5521, .F. ) ;
#7155=FILL_AREA_STYLE_COLOUR ( '', #28437 ) ;
#7156=CARTESIAN_POINT ( 'NONE',  ( 158.9851497308104058, -3.535533905932725318, 3.535533905932725318 ) ) ;
#7159=CARTESIAN_POINT ( 'NONE',  ( 159.3675748654052029, -5.500000000000012434, 2.278174593052012309 ) ) ;
#7160=DIRECTION ( 'NONE',  ( -0.000000000000000000, 1.000000000000000000, -0.000000000000000000 ) ) ;
#7173=CARTESIAN_POINT ( 'NONE',  ( 157.9836002691896226, 4.999999999999989342, -2.071067811865468400 ) ) ;
#7177=TOROIDAL_SURFACE ( 'NONE', #27741, 11.00000000000000355, 1.000000000000000000 ) ;
#7178=UNCERTAINTY_MEASURE_WITH_UNIT (LENGTH_MEASURE( 1.000000000000000082E-05 ), #3707, 'distance_accuracy_value', 'NONE');
#7180=CARTESIAN_POINT ( 'NONE',  ( 139.5000000000000284, -54.99999999999990763, -8.000000000000007105 ) ) ;
#7182=VECTOR ( 'NONE', #28151, 1000.000000000000000 ) ;
#7184=ORIENTED_EDGE ( 'NONE', *, *, #23390, .T. ) ;
#7191=CARTESIAN_POINT ( 'NONE',  ( 149.6250000000000284, 0.000000000000000000, -6.000000000000005329 ) ) ;
#7196=ORIENTED_EDGE ( 'NONE', *, *, #18260, .F. ) ;
#7197=CARTESIAN_POINT ( 'NONE',  ( 151.5863248654052313, 0.000000000000000000, 5.500000000000005329 ) ) ;
#7201=EDGE_CURVE ( 'NONE', #22266, #1192, #26519, .T. ) ;
#7209=FILL_AREA_STYLE ('',( #25941 ) ) ;
#7211=UNCERTAINTY_MEASURE_WITH_UNIT (LENGTH_MEASURE( 1.000000000000000082E-05 ), #22543, 'distance_accuracy_value', 'NONE');
#7213=CARTESIAN_POINT ( 'NONE',  ( 159.0000000000000284, -59.99999999999980105, -4.000000000000003553 ) ) ;
#7215=EDGE_LOOP ( 'NONE', ( #17748, #26509, #21257, #29756 ) ) ;
#7217=CARTESIAN_POINT ( 'NONE',  ( 1.000000000000000888, -16.43939393939395188, 5.999693900976774685 ) ) ;
#7219=CARTESIAN_POINT ( 'NONE',  ( 0.9564710672350417164, -15.26172842777273964, 8.566785667046460162 ) ) ;
#7220=VECTOR ( 'NONE', #23593, 1000.000000000000000 ) ;
#7222=EDGE_LOOP ( 'NONE', ( #27147, #27902, #10951, #791 ) ) ;
#7223=MECHANICAL_DESIGN_GEOMETRIC_PRESENTATION_REPRESENTATION('',(#17548),#11166);
#7224=SURFACE_STYLE_USAGE ( .BOTH. , #12177 ) ;
#7225=DIRECTION ( 'NONE',  ( 1.000000000000000000, -0.000000000000000000, -0.000000000000000000 ) ) ;
#7233=CYLINDRICAL_SURFACE ( 'NONE', #1207, 9.999999999999998224 ) ;
#7234=CARTESIAN_POINT ( 'NONE',  ( 133.7812500000000284, 2.485281374238585972, 6.000000000000005329 ) ) ;
#7240=CARTESIAN_POINT ( 'NONE',  ( 144.5699251345947687, 2.278174593052290753, 5.499999999999732658 ) ) ;
#7242=CARTESIAN_POINT ( 'NONE',  ( 0.9562047175114668507, -15.26206247212127209, 8.566170523763496192 ) ) ;
#7245=CARTESIAN_POINT ( 'NONE',  ( 146.7038997308104342, 2.071067811865468400, 4.999999999999989342 ) ) ;
#7251=EDGE_CURVE ( 'NONE', #22616, #5051, #19883, .T. ) ;
#7252=CARTESIAN_POINT ( 'NONE',  ( 135.0000000000000284, -54.99999999999993605, 8.000000000000007105 ) ) ;
#7261=CARTESIAN_POINT ( 'NONE',  ( 138.9375000000000568, -4.242640687119298093, -4.242640687119298093 ) ) ;
#7264=CARTESIAN_POINT ( 'NONE',  ( 142.8824251345948824, 5.500000000000012434, 2.278174593052012309 ) ) ;
#7265=( GEOMETRIC_REPRESENTATION_CONTEXT ( 3 ) GLOBAL_UNCERTAINTY_ASSIGNED_CONTEXT ( ( #5123 ) ) GLOBAL_UNIT_ASSIGNED_CONTEXT ( ( #21918, #558, #26354 ) ) REPRESENTATION_CONTEXT ( 'NONE', 'WORKASPACE' ) );
#7266=TOROIDAL_SURFACE ( 'NONE', #12697, 10.49999999999999645, 0.5000000000000000000 ) ;
#7267=CARTESIAN_POINT ( 'NONE',  ( 133.0312500000000568, -2.485281374238555774, -6.000000000000005329 ) ) ;
#7271=AXIS2_PLACEMENT_3D ( 'NONE', #18685, #26016, #28160 ) ;
#7272=VERTEX_POINT ( 'NONE', #15180 ) ;
#7275=EDGE_CURVE ( 'NONE', #22336, #26257, #29722, .T. ) ;
#7276=DIRECTION ( 'NONE',  ( 0.000000000000000000, 0.000000000000000000, -1.000000000000000000 ) ) ;
#7286=CARTESIAN_POINT ( 'NONE',  ( 139.9650691573131098, -9.167294735415024931, 7.745767522440335284 ) ) ;
#7291=DIRECTION ( 'NONE',  ( 1.000000000000000000, -0.000000000000000000, -0.000000000000000000 ) ) ;
#7293=CARTESIAN_POINT ( 'NONE',  ( 139.5000000000000000, -9.165151389911669000, 8.000000000000007105 ) ) ;
#7294=CARTESIAN_POINT ( 'NONE',  ( 144.3898502691896510, 3.535533905932725318, -3.535533905932725318 ) ) ;
#7296=CARTESIAN_POINT ( 'NONE',  ( 160.1250000000000568, 0.000000000000000000, -6.000000000000005329 ) ) ;
#7297=CARTESIAN_POINT ( 'NONE',  ( 144.3675748654052597, -5.500000000000012434, 2.278174593052012309 ) ) ;
#7300=CARTESIAN_POINT ( 'NONE',  ( -15.49999999999999289, -54.99999999999990763, 7.500000000000007105 ) ) ;
#7302=VERTEX_POINT ( 'NONE', #4390 ) ;
#7303=CARTESIAN_POINT ( 'NONE',  ( 151.4062500000000000, 6.000000000000005329, -2.485281374238555774 ) ) ;
#7313=CARTESIAN_POINT ( 'NONE',  ( 154.3913997308104342, -2.071067811865468400, 4.999999999999989342 ) ) ;
#7314=CARTESIAN_POINT ( 'NONE',  ( 1.000000000000000888, -14.14213562373095634, 8.500000000000007105 ) ) ;
#7317=CARTESIAN_POINT ( 'NONE',  ( 160.8824251345948824, 5.500000000000012434, 2.278174593052012309 ) ) ;
#7325=CARTESIAN_POINT ( 'NONE',  ( 155.6398502691896510, -3.535533905932752852, 3.535533905932725318 ) ) ;
#7330=CARTESIAN_POINT ( 'NONE',  ( 116.0000000000000142, 6.735557395310442023E-16, 5.500000000000000000 ) ) ;
#7336=CARTESIAN_POINT ( 'NONE',  ( -19.99999999999998224, -25.00000000000010658, -7.500000000000007105 ) ) ;
#7338=EDGE_CURVE ( 'NONE', #6732, #29422, #13353, .T. ) ;
#7348=CARTESIAN_POINT ( 'NONE',  ( 159.0863248654052597, 0.000000000000000000, 5.500000000000005329 ) ) ;
#7352=CIRCLE ( 'NONE', #26467, 12.00000000000000178 ) ;
#7353=( NAMED_UNIT ( * ) SI_UNIT ( $, .STERADIAN. ) SOLID_ANGLE_UNIT ( ) );
#7354=ORIENTED_EDGE ( 'NONE', *, *, #14919, .F. ) ;
#7355=DIRECTION ( 'NONE',  ( 0.000000000000000000, 0.000000000000000000, 1.000000000000000000 ) ) ;
#7356=( NAMED_UNIT ( * ) PLANE_ANGLE_UNIT ( ) SI_UNIT ( $, .RADIAN. ) );
#7365=DIRECTION ( 'NONE',  ( 0.000000000000000000, -1.000000000000000000, 0.000000000000000000 ) ) ;
#7366=DIRECTION ( 'NONE',  ( 0.000000000000000000, 0.000000000000000000, 1.000000000000000000 ) ) ;
#7367=ORIENTED_EDGE ( 'NONE', *, *, #29347, .F. ) ;
#7372=CARTESIAN_POINT ( 'NONE',  ( -20.99999999999998224, -19.99999999999998934, 4.000000000000003553 ) ) ;
#7373=EDGE_CURVE ( 'NONE', #15059, #13602, #21796, .T. ) ;
#7376=VERTEX_POINT ( 'NONE', #25119 ) ;
#7380=ORIENTED_EDGE ( 'NONE', *, *, #7251, .T. ) ;
#7382=CARTESIAN_POINT ( 'NONE',  ( 133.6875000000000284, 4.242640687119269671, 4.242640687119298093 ) ) ;
#7383=EDGE_CURVE ( 'NONE', #6328, #20568, #25426, .T. ) ;
#7386=PLANE ( 'NONE',  #14753 ) ;
#7391=CARTESIAN_POINT ( 'NONE',  ( 0.9999999945711265381, -15.13437201258503606, 8.790312755061723493 ) ) ;
#7394=CARTESIAN_POINT ( 'NONE',  ( 135.9226497308104058, 5.000000000000004441, 0.000000000000000000 ) ) ;
#7398=( GEOMETRIC_REPRESENTATION_CONTEXT ( 3 ) GLOBAL_UNCERTAINTY_ASSIGNED_CONTEXT ( ( #5919 ) ) GLOBAL_UNIT_ASSIGNED_CONTEXT ( ( #21653, #14022, #12014 ) ) REPRESENTATION_CONTEXT ( 'NONE', 'WORKASPACE' ) );
#7399=CARTESIAN_POINT ( 'NONE',  ( 150.0863248654052313, 0.000000000000000000, 5.500000000000005329 ) ) ;
#7401=VECTOR ( 'NONE', #7225, 1000.000000000000000 ) ;
#7402=ORIENTED_EDGE ( 'NONE', *, *, #17451, .T. ) ;
#7406=ORIENTED_EDGE ( 'NONE', *, *, #13180, .T. ) ;
#7408=CARTESIAN_POINT ( 'NONE',  ( 135.0000000000000284, 6.000000000000005329, 0.000000000000000000 ) ) ;
#7409=EDGE_CURVE ( 'NONE', #27076, #8039, #2275, .T. ) ;
#7412=CARTESIAN_POINT ( 'NONE',  ( 160.2038997308104911, 2.071067811865468400, 4.999999999999989342 ) ) ;
#7414=EDGE_CURVE ( 'NONE', #21999, #605, #4201, .T. ) ;
#7420=CARTESIAN_POINT ( 'NONE',  ( 140.5000000000000284, -11.02592621076652790, -4.736429266082377687 ) ) ;
#7422=DIRECTION ( 'NONE',  ( 0.000000000000000000, 0.000000000000000000, 1.000000000000000000 ) ) ;
#7424=DIRECTION ( 'NONE',  ( 1.000000000000000000, -0.000000000000000000, 0.000000000000000000 ) ) ;
#7426=DIRECTION ( 'NONE',  ( -1.000000000000000000, -0.000000000000000000, -0.000000000000000000 ) ) ;
#7427=VECTOR ( 'NONE', #20322, 1000.000000000000000 ) ;
#7433=CARTESIAN_POINT ( 'NONE',  ( 154.9687500000000568, -2.485281374238585972, 6.000000000000005329 ) ) ;
#7434=CARTESIAN_POINT ( 'NONE',  ( 161.0000000000000284, 6.735557395310442023E-16, 5.500000000000000000 ) ) ;
#7435=EDGE_CURVE ( 'NONE', #15258, #11662, #20538, .T. ) ;
#7436=DIRECTION ( 'NONE',  ( 0.000000000000000000, 0.000000000000000000, 1.000000000000000000 ) ) ;
#7439=CARTESIAN_POINT ( 'NONE',  ( 147.7500000000000284, -6.000000000000005329, 0.000000000000000000 ) ) ;
#7440=VECTOR ( 'NONE', #11833, 1000.000000000000000 ) ;
#7441=AXIS2_PLACEMENT_3D ( 'NONE', #3783, #17497, #5776 ) ;
#7442=( NAMED_UNIT ( * ) SI_UNIT ( $, .STERADIAN. ) SOLID_ANGLE_UNIT ( ) );
#7443=ADVANCED_FACE ( 'NONE', ( #27567 ), #8413, .F. ) ;
#7453=CARTESIAN_POINT ( 'NONE',  ( 158.0476497308104342, 0.000000000000000000, -5.000000000000004441 ) ) ;
#7458=CARTESIAN_POINT ( 'NONE',  ( 140.0000000000000284, -10.99818166789400919, 4.800000000000004263 ) ) ;
#7460=CARTESIAN_POINT ( 'NONE',  ( 160.6949251345948539, 5.500000000000012434, -2.278174593052012309 ) ) ;
#7464=CARTESIAN_POINT ( 'NONE',  ( 142.1175748654052029, 5.500000000000012434, -2.278174593052012309 ) ) ;
#7471=ADVANCED_FACE ( 'NONE', ( #11048, #1491 ), #26821, .F. ) ;
#7472=SURFACE_SIDE_STYLE ('',( #19172 ) ) ;
#7475=VERTEX_POINT ( 'NONE', #19939 ) ;
#7476=LINE ( 'NONE', #14863, #10222 ) ;
#7479=ORIENTED_EDGE ( 'NONE', *, *, #8184, .T. ) ;
#7480=ORIENTED_EDGE ( 'NONE', *, *, #28701, .F. ) ;
#7484=UNCERTAINTY_MEASURE_WITH_UNIT (LENGTH_MEASURE( 1.000000000000000082E-05 ), #13423, 'distance_accuracy_value', 'NONE');
#7485=VECTOR ( 'NONE', #6936, 1000.000000000000000 ) ;
#7494=DIRECTION ( 'NONE',  ( -1.000000000000000000, -0.000000000000000000, -0.000000000000000000 ) ) ;
#7497=DIRECTION ( 'NONE',  ( 0.000000000000000000, 0.000000000000000000, 1.000000000000000000 ) ) ;
#7499=DIRECTION ( 'NONE',  ( 1.000000000000000000, -0.000000000000000000, -0.000000000000000000 ) ) ;
#7502=CARTESIAN_POINT ( 'NONE',  ( -0.5000000000000004441, -14.50000000000001243, -7.500000000000007105 ) ) ;
#7505=CARTESIAN_POINT ( 'NONE',  ( 0.8617483151293284793, -15.74632760175659740, 7.643625642394846764 ) ) ;
#7513=( NAMED_UNIT ( * ) PLANE_ANGLE_UNIT ( ) SI_UNIT ( $, .RADIAN. ) );
#7519=CARTESIAN_POINT ( 'NONE',  ( 161.4375000000000284, -4.242640687119298093, -4.242640687119298093 ) ) ;
#7522=PRESENTATION_STYLE_ASSIGNMENT (( #23826 ) ) ;
#7524=DIRECTION ( 'NONE',  ( -1.000000000000000000, -0.000000000000000000, -0.000000000000000000 ) ) ;
#7529=CARTESIAN_POINT ( 'NONE',  ( 140.4226497308104342, 5.000000000000004441, 0.000000000000000000 ) ) ;
#7530=CARTESIAN_POINT ( 'NONE',  ( 137.4300748654051745, 2.278174593051640162, -5.500000000000382805 ) ) ;
#7531=STYLED_ITEM ( 'NONE', ( #23012 ), #10296 ) ;
#7533=CARTESIAN_POINT ( 'NONE',  ( 116.0000000000000142, 0.000000000000000000, 0.000000000000000000 ) ) ;
#7539=ORIENTED_EDGE ( 'NONE', *, *, #13768, .T. ) ;
#7544=ADVANCED_FACE ( 'NONE', ( #15368 ), #16614, .T. ) ;
#7545=EDGE_LOOP ( 'NONE', ( #10436, #14069, #22073, #21409 ) ) ;
#7550=CARTESIAN_POINT ( 'NONE',  ( 134.5312500000000568, -2.485281374238555774, -6.000000000000005329 ) ) ;
#7559=CARTESIAN_POINT ( 'NONE',  ( -4.999999999999886313, -69.50000000000001421, -7.500000000000007105 ) ) ;
#7562=CARTESIAN_POINT ( 'NONE',  ( 140.6083823193137903, -11.80419115965732502, -4.059228028636178820 ) ) ;
#7569=CIRCLE ( 'NONE', #24753, 0.5000000000000000000 ) ;
#7572=ADVANCED_FACE ( 'NONE', ( #608 ), #28208, .T. ) ;
#7574=DIRECTION ( 'NONE',  ( 1.000000000000000000, 0.000000000000000000, -0.000000000000000000 ) ) ;
#7575=CARTESIAN_POINT ( 'NONE',  ( 143.2648502691896510, 3.535533905932725318, 3.535533905932752852 ) ) ;
#7576=CARTESIAN_POINT ( 'NONE',  ( 154.8750000000000284, 0.000000000000000000, 6.000000000000005329 ) ) ;
#7577=CARTESIAN_POINT ( 'NONE',  ( 149.1636751345948255, 0.000000000000000000, 5.500000000000005329 ) ) ;
#7583=EDGE_LOOP ( 'NONE', ( #14735, #19057, #25588, #7147 ) ) ;
#7584=CARTESIAN_POINT ( 'NONE',  ( 152.6250000000000284, 0.000000000000000000, -6.000000000000005329 ) ) ;
#7585=CARTESIAN_POINT ( 'NONE',  ( 161.5000000000000853, -2.984449860524901688, -5.205099329504969674 ) ) ;
#7586=UNCERTAINTY_MEASURE_WITH_UNIT (LENGTH_MEASURE( 1.000000000000000082E-05 ), #27666, 'distance_accuracy_value', 'NONE');
#7596=DIRECTION ( 'NONE',  ( -0.000000000000000000, -0.000000000000000000, -1.000000000000000000 ) ) ;
#7601=FACE_OUTER_BOUND ( 'NONE', #14455, .T. ) ;
#7606=CARTESIAN_POINT ( 'NONE',  ( 144.8511751345948255, -3.889087296526011706, 3.889087296526011706 ) ) ;
#7610=CARTESIAN_POINT ( 'NONE',  ( 156.3898502691896510, 3.535533905932725318, -3.535533905932725318 ) ) ;
#7616=CARTESIAN_POINT ( 'NONE',  ( 162.0000000000000284, 0.000000000000000000, 0.000000000000000000 ) ) ;
#7618=ORIENTED_EDGE ( 'NONE', *, *, #27114, .T. ) ;
#7619=AXIS2_PLACEMENT_3D ( 'NONE', #24246, #10291, #19657 ) ;
#7620=CARTESIAN_POINT ( 'NONE',  ( -0.07769256095283699759, -15.23231281889969679, -7.500000000000007105 ) ) ;
#7622=EDGE_LOOP ( 'NONE', ( #12193, #7623, #19248, #2779 ) ) ;
#7623=ORIENTED_EDGE ( 'NONE', *, *, #27984, .F. ) ;
#7624=AXIS2_PLACEMENT_3D ( 'NONE', #14542, #2673, #4832 ) ;
#7633=CARTESIAN_POINT ( 'NONE',  ( 133.7663997308104342, -4.999999999999989342, -2.071067811865468400 ) ) ;
#7634=ADVANCED_FACE ( 'NONE', ( #14764 ), #20892, .F. ) ;
#7637=CARTESIAN_POINT ( 'NONE',  ( 0.7909681984462132442, -15.46453874178244980, -8.191422655757447657 ) ) ;
#7638=EDGE_CURVE ( 'NONE', #8771, #3609, #26882, .T. ) ;
#7640=CARTESIAN_POINT ( 'NONE',  ( 141.5550748654052313, -5.500000000000012434, -2.278174593052012309 ) ) ;
#7647=SURFACE_STYLE_FILL_AREA ( #7209 ) ;
#7649=FILL_AREA_STYLE ('',( #5783 ) ) ;
#7651=LINE ( 'NONE', #5637, #3814 ) ;
#7653=CARTESIAN_POINT ( 'NONE',  ( 124.9999999999999432, -69.50000000000000000, -7.500000000000007105 ) ) ;
#7654=ORIENTED_EDGE ( 'NONE', *, *, #25589, .F. ) ;
#7658=FILL_AREA_STYLE_COLOUR ( '', #23130 ) ;
#7660=FACE_OUTER_BOUND ( 'NONE', #6562, .T. ) ;
#7661=VERTEX_POINT ( 'NONE', #21998 ) ;
#7663=ORIENTED_EDGE ( 'NONE', *, *, #22890, .T. ) ;
#7664=ORIENTED_EDGE ( 'NONE', *, *, #27810, .T. ) ;
#7666=CARTESIAN_POINT ( 'NONE',  ( -4.999999999999990230, -24.99999999999999289, -7.500000000000007105 ) ) ;
#7667=CARTESIAN_POINT ( 'NONE',  ( 160.4062500000000284, 6.000000000000005329, -2.485281374238555774 ) ) ;
#7671=DIRECTION ( 'NONE',  ( 1.000000000000000000, -0.000000000000000000, -0.000000000000000000 ) ) ;
#7672=CARTESIAN_POINT ( 'NONE',  ( -0.5000000000000004441, -10.00000000000000888, 7.500000000000007105 ) ) ;
#7673=DIRECTION ( 'NONE',  ( 0.000000000000000000, 0.000000000000000000, -1.000000000000000000 ) ) ;
#7676=CARTESIAN_POINT ( 'NONE',  ( 8.673617379884035472E-16, -16.43939393939395188, -5.999693900976774685 ) ) ;
#7681=CARTESIAN_POINT ( 'NONE',  ( 138.1726497308104342, -5.000000000000004441, 0.000000000000000000 ) ) ;
#7686=AXIS2_PLACEMENT_3D ( 'NONE', #955, #7574, #24306 ) ;
#7688=CARTESIAN_POINT ( 'NONE',  ( 154.2261751345948539, -3.889087296526011706, -3.889087296526011706 ) ) ;
#7696=CARTESIAN_POINT ( 'NONE',  ( 136.0312500000000284, -2.485281374238556218, -6.000000000000005329 ) ) ;
#7698=DIRECTION ( 'NONE',  ( 0.000000000000000000, 0.000000000000000000, -1.000000000000000000 ) ) ;
#7699=DIRECTION ( 'NONE',  ( 1.000000000000000000, -6.938893903907222067E-15, 0.000000000000000000 ) ) ;
#7711=CARTESIAN_POINT ( 'NONE',  ( 135.0000000000000284, 0.000000000000000000, 0.000000000000000000 ) ) ;
#7718=CARTESIAN_POINT ( 'NONE',  ( 141.0000000000000284, -12.00000000000001066, -4.000000000000003553 ) ) ;
#7721=CARTESIAN_POINT ( 'NONE',  ( 139.7459307364638050, -9.280942085683948406, 7.936758083481400661 ) ) ;
#7727=PRESENTATION_STYLE_ASSIGNMENT (( #26312 ) ) ;
#7728=CARTESIAN_POINT ( 'NONE',  ( 149.5312500000000284, -2.485281374238556218, -6.000000000000005329 ) ) ;
#7735=CARTESIAN_POINT ( 'NONE',  ( 146.1562500000000853, -6.000000000000005329, 2.485281374238555774 ) ) ;
#7736=AXIS2_PLACEMENT_3D ( 'NONE', #29174, #10793, #1384 ) ;
#7737=ADVANCED_FACE ( 'NONE', ( #3385 ), #2941, .F. ) ;
#7756=( BOUNDED_CURVE ( )  B_SPLINE_CURVE ( 2, ( #9968, #738, #10121, #12155, #427, #5326, #582, #9816, #17199 ),
 .UNSPECIFIED., .F., .T. ) 
 B_SPLINE_CURVE_WITH_KNOTS ( ( 3, 2, 2, 2, 3 ),
 ( 0.8624999999999993783, 0.8687499999999996891, 0.8749999999999998890, 0.8812500000000000888, 0.8875000000000003997 ),
 .UNSPECIFIED. ) 
 CURVE ( )  GEOMETRIC_REPRESENTATION_ITEM ( )  RATIONAL_B_SPLINE_CURVE ( ( 1.000000000000008216, 0.9238795325112786339, 1.000000000000000000, 0.9238795325112867385, 1.000000000000000000, 0.9238795325112867385, 1.000000000000000000, 0.9238795325112812984, 1.000000000000005329 ) ) 
 REPRESENTATION_ITEM ( '' )  );
#7765=CARTESIAN_POINT ( 'NONE',  ( 129.9999999999998010, -89.00000000000001421, 4.000000000000003553 ) ) ;
#7768=EDGE_LOOP ( 'NONE', ( #6540, #9827, #9192, #29555 ) ) ;
#7781=CARTESIAN_POINT ( 'NONE',  ( 0.8631338372297805428, -15.37878787878787534, -8.351220472436786224 ) ) ;
#7782=AXIS2_PLACEMENT_3D ( 'NONE', #27625, #20435, #3982 ) ;
#7783=DIRECTION ( 'NONE',  ( 0.000000000000000000, 1.000000000000000000, 0.000000000000000000 ) ) ;
#7793=DIRECTION ( 'NONE',  ( 0.000000000000000000, 0.000000000000000000, -1.000000000000000000 ) ) ;
#7800=VERTEX_POINT ( 'NONE', #17877 ) ;
#7803=EDGE_CURVE ( 'NONE', #20342, #22235, #23002, .T. ) ;
#7805=ORIENTED_EDGE ( 'NONE', *, *, #13913, .F. ) ;
#7808=AXIS2_PLACEMENT_3D ( 'NONE', #18338, #13587, #20002 ) ;
#7811=CARTESIAN_POINT ( 'NONE',  ( 132.7500000000000284, -6.000000000000005329, 0.000000000000000000 ) ) ;
#7812=CARTESIAN_POINT ( 'NONE',  ( 159.9375000000000284, -4.242640687119298093, -4.242640687119298093 ) ) ;
#7813=VECTOR ( 'NONE', #7160, 1000.000000000000000 ) ;
#7817=LINE ( 'NONE', #26559, #5240 ) ;
#7819=ORIENTED_EDGE ( 'NONE', *, *, #25616, .F. ) ;
#7823=CARTESIAN_POINT ( 'NONE',  ( 140.0476497308104058, 0.000000000000000000, -5.000000000000004441 ) ) ;
#7832=SURFACE_SIDE_STYLE ('',( #14785 ) ) ;
#7834=AXIS2_PLACEMENT_3D ( 'NONE', #14463, #7494, #10276 ) ;
#7835=ORIENTED_EDGE ( 'NONE', *, *, #28235, .T. ) ;
#7840=CARTESIAN_POINT ( 'NONE',  ( 153.1800748654052597, -2.278174593052058938, 5.499999999999964473 ) ) ;
#7847=EDGE_CURVE ( 'NONE', #3318, #20198, #2051, .T. ) ;
#7848=CARTESIAN_POINT ( 'NONE',  ( 155.1636751345948255, 0.000000000000000000, 5.500000000000005329 ) ) ;
#7850=ORIENTED_EDGE ( 'NONE', *, *, #17451, .F. ) ;
#7862=DIRECTION ( 'NONE',  ( 0.000000000000000000, 0.000000000000000000, 1.000000000000000000 ) ) ;
#7864=CARTESIAN_POINT ( 'NONE',  ( 0.000000000000000000, 9.000000000000007105, -3.000000000000002665 ) ) ;
#7865=SURFACE_STYLE_FILL_AREA ( #15596 ) ;
#7870=CARTESIAN_POINT ( 'NONE',  ( 146.8988248654052313, 3.889087296526011706, 3.889087296526011706 ) ) ;
#7874=FACE_OUTER_BOUND ( 'NONE', #2903, .T. ) ;
#7876=CARTESIAN_POINT ( 'NONE',  ( 141.9523502691896510, 0.000000000000000000, 5.000000000000004441 ) ) ;
#7877=CARTESIAN_POINT ( 'NONE',  ( 149.1562500000000568, -6.000000000000005329, 2.485281374238556218 ) ) ;
#7882=EDGE_CURVE ( 'NONE', #12140, #26257, #25236, .T. ) ;
#7884=CARTESIAN_POINT ( 'NONE',  ( 146.6250000000000284, 0.000000000000000000, -6.000000000000005329 ) ) ;
#7890=SURFACE_STYLE_FILL_AREA ( #10227 ) ;
#7894=STYLED_ITEM ( 'NONE', ( #22869 ), #12368 ) ;
#7896=SURFACE_STYLE_USAGE ( .BOTH. , #18597 ) ;
#7901=CARTESIAN_POINT ( 'NONE',  ( -4.999999999999886313, -70.00000000000001421, 7.500000000000007105 ) ) ;
#7906=CARTESIAN_POINT ( 'NONE',  ( -19.99999999999998224, -54.99999999999990763, 8.000000000000007105 ) ) ;
#7908=CARTESIAN_POINT ( 'NONE',  ( 154.2336002691896226, -4.999999999999989342, 2.071067811865468400 ) ) ;
#7909=CARTESIAN_POINT ( 'NONE',  ( 141.5699251345948255, 2.278174593052322283, 5.499999999999701572 ) ) ;
#7912=VECTOR ( 'NONE', #23542, 1000.000000000000000 ) ;
#7917=CARTESIAN_POINT ( 'NONE',  ( 159.6562500000000568, -6.000000000000005329, 2.485281374238555774 ) ) ;
#7922=CARTESIAN_POINT ( 'NONE',  ( 147.1875000000000284, 4.242640687119269671, 4.242640687119298093 ) ) ;
#7932=CARTESIAN_POINT ( 'NONE',  ( 135.0000000000000000, -7.309996799604661533, 8.297000954077597967 ) ) ;
#7933=CARTESIAN_POINT ( 'NONE',  ( 147.1011751345948539, 3.889087296526011706, -3.889087296526011706 ) ) ;
#7936=ORIENTED_EDGE ( 'NONE', *, *, #3016, .F. ) ;
#7941=CARTESIAN_POINT ( 'NONE',  ( 155.8988248654052313, 3.889087296526011706, 3.889087296526011706 ) ) ;
#7955=CARTESIAN_POINT ( 'NONE',  ( 141.0000000000000284, -19.99999999999998934, 4.000000000000003553 ) ) ;
#7957=ADVANCED_FACE ( 'NONE', ( #2759 ), #7233, .F. ) ;
#7958=ORIENTED_EDGE ( 'NONE', *, *, #18510, .F. ) ;
#7966=CARTESIAN_POINT ( 'NONE',  ( 133.7961002691896795, 2.071067811865468400, -4.999999999999989342 ) ) ;
#7967=ORIENTED_EDGE ( 'NONE', *, *, #493, .F. ) ;
#7974=CARTESIAN_POINT ( 'NONE',  ( 0.1285875681788154201, -16.20696777277755984, -6.610703565164271822 ) ) ;
#7977=CARTESIAN_POINT ( 'NONE',  ( 140.2351497308104058, 3.535533905932725318, -3.535533905932725318 ) ) ;
#7982=FILL_AREA_STYLE ('',( #29163 ) ) ;
#7988=AXIS2_PLACEMENT_3D ( 'NONE', #26353, #10098, #19037 ) ;
#7993=CARTESIAN_POINT ( 'NONE',  ( 124.9999999999999432, -70.00000000000000000, 8.000000000000007105 ) ) ;
#7996=CARTESIAN_POINT ( 'NONE',  ( 0.9868033348211117106, -16.18260772123498725, 6.670819112052090993 ) ) ;
#7997=PRESENTATION_STYLE_ASSIGNMENT (( #21067 ) ) ;
#8000=CARTESIAN_POINT ( 'NONE',  ( 135.2812500000000284, 2.485281374238585972, 6.000000000000005329 ) ) ;
#8002=SURFACE_STYLE_FILL_AREA ( #22149 ) ;
#8005=FILL_AREA_STYLE ('',( #26032 ) ) ;
#8006=DIRECTION ( 'NONE',  ( -0.000000000000000000, 0.000000000000000000, 1.000000000000000000 ) ) ;
#8008=ORIENTED_EDGE ( 'NONE', *, *, #5647, .F. ) ;
#8011=CARTESIAN_POINT ( 'NONE',  ( 136.7886751345948539, 5.500000000000005329, 0.000000000000000000 ) ) ;
#8014=DIRECTION ( 'NONE',  ( 0.000000000000000000, 0.000000000000000000, -1.000000000000000000 ) ) ;
#8015=CARTESIAN_POINT ( 'NONE',  ( 159.0788997308104058, -4.999999999999989342, 2.071067811865468400 ) ) ;
#8018=DIRECTION ( 'NONE',  ( 1.000000000000000000, -0.000000000000000000, -0.000000000000000000 ) ) ;
#8019=EDGE_CURVE ( 'NONE', #12140, #13151, #17455, .T. ) ;
#8029=CARTESIAN_POINT ( 'NONE',  ( 153.5625000000000568, -4.242640687119298093, 4.242640687119298093 ) ) ;
#8035=CARTESIAN_POINT ( 'NONE',  ( 143.9062500000000568, 6.000000000000005329, -2.485281374238555774 ) ) ;
#8036=CARTESIAN_POINT ( 'NONE',  ( 161.3144437930461095, -5.725702186695466267, 1.060355218292538204 ) ) ;
#8039=VERTEX_POINT ( 'NONE', #23530 ) ;
#8051=DIRECTION ( 'NONE',  ( 0.000000000000000000, 0.000000000000000000, -1.000000000000000000 ) ) ;
#8053=CARTESIAN_POINT ( 'NONE',  ( 153.6711002691896510, 4.999999999999989342, 2.071067811865468400 ) ) ;
#8054=CARTESIAN_POINT ( 'NONE',  ( 139.8141223307606822, -9.354659407854123643, -7.895782739253818683 ) ) ;
#8060=EDGE_LOOP ( 'NONE', ( #22863, #28351, #11971, #83 ) ) ;
#8061=CARTESIAN_POINT ( 'NONE',  ( 161.9062500000000568, 6.000000000000005329, -2.485281374238555774 ) ) ;
#8066=ORIENTED_EDGE ( 'NONE', *, *, #19582, .F. ) ;
#8075=CARTESIAN_POINT ( 'NONE',  ( 147.3824251345948255, 5.500000000000012434, 2.278174593052012309 ) ) ;
#8078=EDGE_LOOP ( 'NONE', ( #9009, #3834, #20377, #23634 ) ) ;
#8079=CARTESIAN_POINT ( 'NONE',  ( 0.1661021849294502251, -15.34535758500844693, -8.416596529583351582 ) ) ;
#8081=EDGE_CURVE ( 'NONE', #28850, #25181, #1854, .T. ) ;
#8083=CARTESIAN_POINT ( 'NONE',  ( -4.999999999999990230, -55.00000000000002132, -8.000000000000007105 ) ) ;
#8088=CARTESIAN_POINT ( 'NONE',  ( 154.6800748654052313, -2.278174593052082475, 5.499999999999942268 ) ) ;
#8091=( NAMED_UNIT ( * ) PLANE_ANGLE_UNIT ( ) SI_UNIT ( $, .RADIAN. ) );
#8095=ORIENTED_EDGE ( 'NONE', *, *, #28548, .T. ) ;
#8099=ORIENTED_EDGE ( 'NONE', *, *, #14576, .T. ) ;
#8101=CIRCLE ( 'NONE', #27725, 5.500000000000000000 ) ;
#8105=ORIENTED_EDGE ( 'NONE', *, *, #27883, .F. ) ;
#8106=CARTESIAN_POINT ( 'NONE',  ( 160.5937500000000284, 6.000000000000005329, 2.485281374238585972 ) ) ;
#8107=ADVANCED_FACE ( 'NONE', ( #9349 ), #30170, .T. ) ;
#8112=DIRECTION ( 'NONE',  ( 1.000000000000000000, 0.000000000000000000, 0.000000000000000000 ) ) ;
#8124=CARTESIAN_POINT ( 'NONE',  ( 0.7669223171414829565, -15.58766199952932396, -7.954545454545463912 ) ) ;
#8127=FACE_OUTER_BOUND ( 'NONE', #18898, .T. ) ;
#8128=CARTESIAN_POINT ( 'NONE',  ( 135.0000000000000284, 1.949781249179022291, 5.142796231657420947 ) ) ;
#8129=CARTESIAN_POINT ( 'NONE',  ( 147.8511751345948255, -3.889087296526011706, 3.889087296526011706 ) ) ;
#8130=CARTESIAN_POINT ( 'NONE',  ( -4.999999999999886313, -10.00000000000000888, 8.000000000000007105 ) ) ;
#8132=SURFACE_STYLE_USAGE ( .BOTH. , #7832 ) ;
#8134=ORIENTED_EDGE ( 'NONE', *, *, #29593, .F. ) ;
#8137=DIRECTION ( 'NONE',  ( 0.000000000000000000, -0.9393939393939397808, -0.3428396514843859988 ) ) ;
#8144=DIRECTION ( 'NONE',  ( 0.000000000000000000, 0.000000000000000000, -1.000000000000000000 ) ) ;
#8146=CARTESIAN_POINT ( 'NONE',  ( 140.1363996827915059, -11.13639968279144732, 4.472640761300552548 ) ) ;
#8148=ORIENTED_EDGE ( 'NONE', *, *, #8340, .F. ) ;
#8152=CARTESIAN_POINT ( 'NONE',  ( 136.5074251345947971, 2.278174593051935037, -5.500000000000088818 ) ) ;
#8156=CARTESIAN_POINT ( 'NONE',  ( 1.000000000000000888, 0.000000000000000000, 0.000000000000000000 ) ) ;
#8157=CARTESIAN_POINT ( 'NONE',  ( 148.2976497308104058, 0.000000000000000000, 5.000000000000004441 ) ) ;
#8163=CARTESIAN_POINT ( 'NONE',  ( 135.0000000000000284, -6.982120021884474781, 8.500000000000007105 ) ) ;
#8172=CARTESIAN_POINT ( 'NONE',  ( 145.1250000000000284, 0.000000000000000000, -6.000000000000005329 ) ) ;
#8173=DIRECTION ( 'NONE',  ( 0.000000000000000000, 0.000000000000000000, -1.000000000000000000 ) ) ;
#8174=STYLED_ITEM ( 'NONE', ( #4281 ), #6354 ) ;
#8176=CIRCLE ( 'NONE', #23902, 0.5000000000000004441 ) ;
#8179=EDGE_LOOP ( 'NONE', ( #25484, #9475, #27381, #15996, #5358, #18560, #29209, #8587, #18351, #18517, #20114, #6333, #12615, #5611, #15389, #183, #23824 ) ) ;
#8180=CARTESIAN_POINT ( 'NONE',  ( 145.1250000000000284, 0.000000000000000000, -6.000000000000005329 ) ) ;
#8182=VERTEX_POINT ( 'NONE', #28214 ) ;
#8184=EDGE_CURVE ( 'NONE', #10874, #27076, #25777, .T. ) ;
#8188=VERTEX_POINT ( 'NONE', #21220 ) ;
#8196=AXIS2_PLACEMENT_3D ( 'NONE', #5050, #24244, #12180 ) ;
#8206=CARTESIAN_POINT ( 'NONE',  ( 151.0461002691896510, -2.071067811865468400, 4.999999999999989342 ) ) ;
#8209=VECTOR ( 'NONE', #1213, 1000.000000000000000 ) ;
#8213=CARTESIAN_POINT ( 'NONE',  ( 150.4613248654052029, -5.500000000000005329, 0.000000000000000000 ) ) ;
#8216=CARTESIAN_POINT ( 'NONE',  ( 161.1562500000000284, -6.000000000000005329, 2.485281374238555774 ) ) ;
#8219=( GEOMETRIC_REPRESENTATION_CONTEXT ( 3 ) GLOBAL_UNCERTAINTY_ASSIGNED_CONTEXT ( ( #7586 ) ) GLOBAL_UNIT_ASSIGNED_CONTEXT ( ( #27666, #5192, #23257 ) ) REPRESENTATION_CONTEXT ( 'NONE', 'WORKASPACE' ) );
#8221=CARTESIAN_POINT ( 'NONE',  ( 143.9136751345948539, 0.000000000000000000, -5.500000000000005329 ) ) ;
#8225=DIRECTION ( 'NONE',  ( 1.000000000000000000, -0.000000000000000000, -0.000000000000000000 ) ) ;
#8232=EDGE_LOOP ( 'NONE', ( #9194, #8134, #16194, #15894 ) ) ;
#8235=FACE_OUTER_BOUND ( 'NONE', #20770, .T. ) ;
#8236=CARTESIAN_POINT ( 'NONE',  ( 141.0863248654052313, 0.000000000000000000, 5.500000000000005329 ) ) ;
#8242=CARTESIAN_POINT ( 'NONE',  ( 116.0000000000000142, 0.000000000000000000, -5.500000000000000000 ) ) ;
#8246=CARTESIAN_POINT ( 'NONE',  ( 135.2746852666345774, -8.503752835045871095, 8.096569711865882368 ) ) ;
#8247=VERTEX_POINT ( 'NONE', #162 ) ;
#8250=CARTESIAN_POINT ( 'NONE',  ( 135.3654420556978835, -8.709829393440356782, -8.045671146456855993 ) ) ;
#8252=ORIENTED_EDGE ( 'NONE', *, *, #5344, .T. ) ;
#8263=CARTESIAN_POINT ( 'NONE',  ( 155.6250000000000284, 0.000000000000000000, -6.000000000000005329 ) ) ;
#8266=CARTESIAN_POINT ( 'NONE',  ( 151.4136751345948539, 0.000000000000000000, -5.500000000000005329 ) ) ;
#8274=CARTESIAN_POINT ( 'NONE',  ( 0.2150838311359447030, -15.80975343865253713, -7.511900204273787907 ) ) ;
#8277=CARTESIAN_POINT ( 'NONE',  ( 159.2681041991610016, -11.07692307732762771, -4.615384614413698294 ) ) ;
#8286=CARTESIAN_POINT ( 'NONE',  ( -4.999999999999886313, -9.000000000000007105, -4.000000000000003553 ) ) ;
#8293=DIRECTION ( 'NONE',  ( 1.000000000000000000, 0.000000000000000000, 1.734723475976807094E-15 ) ) ;
#8297=FACE_OUTER_BOUND ( 'NONE', #24817, .T. ) ;
#8298=ORIENTED_EDGE ( 'NONE', *, *, #17909, .T. ) ;
#8303=EDGE_CURVE ( 'NONE', #5729, #7007, #22313, .T. ) ;
#8305=DIRECTION ( 'NONE',  ( -1.734723475976824844E-16, 1.000000000000000000, -0.000000000000000000 ) ) ;
#8307=CARTESIAN_POINT ( 'NONE',  ( 159.0723610732460713, -12.00000000000000888, 4.000000000000001776 ) ) ;
#8308=CARTESIAN_POINT ( 'NONE',  ( 143.9062500000000568, 6.000000000000005329, -2.485281374238555774 ) ) ;
#8311=CARTESIAN_POINT ( 'NONE',  ( 136.1175748654052313, 5.500000000000012434, -2.278174593052012309 ) ) ;
#8314=CARTESIAN_POINT ( 'NONE',  ( 140.7261751345948539, -3.889087296526011706, -3.889087296526011706 ) ) ;
#8315=CARTESIAN_POINT ( 'NONE',  ( 136.1324251345948539, -5.500000000000012434, -2.278174593052012309 ) ) ;
#8317=CARTESIAN_POINT ( 'NONE',  ( 136.0000000000000284, -8.946933499675704837, -8.000000000000007105 ) ) ;
#8318=CARTESIAN_POINT ( 'NONE',  ( 151.6726497308104058, -5.000000000000004441, 0.000000000000000000 ) ) ;
#8323=CARTESIAN_POINT ( 'NONE',  ( 135.3281957118843479, -8.627452770990513997, 8.066272317427783278 ) ) ;
#8327=VERTEX_POINT ( 'NONE', #2610 ) ;
#8334=CARTESIAN_POINT ( 'NONE',  ( 146.9062500000000568, 6.000000000000005329, -2.485281374238556218 ) ) ;
#8337=( GEOMETRIC_REPRESENTATION_CONTEXT ( 3 ) GLOBAL_UNCERTAINTY_ASSIGNED_CONTEXT ( ( #28383 ) ) GLOBAL_UNIT_ASSIGNED_CONTEXT ( ( #314, #7, #17081 ) ) REPRESENTATION_CONTEXT ( 'NONE', 'WORKASPACE' ) );
#8338=FILL_AREA_STYLE_COLOUR ( '', #4774 ) ;
#8340=EDGE_CURVE ( 'NONE', #1935, #27983, #6168, .T. ) ;
#8342=ORIENTED_EDGE ( 'NONE', *, *, #1254, .F. ) ;
#8343=CARTESIAN_POINT ( 'NONE',  ( 143.2500000000000568, -6.000000000000005329, 0.000000000000000000 ) ) ;
#8344=CARTESIAN_POINT ( 'NONE',  ( 161.4835765834562267, -3.531227715922129917, -4.872661563383335448 ) ) ;
#8349=EDGE_LOOP ( 'NONE', ( #19526, #3190, #28586 ) ) ;
#8354=ORIENTED_EDGE ( 'NONE', *, *, #15196, .T. ) ;
#8358=CYLINDRICAL_SURFACE ( 'NONE', #16543, 1.000000000000000888 ) ;
#8359=CIRCLE ( 'NONE', #508, 0.5000000000000004441 ) ;
#8366=CARTESIAN_POINT ( 'NONE',  ( 156.4613248654052029, -5.500000000000005329, 0.000000000000000000 ) ) ;
#8373=CARTESIAN_POINT ( 'NONE',  ( 152.7336002691896510, -4.999999999999989342, 2.071067811865468400 ) ) ;
#8375=CARTESIAN_POINT ( 'NONE',  ( -20.99999999999998224, -19.99999999999998934, 5.000000000000004441 ) ) ;
#8376=CARTESIAN_POINT ( 'NONE',  ( 135.1949251345948539, 5.500000000000012434, -2.278174593052012309 ) ) ;
#8380=CYLINDRICAL_SURFACE ( 'NONE', #23838, 0.5000000000000004441 ) ;
#8382=CARTESIAN_POINT ( 'NONE',  ( 160.3125000000000284, 4.242640687119298093, -4.242640687119298093 ) ) ;
#8384=CARTESIAN_POINT ( 'NONE',  ( 145.6949251345948255, 5.500000000000012434, -2.278174593052012309 ) ) ;
#8387=UNCERTAINTY_MEASURE_WITH_UNIT (LENGTH_MEASURE( 1.000000000000000082E-05 ), #22279, 'distance_accuracy_value', 'NONE');
#8388=ORIENTED_EDGE ( 'NONE', *, *, #13236, .T. ) ;
#8395=CARTESIAN_POINT ( 'NONE',  ( 135.0000000000000568, -8.296129373581107913, 7.693241659069887994 ) ) ;
#8399=ORIENTED_EDGE ( 'NONE', *, *, #13249, .T. ) ;
#8402=CARTESIAN_POINT ( 'NONE',  ( 155.3363248654052313, 0.000000000000000000, -5.500000000000005329 ) ) ;
#8413=CYLINDRICAL_SURFACE ( 'NONE', #27260, 5.500000000000000000 ) ;
#8414=CARTESIAN_POINT ( 'NONE',  ( 141.1949251345947971, 5.500000000000012434, -2.278174593052012309 ) ) ;
#8415=CARTESIAN_POINT ( 'NONE',  ( 135.0968198485644791, -7.962041090232468754, 8.242705641925590854 ) ) ;
#8417=ORIENTED_EDGE ( 'NONE', *, *, #3365, .T. ) ;
#8422=ORIENTED_EDGE ( 'NONE', *, *, #29593, .T. ) ;
#8423=CARTESIAN_POINT ( 'NONE',  ( 139.5863248654052313, 0.000000000000000000, 5.500000000000005329 ) ) ;
#8427=EDGE_LOOP ( 'NONE', ( #9612, #10601, #16608, #26000 ) ) ;
#8429=ORIENTED_EDGE ( 'NONE', *, *, #27593, .T. ) ;
#8431=CARTESIAN_POINT ( 'NONE',  ( 157.0312500000000853, -2.485281374238555774, -6.000000000000005329 ) ) ;
#8439=CARTESIAN_POINT ( 'NONE',  ( 159.0000000000000853, -11.33333333333334281, 4.000000000000006217 ) ) ;
#8443=CARTESIAN_POINT ( 'NONE',  ( -0.08077072505711925532, -15.22017114206482269, -7.626010301205228714 ) ) ;
#8445=CARTESIAN_POINT ( 'NONE',  ( 140.0550748654052597, -5.500000000000012434, -2.278174593052012309 ) ) ;
#8446=CARTESIAN_POINT ( 'NONE',  ( 0.7509536901451536739, -15.55282566733050942, -8.022540739038966251 ) ) ;
#8453=CARTESIAN_POINT ( 'NONE',  ( 148.2261751345948539, -3.889087296526011706, -3.889087296526011706 ) ) ;
#8461=CARTESIAN_POINT ( 'NONE',  ( 141.3898502691896510, 3.535533905932725318, -3.535533905932725318 ) ) ;
#8467=CARTESIAN_POINT ( 'NONE',  ( 147.6636751345948255, 0.000000000000000000, 5.500000000000005329 ) ) ;
#8471=CARTESIAN_POINT ( 'NONE',  ( 142.5000000000000568, 6.000000000000005329, 0.000000000000000000 ) ) ;
#8472=ORIENTED_EDGE ( 'NONE', *, *, #2159, .T. ) ;
#8473=DIRECTION ( 'NONE',  ( 0.000000000000000000, 0.000000000000000000, 1.000000000000000000 ) ) ;
#8474=ADVANCED_FACE ( 'NONE', ( #26550 ), #15519, .T. ) ;
#8476=CARTESIAN_POINT ( 'NONE',  ( 136.6011751345948539, 3.889087296526011706, -3.889087296526011706 ) ) ;
#8479=CARTESIAN_POINT ( 'NONE',  ( 153.0788997308104058, -4.999999999999989342, 2.071067811865468400 ) ) ;
#8481=DIRECTION ( 'NONE',  ( 1.000000000000000000, 1.067522139062651411E-16, 0.000000000000000000 ) ) ;
#8488=( NAMED_UNIT ( * ) SI_UNIT ( $, .STERADIAN. ) SOLID_ANGLE_UNIT ( ) );
#8496=CARTESIAN_POINT ( 'NONE',  ( 144.8437500000000000, -6.000000000000005329, -2.485281374238556218 ) ) ;
#8499=ORIENTED_EDGE ( 'NONE', *, *, #6809, .T. ) ;
#8500=CARTESIAN_POINT ( 'NONE',  ( 136.3125000000000284, 4.242640687119298093, -4.242640687119298093 ) ) ;
#8501=CARTESIAN_POINT ( 'NONE',  ( 161.3463853183868366, -5.851553901883566944, -0.2004824262064201779 ) ) ;
#8504=ORIENTED_EDGE ( 'NONE', *, *, #4839, .F. ) ;
#8510=VERTEX_POINT ( 'NONE', #25297 ) ;
#8511=DIRECTION ( 'NONE',  ( 1.000000000000000000, 1.734723475976843579E-16, -0.000000000000000000 ) ) ;
#8513=CARTESIAN_POINT ( 'NONE',  ( 135.0000000000000284, -6.982120021884474781, -8.500000000000007105 ) ) ;
#8515=EDGE_CURVE ( 'NONE', #28288, #28619, #30196, .T. ) ;
#8519=DIRECTION ( 'NONE',  ( 0.000000000000000000, 0.000000000000000000, 1.000000000000000000 ) ) ;
#8524=DIRECTION ( 'NONE',  ( -1.000000000000000000, 0.000000000000000000, 0.000000000000000000 ) ) ;
#8527=CARTESIAN_POINT ( 'NONE',  ( 153.4836002691896226, 4.999999999999989342, -2.071067811865468400 ) ) ;
#8528=CARTESIAN_POINT ( 'NONE',  ( 150.2886751345948255, 5.500000000000005329, 0.000000000000000000 ) ) ;
#8530=CARTESIAN_POINT ( 'NONE',  ( 135.5699251345948255, 2.278174593052383567, 5.499999999999640288 ) ) ;
#8533=LINE ( 'NONE', #27254, #28333 ) ;
#8536=CARTESIAN_POINT ( 'NONE',  ( 154.7812500000000568, 2.485281374238585972, 6.000000000000005329 ) ) ;
#8537=CARTESIAN_POINT ( 'NONE',  ( -0.07769256095284393648, -15.23231281889969679, 7.500000000000007105 ) ) ;
#8542=VERTEX_POINT ( 'NONE', #4267 ) ;
#8543=EDGE_LOOP ( 'NONE', ( #1369, #17511, #19146 ) ) ;
#8551=DIRECTION ( 'NONE',  ( 0.000000000000000000, 0.000000000000000000, -1.000000000000000000 ) ) ;
#8554=EDGE_CURVE ( 'NONE', #27945, #17372, #13846, .T. ) ;
#8555=FACE_OUTER_BOUND ( 'NONE', #12024, .T. ) ;
#8557=CARTESIAN_POINT ( 'NONE',  ( 155.9925748654052313, 2.278174593051927044, 5.500000000000096811 ) ) ;
#8564=CARTESIAN_POINT ( 'NONE',  ( 116.0000000000000142, 0.000000000000000000, 0.000000000000000000 ) ) ;
#8567=VERTEX_POINT ( 'NONE', #15849 ) ;
#8578=( BOUNDED_CURVE ( )  B_SPLINE_CURVE ( 2, ( #9096, #18493, #14354, #25518, #23398, #2188, #16357, #9247, #28269 ),
 .UNSPECIFIED., .F., .T. ) 
 B_SPLINE_CURVE_WITH_KNOTS ( ( 3, 2, 2, 2, 3 ),
 ( 0.7875000000000001998, 0.7937499999999999556, 0.7999999999999998224, 0.8062499999999995781, 0.8124999999999993339 ),
 .UNSPECIFIED. ) 
 CURVE ( )  GEOMETRIC_REPRESENTATION_ITEM ( )  RATIONAL_B_SPLINE_CURVE ( ( 0.9999999999999973355, 0.9238795325112894030, 1.000000000000000000, 0.9238795325112867385, 1.000000000000000000, 0.9238795325112867385, 1.000000000000000000, 0.9238795325112948431, 0.9999999999999918954 ) ) 
 REPRESENTATION_ITEM ( '' )  );
#8581=ORIENTED_EDGE ( 'NONE', *, *, #7251, .F. ) ;
#8583=CARTESIAN_POINT ( 'NONE',  ( 158.8125000000000284, 4.242640687119298093, -4.242640687119298093 ) ) ;
#8584=EDGE_CURVE ( 'NONE', #10268, #17372, #5656, .T. ) ;
#8587=ORIENTED_EDGE ( 'NONE', *, *, #15384, .T. ) ;
#8592=CARTESIAN_POINT ( 'NONE',  ( 116.0000000000000142, 0.000000000000000000, 0.000000000000000000 ) ) ;
#8596=( GEOMETRIC_REPRESENTATION_CONTEXT ( 3 ) GLOBAL_UNCERTAINTY_ASSIGNED_CONTEXT ( ( #418 ) ) GLOBAL_UNIT_ASSIGNED_CONTEXT ( ( #11834, #11365, #2272 ) ) REPRESENTATION_CONTEXT ( 'NONE', 'WORKASPACE' ) );
#8608=ORIENTED_EDGE ( 'NONE', *, *, #26434, .F. ) ;
#8611=CARTESIAN_POINT ( 'NONE',  ( 159.8363248654052313, 0.000000000000000000, -5.500000000000005329 ) ) ;
#8612=CARTESIAN_POINT ( 'NONE',  ( 141.1086002691896226, -2.071067811865468400, -4.999999999999989342 ) ) ;
#8613=ORIENTED_EDGE ( 'NONE', *, *, #9184, .F. ) ;
#8618=CARTESIAN_POINT ( 'NONE',  ( 140.0000000000000284, -11.48520880827726032, -4.868161254798472726 ) ) ;
#8623=CARTESIAN_POINT ( 'NONE',  ( 144.8437500000000000, -6.000000000000005329, -2.485281374238555774 ) ) ;
#8628=STYLED_ITEM ( 'NONE', ( #2043 ), #19286 ) ;
#8632=CARTESIAN_POINT ( 'NONE',  ( 161.0000000000000284, -11.67610212985248452, -2.769230769230773603 ) ) ;
#8635=CYLINDRICAL_SURFACE ( 'NONE', #16236, 1.000000000000000000 ) ;
#8636=CARTESIAN_POINT ( 'NONE',  ( 147.4538997308104058, -2.071067811865468400, -4.999999999999989342 ) ) ;
#8638=DIRECTION ( 'NONE',  ( 1.067522139062651411E-16, -1.000000000000000000, 0.000000000000000000 ) ) ;
#8639=FACE_OUTER_BOUND ( 'NONE', #4901, .T. ) ;
#8640=FILL_AREA_STYLE ('',( #18189 ) ) ;
#8644=ORIENTED_EDGE ( 'NONE', *, *, #5834, .F. ) ;
#8645=COLOUR_RGB ( '', 0.40784314, 0.44705882, 0.49803922) ;
#8648=B_SPLINE_CURVE_WITH_KNOTS ( 'NONE', 3,
 ( #9294, #9142, #30177, #16697, #13951, #12091, #26018, #21432, #363, #7293 ),
 .UNSPECIFIED., .F., .F.,
 ( 4, 2, 2, 2, 4 ),
 ( 0.000000000000000000, 0.0005899865232072658413, 0.0008849797848109120435, 0.001032476415612737638, 0.001179973046414563558 ),
 .UNSPECIFIED. ) ;
#8651=STYLED_ITEM ( 'NONE', ( #24165 ), #24848 ) ;
#8655=CARTESIAN_POINT ( 'NONE',  ( 144.7500000000000568, -6.000000000000005329, 0.000000000000000000 ) ) ;
#8656=CARTESIAN_POINT ( 'NONE',  ( 142.3199251345948539, -2.278174593052058938, -5.499999999999964473 ) ) ;
#8657=VECTOR ( 'NONE', #28350, 1000.000000000000000 ) ;
#8659=CARTESIAN_POINT ( 'NONE',  ( 124.9999999999999432, -71.00000000000001421, -4.000000000000003553 ) ) ;
#8660=CARTESIAN_POINT ( 'NONE',  ( 138.9375000000000568, -4.242640687119298093, -4.242640687119298093 ) ) ;
#8665=ADVANCED_FACE ( 'NONE', ( #14594 ), #28375, .T. ) ;
#8669=AXIS2_PLACEMENT_3D ( 'NONE', #7533, #10465, #17389 ) ;
#8675=CARTESIAN_POINT ( 'NONE',  ( -4.999999999999879208, -9.000000000000007105, -4.000000000000003553 ) ) ;
#8680=CARTESIAN_POINT ( 'NONE',  ( 136.6800748654052313, -2.278174593051950136, 5.500000000000074607 ) ) ;
#8682=PRODUCT_DEFINITION_SHAPE ( 'NONE', 'NONE',  #20816 ) ;
#8684=DIRECTION ( 'NONE',  ( -0.000000000000000000, -0.000000000000000000, -1.000000000000000000 ) ) ;
#8685=CARTESIAN_POINT ( 'NONE',  ( -9.999999999999980460, -60.00000000000001421, -4.000000000000003553 ) ) ;
#8688=CARTESIAN_POINT ( 'NONE',  ( 148.5148502691896510, -3.535533905932725318, -3.535533905932725318 ) ) ;
#8690=CARTESIAN_POINT ( 'NONE',  ( 124.9999999999999432, -65.50000000000000000, 7.500000000000007105 ) ) ;
#8691=CIRCLE ( 'NONE', #1813, 12.00000000000000178 ) ;
#8692=CARTESIAN_POINT ( 'NONE',  ( 140.5000000000000284, -10.99818166789401275, -4.799999999999998934 ) ) ;
#8693=EDGE_CURVE ( 'NONE', #24844, #9038, #4687, .T. ) ;
#8694=CARTESIAN_POINT ( 'NONE',  ( 139.3199251345948255, -2.278174593052098018, -5.499999999999928058 ) ) ;
#8695=CARTESIAN_POINT ( 'NONE',  ( 140.0000000000000284, -54.99999999999990763, -5.000000000000004441 ) ) ;
#8697=EDGE_LOOP ( 'NONE', ( #16530, #7062, #18334, #14442 ) ) ;
#8698=CARTESIAN_POINT ( 'NONE',  ( 156.1875000000000284, 4.242640687119269671, 4.242640687119298093 ) ) ;
#8699=CARTESIAN_POINT ( 'NONE',  ( -4.999999999999886313, -10.00000000000000888, 5.000000000000004441 ) ) ;
#8706=MECHANICAL_DESIGN_GEOMETRIC_PRESENTATION_REPRESENTATION('',(#16097),#26799);
#8712=CARTESIAN_POINT ( 'NONE',  ( 140.1564095343160830, -9.003322169323498159, -7.934381245738292954 ) ) ;
#8716=( NAMED_UNIT ( * ) SI_UNIT ( $, .STERADIAN. ) SOLID_ANGLE_UNIT ( ) );
#8717=CARTESIAN_POINT ( 'NONE',  ( -0.5000000000000004441, -10.50000000000000888, -7.500000000000007105 ) ) ;
#8724=DIRECTION ( 'NONE',  ( 0.000000000000000000, 0.000000000000000000, 1.000000000000000000 ) ) ;
#8732=EDGE_CURVE ( 'NONE', #6912, #4935, #7756, .T. ) ;
#8733=( GEOMETRIC_REPRESENTATION_CONTEXT ( 3 ) GLOBAL_UNCERTAINTY_ASSIGNED_CONTEXT ( ( #21743 ) ) GLOBAL_UNIT_ASSIGNED_CONTEXT ( ( #19254, #10026, #14797 ) ) REPRESENTATION_CONTEXT ( 'NONE', 'WORKASPACE' ) );
#8737=( LENGTH_UNIT ( ) NAMED_UNIT ( * ) SI_UNIT ( .MILLI., .METRE. ) );
#8740=ORIENTED_EDGE ( 'NONE', *, *, #29699, .T. ) ;
#8743=ADVANCED_FACE ( 'NONE', ( #8235 ), #29203, .F. ) ;
#8746=CARTESIAN_POINT ( 'NONE',  ( 156.5625000000000284, -4.242640687119298093, 4.242640687119298093 ) ) ;
#8749=ORIENTED_EDGE ( 'NONE', *, *, #24622, .T. ) ;
#8750=CARTESIAN_POINT ( 'NONE',  ( 150.7574251345948539, -2.278174593051764951, 5.500000000000262013 ) ) ;
#8754=CARTESIAN_POINT ( 'NONE',  ( 160.7532596262684592, -11.42128382377059737, 3.688773085009012576 ) ) ;
#8759=CARTESIAN_POINT ( 'NONE',  ( 159.1340520995980228, -12.00000000044276227, -4.000000000000002665 ) ) ;
#8761=CARTESIAN_POINT ( 'NONE',  ( 157.6800748654052313, -2.278174593052104679, 5.499999999999918288 ) ) ;
#8765=CARTESIAN_POINT ( 'NONE',  ( -4.999999999999990230, -24.99999999999999289, -7.500000000000007105 ) ) ;
#8771=VERTEX_POINT ( 'NONE', #29122 ) ;
#8776=CARTESIAN_POINT ( 'NONE',  ( 136.7023502691896510, 0.000000000000000000, -5.000000000000004441 ) ) ;
#8779=EDGE_LOOP ( 'NONE', ( #23647, #11231, #3878, #15090 ) ) ;
#8783=CARTESIAN_POINT ( 'NONE',  ( 140.5384615384615756, -11.07692307692309264, -4.615384615384626521 ) ) ;
#8784=EDGE_CURVE ( 'NONE', #27945, #23810, #4199, .T. ) ;
#8789=CARTESIAN_POINT ( 'NONE',  ( 141.3750000000000284, 0.000000000000000000, 6.000000000000005329 ) ) ;
#8798=CARTESIAN_POINT ( 'NONE',  ( 150.1726497308104058, -5.000000000000004441, 0.000000000000000000 ) ) ;
#8799=CARTESIAN_POINT ( 'NONE',  ( 160.5863248654052597, 0.000000000000000000, 5.500000000000005329 ) ) ;
#8802=LINE ( 'NONE', #18191, #21160 ) ;
#8803=AXIS2_PLACEMENT_3D ( 'NONE', #18101, #13051, #23861 ) ;
#8808=VERTEX_POINT ( 'NONE', #24832 ) ;
#8809=EDGE_CURVE ( 'NONE', #12588, #22616, #3438, .T. ) ;
#8817=CARTESIAN_POINT ( 'NONE',  ( 147.7500000000000284, -6.000000000000005329, 0.000000000000000000 ) ) ;
#8818=CARTESIAN_POINT ( 'NONE',  ( 160.9999999872065644, -11.61885033700936987, -3.010625523247188351 ) ) ;
#8821=CARTESIAN_POINT ( 'NONE',  ( 139.0312500000000853, -2.485281374238555774, -6.000000000000005329 ) ) ;
#8823=ORIENTED_EDGE ( 'NONE', *, *, #8809, .F. ) ;
#8825=AXIS2_PLACEMENT_3D ( 'NONE', #4474, #2182, #25510 ) ;
#8828=ORIENTED_EDGE ( 'NONE', *, *, #17310, .F. ) ;
#8842=( NAMED_UNIT ( * ) PLANE_ANGLE_UNIT ( ) SI_UNIT ( $, .RADIAN. ) );
#8848=CYLINDRICAL_SURFACE ( 'NONE', #25717, 1.000000000000000888 ) ;
#8855=CARTESIAN_POINT ( 'NONE',  ( 159.0937500000000284, 6.000000000000005329, 2.485281374238585972 ) ) ;
#8859=EDGE_LOOP ( 'NONE', ( #15695, #6854, #28172, #461, #11182 ) ) ;
#8862=VERTEX_POINT ( 'NONE', #10422 ) ;
#8864=( GEOMETRIC_REPRESENTATION_CONTEXT ( 3 ) GLOBAL_UNCERTAINTY_ASSIGNED_CONTEXT ( ( #7211 ) ) GLOBAL_UNIT_ASSIGNED_CONTEXT ( ( #22543, #6703, #15966 ) ) REPRESENTATION_CONTEXT ( 'NONE', 'WORKASPACE' ) );
#8868=DIRECTION ( 'NONE',  ( 0.000000000000000000, 0.8570991287109669399, 0.5151515151515151381 ) ) ;
#8870=CARTESIAN_POINT ( 'NONE',  ( 159.0863248654052597, 0.000000000000000000, 5.500000000000005329 ) ) ;
#8874=CARTESIAN_POINT ( 'NONE',  ( 147.3675748654052029, -5.500000000000012434, 2.278174593052012309 ) ) ;
#8882=CARTESIAN_POINT ( 'NONE',  ( 159.9523502691896510, 0.000000000000000000, 5.000000000000004441 ) ) ;
#8883=CARTESIAN_POINT ( 'NONE',  ( -0.06476833834507110532, -14.68192379133359715, 8.233483135134466835 ) ) ;
#8884=ORIENTED_EDGE ( 'NONE', *, *, #14613, .F. ) ;
#8888=CARTESIAN_POINT ( 'NONE',  ( 161.0439367657379819, 2.138417669162241186, 5.124551926995916773 ) ) ;
#8892=ORIENTED_EDGE ( 'NONE', *, *, #29666, .F. ) ;
#8894=ORIENTED_EDGE ( 'NONE', *, *, #21263, .F. ) ;
#8896=CARTESIAN_POINT ( 'NONE',  ( 158.1562500000000284, -6.000000000000005329, 2.485281374238555774 ) ) ;
#8897=ORIENTED_EDGE ( 'NONE', *, *, #22385, .F. ) ;
#8901=ORIENTED_EDGE ( 'NONE', *, *, #2366, .T. ) ;
#8902=LINE ( 'NONE', #25156, #25352 ) ;
#8905=DIRECTION ( 'NONE',  ( 1.000000000000000000, -0.000000000000000000, -0.000000000000000000 ) ) ;
#8907=DIRECTION ( 'NONE',  ( 0.000000000000000000, 0.000000000000000000, -1.000000000000000000 ) ) ;
#8910=CARTESIAN_POINT ( 'NONE',  ( 125.0000000000000568, -55.00000000000000711, 8.000000000000007105 ) ) ;
#8911=CARTESIAN_POINT ( 'NONE',  ( 159.6672377553881574, -12.19842965096654552, -3.747663857213427541 ) ) ;
#8912=DIRECTION ( 'NONE',  ( 0.000000000000000000, 0.000000000000000000, 1.000000000000000000 ) ) ;
#8917=DIRECTION ( 'NONE',  ( 1.000000000000000000, 6.938893903907222067E-15, 0.000000000000000000 ) ) ;
#8919=DIRECTION ( 'NONE',  ( -1.000000000000000000, 0.000000000000000000, -0.000000000000000000 ) ) ;
#8927=DIRECTION ( 'NONE',  ( 0.000000000000000000, 0.000000000000000000, -1.000000000000000000 ) ) ;
#8928=CARTESIAN_POINT ( 'NONE',  ( 137.5461002691896510, -2.071067811865468400, 4.999999999999989342 ) ) ;
#8935=AXIS2_PLACEMENT_3D ( 'NONE', #24225, #9669, #5027 ) ;
#8938=ORIENTED_EDGE ( 'NONE', *, *, #683, .F. ) ;
#8941=CARTESIAN_POINT ( 'NONE',  ( 141.0000000000000284, 6.000000000000005329, 0.000000000000000000 ) ) ;
#8945=EDGE_CURVE ( 'NONE', #11342, #25384, #9760, .T. ) ;
#8949=CARTESIAN_POINT ( 'NONE',  ( 135.0029060396527996, -6.966976446506110143, -8.000000000000007105 ) ) ;
#8950=CARTESIAN_POINT ( 'NONE',  ( 141.9226497308104342, 5.000000000000004441, 0.000000000000000000 ) ) ;
#8953=CARTESIAN_POINT ( 'NONE',  ( 116.0000000000000142, 6.735557395310442023E-16, 5.500000000000000000 ) ) ;
#8956=EDGE_CURVE ( 'NONE', #13611, #20342, #25753, .T. ) ;
#8957=( BOUNDED_CURVE ( )  B_SPLINE_CURVE ( 2, ( #9629, #21758, #5290, #7460, #19022, #7317, #3138, #14699, #16871 ),
 .UNSPECIFIED., .F., .F. ) 
 B_SPLINE_CURVE_WITH_KNOTS ( ( 3, 2, 2, 2, 3 ),
 ( 0.9375000000000004441, 0.9437500000000003109, 0.9500000000000000666, 0.9562500000000000444, 0.9570852465708525880 ),
 .UNSPECIFIED. ) 
 CURVE ( )  GEOMETRIC_REPRESENTATION_ITEM ( )  RATIONAL_B_SPLINE_CURVE ( ( 0.9999999999999945599, 0.9238795325112921786, 1.000000000000000000, 0.9238795325112867385, 1.000000000000000000, 0.9238795325112867385, 1.000000000000000000, 0.9898273024893375904, 0.9823735524065475566 ) ) 
 REPRESENTATION_ITEM ( '' )  );
#8961=VERTEX_POINT ( 'NONE', #9484 ) ;
#8964=DIRECTION ( 'NONE',  ( 0.000000000000000000, 0.000000000000000000, 1.000000000000000000 ) ) ;
#8969=CARTESIAN_POINT ( 'NONE',  ( 138.0000000000000284, 6.000000000000005329, 0.000000000000000000 ) ) ;
#8970=CARTESIAN_POINT ( 'NONE',  ( 138.8437500000000568, -6.000000000000005329, -2.485281374238555774 ) ) ;
#8989=CARTESIAN_POINT ( 'NONE',  ( -0.8012806810451077455, -9.198719318954825752, 4.013103574300091125 ) ) ;
#8990=CARTESIAN_POINT ( 'NONE',  ( 156.7425748654052029, -2.278174593052183283, -5.499999999999842792 ) ) ;
#8992=FACE_OUTER_BOUND ( 'NONE', #21595, .T. ) ;
#8996=CARTESIAN_POINT ( 'NONE',  ( -4.999999999999886313, -10.00000000000000888, 8.000000000000007105 ) ) ;
#8997=DIRECTION ( 'NONE',  ( 1.000000000000000000, 0.000000000000000000, 0.000000000000000000 ) ) ;
#9000=CARTESIAN_POINT ( 'NONE',  ( 141.0000000000000284, -12.00000000000001066, -4.000000000000003553 ) ) ;
#9005=CARTESIAN_POINT ( 'NONE',  ( 157.8750000000000568, 0.000000000000000000, 6.000000000000005329 ) ) ;
#9009=ORIENTED_EDGE ( 'NONE', *, *, #8693, .T. ) ;
#9016=COLOUR_RGB ( '', 0.08235294, 0.09019608, 0.10196078) ;
#9019=ORIENTED_EDGE ( 'NONE', *, *, #11446, .F. ) ;
#9020=DIRECTION ( 'NONE',  ( 0.000000000000000000, 0.000000000000000000, -1.000000000000000000 ) ) ;
#9022=DIRECTION ( 'NONE',  ( 0.000000000000000000, 1.000000000000000000, -0.000000000000000000 ) ) ;
#9026=SURFACE_SIDE_STYLE ('',( #9635 ) ) ;
#9029=CARTESIAN_POINT ( 'NONE',  ( 159.1086002691896226, -2.071067811865468400, -4.999999999999989342 ) ) ;
#9030=CARTESIAN_POINT ( 'NONE',  ( 0.7577100060955550553, -15.57040985681421219, 7.988286010711783014 ) ) ;
#9031=ORIENTED_EDGE ( 'NONE', *, *, #23349, .F. ) ;
#9038=VERTEX_POINT ( 'NONE', #7012 ) ;
#9041=ORIENTED_EDGE ( 'NONE', *, *, #20256, .T. ) ;
#9044=CARTESIAN_POINT ( 'NONE',  ( 148.4062500000000568, 6.000000000000005329, -2.485281374238555774 ) ) ;
#9045=EDGE_LOOP ( 'NONE', ( #30033, #27066, #21826, #29681 ) ) ;
#9048=EDGE_CURVE ( 'NONE', #18703, #1706, #26243, .T. ) ;
#9054=SURFACE_STYLE_USAGE ( .BOTH. , #29626 ) ;
#9057=DIRECTION ( 'NONE',  ( -0.000000000000000000, -0.5151515151515151381, -0.8570991287109668288 ) ) ;
#9063=CARTESIAN_POINT ( 'NONE',  ( -0.5631067912581171342, -9.873786417483785272, -4.496381089953987775 ) ) ;
#9065=DIRECTION ( 'NONE',  ( 1.000000000000000000, 0.000000000000000000, 0.000000000000000000 ) ) ;
#9067=CARTESIAN_POINT ( 'NONE',  ( 154.3988248654052313, 3.889087296526011706, 3.889087296526011706 ) ) ;
#9076=ADVANCED_FACE ( 'NONE', ( #30052 ), #15518, .F. ) ;
#9081=ORIENTED_EDGE ( 'NONE', *, *, #5378, .T. ) ;
#9083=CARTESIAN_POINT ( 'NONE',  ( 135.5625000000000284, -4.242640687119298093, 4.242640687119298093 ) ) ;
#9089=FILL_AREA_STYLE ('',( #13900 ) ) ;
#9092=CARTESIAN_POINT ( 'NONE',  ( 146.9851497308104342, -3.535533905932725318, 3.535533905932725318 ) ) ;
#9096=CARTESIAN_POINT ( 'NONE',  ( 155.9136751345948539, 0.000000000000000000, -5.500000000000005329 ) ) ;
#9103=FACE_OUTER_BOUND ( 'NONE', #27751, .T. ) ;
#9107=CARTESIAN_POINT ( 'NONE',  ( 125.0000000000000568, -55.00000000000000711, 5.000000000000004441 ) ) ;
#9108=CARTESIAN_POINT ( 'NONE',  ( 13.99999999999999822, 0.000000000000000000, 0.000000000000000000 ) ) ;
#9109=DIRECTION ( 'NONE',  ( -0.000000000000000000, -0.000000000000000000, -1.000000000000000000 ) ) ;
#9112=CARTESIAN_POINT ( 'NONE',  ( 138.6562500000000284, -6.000000000000005329, 2.485281374238556218 ) ) ;
#9113=CARTESIAN_POINT ( 'NONE',  ( 160.8011092498555854, -11.45390509671190493, -3.580702321368915531 ) ) ;
#9115=CARTESIAN_POINT ( 'NONE',  ( 137.0625000000000284, -4.242640687119298093, 4.242640687119298093 ) ) ;
#9118=EDGE_CURVE ( 'NONE', #13233, #2648, #28922, .T. ) ;
#9120=EDGE_LOOP ( 'NONE', ( #28813, #7539, #7402, #2448, #5128, #23856, #5694, #23030, #15889 ) ) ;
#9128=STYLED_ITEM ( 'NONE', ( #14310 ), #7131 ) ;
#9130=CARTESIAN_POINT ( 'NONE',  ( 140.5573082070725093, -11.11461641399627531, -4.524920606408968204 ) ) ;
#9133=CARTESIAN_POINT ( 'NONE',  ( 139.8004524783788725, -8.830548176177012820, -8.125740240671891712 ) ) ;
#9140=CARTESIAN_POINT ( 'NONE',  ( -10.00000000000000178, -89.00000000000001421, 3.000000000000002665 ) ) ;
#9142=CARTESIAN_POINT ( 'NONE',  ( 140.0000000000000284, -9.835770062369604716, 7.609486625086941736 ) ) ;
#9144=DIRECTION ( 'NONE',  ( -1.000000000000000000, -0.000000000000000000, -0.000000000000000000 ) ) ;
#9145=CARTESIAN_POINT ( 'NONE',  ( 156.5625000000000284, -4.242640687119298093, 4.242640687119298093 ) ) ;
#9146=FILL_AREA_STYLE_COLOUR ( '', #6934 ) ;
#9149=EDGE_CURVE ( 'NONE', #12427, #17415, #245, .T. ) ;
#9150=DIRECTION ( 'NONE',  ( 1.000000000000000000, 0.000000000000000000, 0.000000000000000000 ) ) ;
#9153=CARTESIAN_POINT ( 'NONE',  ( 155.1562500000000284, -6.000000000000005329, 2.485281374238555774 ) ) ;
#9169=CARTESIAN_POINT ( 'NONE',  ( 147.1800748654052597, -2.278174593051996322, 5.500000000000026645 ) ) ;
#9171=CIRCLE ( 'NONE', #17523, 10.49999999999999822 ) ;
#9176=CARTESIAN_POINT ( 'NONE',  ( 116.0000000000000142, 0.000000000000000000, -5.500000000000000000 ) ) ;
#9177=CARTESIAN_POINT ( 'NONE',  ( 158.4523502691896510, 0.000000000000000000, 5.000000000000004441 ) ) ;
#9178=CARTESIAN_POINT ( 'NONE',  ( 0.7669223171414714102, -15.58766199952932041, 7.954545454545456806 ) ) ;
#9180=VERTEX_POINT ( 'NONE', #21612 ) ;
#9184=EDGE_CURVE ( 'NONE', #18727, #29595, #26342, .T. ) ;
#9186=CARTESIAN_POINT ( 'NONE',  ( 157.6011751345948255, 3.889087296526011706, -3.889087296526011706 ) ) ;
#9187=EDGE_CURVE ( 'NONE', #22372, #27165, #8957, .T. ) ;
#9189=ORIENTED_EDGE ( 'NONE', *, *, #676, .F. ) ;
#9192=ORIENTED_EDGE ( 'NONE', *, *, #6855, .T. ) ;
#9193=CARTESIAN_POINT ( 'NONE',  ( 148.1250000000000284, 0.000000000000000000, -6.000000000000005329 ) ) ;
#9194=ORIENTED_EDGE ( 'NONE', *, *, #25421, .T. ) ;
#9198=ORIENTED_EDGE ( 'NONE', *, *, #6923, .T. ) ;
#9205=CARTESIAN_POINT ( 'NONE',  ( -19.99999999999998224, -54.99999999999990763, 8.000000000000007105 ) ) ;
#9209=VECTOR ( 'NONE', #14944, 1000.000000000000000 ) ;
#9215=CARTESIAN_POINT ( 'NONE',  ( -38.99999999999998579, -59.99999999999980105, -3.000000000000002665 ) ) ;
#9217=CARTESIAN_POINT ( 'NONE',  ( 160.3062030939346130, -11.25163267815772805, -4.172369835259413406 ) ) ;
#9220=CARTESIAN_POINT ( 'NONE',  ( 135.0586387269457305, -7.769283529832271995, -8.294211448155943245 ) ) ;
#9221=ORIENTED_EDGE ( 'NONE', *, *, #12507, .F. ) ;
#9224=ORIENTED_EDGE ( 'NONE', *, *, #18509, .F. ) ;
#9225=VECTOR ( 'NONE', #121, 1000.000000000000000 ) ;
#9233=CARTESIAN_POINT ( 'NONE',  ( 133.5000000000000284, 6.000000000000005329, 0.000000000000000000 ) ) ;
#9239=CARTESIAN_POINT ( 'NONE',  ( -4.999999999999990230, -24.99999999999999289, 8.000000000000007105 ) ) ;
#9241=CARTESIAN_POINT ( 'NONE',  ( 146.3288997308104342, 4.999999999999989342, -2.071067811865468400 ) ) ;
#9247=CARTESIAN_POINT ( 'NONE',  ( 156.5699251345948255, 2.278174593052198382, 5.499999999999826805 ) ) ;
#9256=ORIENTED_EDGE ( 'NONE', *, *, #14220, .T. ) ;
#9265=CARTESIAN_POINT ( 'NONE',  ( 142.5000000000000568, 6.000000000000005329, 0.000000000000000000 ) ) ;
#9267=DIRECTION ( 'NONE',  ( -1.000000000000000000, -0.000000000000000000, -0.000000000000000000 ) ) ;
#9268=CARTESIAN_POINT ( 'NONE',  ( 133.5937500000000284, 6.000000000000005329, 2.485281374238585972 ) ) ;
#9278=DIRECTION ( 'NONE',  ( 0.000000000000000000, 0.000000000000000000, 1.000000000000000000 ) ) ;
#9279=ADVANCED_FACE ( 'NONE', ( #19891 ), #1748, .F. ) ;
#9294=CARTESIAN_POINT ( 'NONE',  ( 140.0000000000000284, -10.00000000000000888, 7.500000000000007105 ) ) ;
#9295=CARTESIAN_POINT ( 'NONE',  ( 148.7023502691896510, 0.000000000000000000, -5.000000000000004441 ) ) ;
#9297=CARTESIAN_POINT ( 'NONE',  ( -4.999999999999984013, -65.50000000000001421, -8.000000000000007105 ) ) ;
#9298=CARTESIAN_POINT ( 'NONE',  ( 160.2187500000000284, 2.485281374238556218, -6.000000000000005329 ) ) ;
#9299=FILL_AREA_STYLE ('',( #9146 ) ) ;
#9302=DIRECTION ( 'NONE',  ( 0.000000000000000000, 0.000000000000000000, -1.000000000000000000 ) ) ;
#9306=VECTOR ( 'NONE', #13098, 1000.000000000000000 ) ;
#9307=CARTESIAN_POINT ( 'NONE',  ( 151.8750000000000284, 0.000000000000000000, 6.000000000000005329 ) ) ;
#9311=VERTEX_POINT ( 'NONE', #15319 ) ;
#9319=CARTESIAN_POINT ( 'NONE',  ( 155.1413997308104342, 2.071067811865468400, -4.999999999999989342 ) ) ;
#9322=CARTESIAN_POINT ( 'NONE',  ( 159.4613248654052029, -5.500000000000005329, 0.000000000000000000 ) ) ;
#9330=STYLED_ITEM ( 'NONE', ( #25122 ), #943 ) ;
#9332=EDGE_CURVE ( 'NONE', #25088, #25878, #3622, .T. ) ;
#9334=DIRECTION ( 'NONE',  ( 0.000000000000000000, -0.9730085108210397848, -0.2307692307692307265 ) ) ;
#9335=FILL_AREA_STYLE ('',( #20712 ) ) ;
#9336=CARTESIAN_POINT ( 'NONE',  ( 0.1053031288715569197, -15.23283975038563298, 8.619984219653423096 ) ) ;
#9337=VERTEX_POINT ( 'NONE', #5589 ) ;
#9342=CARTESIAN_POINT ( 'NONE',  ( -1.000000000000000888, -19.99999999999998934, 5.000000000000004441 ) ) ;
#9345=LINE ( 'NONE', #25775, #20185 ) ;
#9348=ORIENTED_EDGE ( 'NONE', *, *, #4997, .T. ) ;
#9349=FACE_OUTER_BOUND ( 'NONE', #25331, .T. ) ;
#9350=AXIS2_PLACEMENT_3D ( 'NONE', #27640, #25188, #3998 ) ;
#9351=CARTESIAN_POINT ( 'NONE',  ( 149.3437500000000284, -6.000000000000005329, -2.485281374238555774 ) ) ;
#9363=CARTESIAN_POINT ( 'NONE',  ( 130.0000000000000284, -60.00000000000001421, 3.000000000000002665 ) ) ;
#9367=CARTESIAN_POINT ( 'NONE',  ( -0.02602735246118789356, -9.486986323769393437, -4.738252045315884509 ) ) ;
#9373=CARTESIAN_POINT ( 'NONE',  ( 135.0102241059247774, -7.375790388331942893, -8.398163806897956718 ) ) ;
#9377=CARTESIAN_POINT ( 'NONE',  ( -0.02669168755773660903, -15.33239425769398423, -6.888162703249225416 ) ) ;
#9378=CARTESIAN_POINT ( 'NONE',  ( 143.2574251345948255, -2.278174593051702335, 5.500000000000323297 ) ) ;
#9379=ORIENTED_EDGE ( 'NONE', *, *, #25394, .F. ) ;
#9383=ORIENTED_EDGE ( 'NONE', *, *, #10474, .F. ) ;
#9385=CARTESIAN_POINT ( 'NONE',  ( -4.999999999999886313, -70.00000000000001421, -5.000000000000004441 ) ) ;
#9387=VERTEX_POINT ( 'NONE', #6673 ) ;
#9388=CARTESIAN_POINT ( 'NONE',  ( 151.7738248654052597, -3.889087296526011706, 3.889087296526011706 ) ) ;
#9389=CARTESIAN_POINT ( 'NONE',  ( 138.5625000000000284, -4.242640687119298093, 4.242640687119298093 ) ) ;
#9392=DIRECTION ( 'NONE',  ( 0.000000000000000000, 0.000000000000000000, -1.000000000000000000 ) ) ;
#9393=AXIS2_PLACEMENT_3D ( 'NONE', #26992, #17216, #22569 ) ;
#9394=AXIS2_PLACEMENT_3D ( 'NONE', #16620, #18761, #28672 ) ;
#9402=CARTESIAN_POINT ( 'NONE',  ( 145.4851497308104342, -3.535533905932725318, 3.535533905932725318 ) ) ;
#9404=( GEOMETRIC_REPRESENTATION_CONTEXT ( 3 ) GLOBAL_UNCERTAINTY_ASSIGNED_CONTEXT ( ( #12147 ) ) GLOBAL_UNIT_ASSIGNED_CONTEXT ( ( #28013, #30336, #16555 ) ) REPRESENTATION_CONTEXT ( 'NONE', 'WORKASPACE' ) );
#9410=FACE_OUTER_BOUND ( 'NONE', #17074, .T. ) ;
#9411=DIRECTION ( 'NONE',  ( 0.000000000000000000, 0.000000000000000000, 1.000000000000000000 ) ) ;
#9412=SURFACE_SIDE_STYLE ('',( #11749 ) ) ;
#9414=AXIS2_PLACEMENT_3D ( 'NONE', #15073, #26566, #466 ) ;
#9418=CARTESIAN_POINT ( 'NONE',  ( -0.5000000000000004441, -14.50000000000001243, 8.500000000000007105 ) ) ;
#9419=ORIENTED_EDGE ( 'NONE', *, *, #1575, .F. ) ;
#9421=CARTESIAN_POINT ( 'NONE',  ( 142.0312500000000284, -2.485281374238556218, -6.000000000000005329 ) ) ;
#9423=DIRECTION ( 'NONE',  ( -0.000000000000000000, -1.000000000000000000, 0.000000000000000000 ) ) ;
#9424=CARTESIAN_POINT ( 'NONE',  ( 159.9226497308104058, 5.000000000000004441, 0.000000000000000000 ) ) ;
#9426=ORIENTED_EDGE ( 'NONE', *, *, #25113, .F. ) ;
#9427=AXIS2_PLACEMENT_3D ( 'NONE', #5261, #7426, #2810 ) ;
#9433=AXIS2_PLACEMENT_3D ( 'NONE', #5854, #25057, #27504 ) ;
#9449=AXIS2_PLACEMENT_3D ( 'NONE', #15289, #4029, #13448 ) ;
#9456=CARTESIAN_POINT ( 'NONE',  ( 141.0000000000000284, -54.99999999999989342, -5.000000000000004441 ) ) ;
#9457=CARTESIAN_POINT ( 'NONE',  ( 156.6562500000000284, -6.000000000000005329, 2.485281374238556218 ) ) ;
#9460=CARTESIAN_POINT ( 'NONE',  ( -4.999999999999990230, -55.00000000000002132, -5.000000000000004441 ) ) ;
#9462=DIRECTION ( 'NONE',  ( 0.000000000000000000, 0.000000000000000000, -1.000000000000000000 ) ) ;
#9464=CARTESIAN_POINT ( 'NONE',  ( 151.7812500000000284, 2.485281374238585972, 6.000000000000005329 ) ) ;
#9466=EDGE_CURVE ( 'NONE', #1664, #9581, #20665, .T. ) ;
#9467=CYLINDRICAL_SURFACE ( 'NONE', #21020, 5.500000000000000000 ) ;
#9469=ORIENTED_EDGE ( 'NONE', *, *, #1936, .T. ) ;
#9473=ADVANCED_FACE ( 'NONE', ( #27390 ), #14284, .F. ) ;
#9475=ORIENTED_EDGE ( 'NONE', *, *, #11589, .T. ) ;
#9477=CARTESIAN_POINT ( 'NONE',  ( 157.4851497308104058, -3.535533905932725318, 3.535533905932725318 ) ) ;
#9478=B_SPLINE_CURVE_WITH_KNOTS ( 'NONE', 3,
 ( #19711, #14320, #18608, #11561, #147, #4749, #9217, #1997, #23660, #6904, #2595, #23365, #5035, #11868, #21207, #9676 ),
 .UNSPECIFIED., .F., .F.,
 ( 4, 2, 2, 2, 2, 2, 2, 4 ),
 ( 0.000000000000000000, 0.0007767943629862210809, 0.001165191544479369894, 0.001553588725972518706, 0.001941985907465667736, 0.002330383088958817416, 0.002718780270451967313, 0.003107177451945116776 ),
 .UNSPECIFIED. ) ;
#9481=CARTESIAN_POINT ( 'NONE',  ( 135.0000000000000284, -7.549834435270740940, 7.500000000000007105 ) ) ;
#9484=CARTESIAN_POINT ( 'NONE',  ( 135.0863248654052313, 0.000000000000000000, 5.500000000000005329 ) ) ;
#9489=DIRECTION ( 'NONE',  ( 0.000000000000000000, 0.000000000000000000, 1.000000000000000000 ) ) ;
#9493=CARTESIAN_POINT ( 'NONE',  ( 160.3273502691896510, -5.000000000000004441, 0.000000000000000000 ) ) ;
#9495=VERTEX_POINT ( 'NONE', #25094 ) ;
#9498=DIRECTION ( 'NONE',  ( 0.000000000000000000, 0.000000000000000000, 1.000000000000000000 ) ) ;
#9500=CARTESIAN_POINT ( 'NONE',  ( 157.8824251345948539, 5.500000000000012434, 2.278174593052012309 ) ) ;
#9506=CARTESIAN_POINT ( 'NONE',  ( -9.999999999999793943, 9.000000000000007105, 4.000000000000003553 ) ) ;
#9507=ORIENTED_EDGE ( 'NONE', *, *, #15099, .F. ) ;
#9510=CARTESIAN_POINT ( 'NONE',  ( 152.8125000000000568, 4.242640687119298093, -4.242640687119298093 ) ) ;
#9520=CARTESIAN_POINT ( 'NONE',  ( 133.2038997308104342, 2.071067811865468400, 4.999999999999989342 ) ) ;
#9521=ORIENTED_EDGE ( 'NONE', *, *, #7201, .T. ) ;
#9522=DIRECTION ( 'NONE',  ( -0.000000000000000000, -0.000000000000000000, -1.000000000000000000 ) ) ;
#9527=CARTESIAN_POINT ( 'NONE',  ( -0.9345383689551295392, -9.130923262089551073, -4.000000000000005329 ) ) ;
#9533=FACE_OUTER_BOUND ( 'NONE', #25999, .T. ) ;
#9534=CARTESIAN_POINT ( 'NONE',  ( -1.000000000000000888, -9.000000000000007105, -4.000000000000003553 ) ) ;
#9535=CARTESIAN_POINT ( 'NONE',  ( -0.04562205425674009662, -14.50000000000001243, 8.291335958003937634 ) ) ;
#9537=CARTESIAN_POINT ( 'NONE',  ( 129.9999999999998010, -89.00000000000001421, -4.000000000000003553 ) ) ;
#9541=ADVANCED_FACE ( 'NONE', ( #27692 ), #19183, .F. ) ;
#9544=ORIENTED_EDGE ( 'NONE', *, *, #2523, .F. ) ;
#9546=CARTESIAN_POINT ( 'NONE',  ( 152.2425748654052029, -2.278174593052229469, -5.499999999999796607 ) ) ;
#9547=CARTESIAN_POINT ( 'NONE',  ( 135.4687500000000853, -2.485281374238585972, 6.000000000000005329 ) ) ;
#9554=FACE_OUTER_BOUND ( 'NONE', #6038, .T. ) ;
#9557=CARTESIAN_POINT ( 'NONE',  ( 142.9538997308104058, -2.071067811865468400, -4.999999999999989342 ) ) ;
#9572=CARTESIAN_POINT ( 'NONE',  ( 140.0625000000000284, -4.242640687119298093, 4.242640687119298093 ) ) ;
#9575=CARTESIAN_POINT ( 'NONE',  ( 138.1800748654051745, -2.278174593051950136, 5.500000000000074607 ) ) ;
#9576=ADVANCED_FACE ( 'NONE', ( #28154 ), #23727, .F. ) ;
#9577=CARTESIAN_POINT ( 'NONE',  ( 135.3750000000000284, 0.000000000000000000, 6.000000000000005329 ) ) ;
#9581=VERTEX_POINT ( 'NONE', #14668 ) ;
#9584=AXIS2_PLACEMENT_3D ( 'NONE', #15332, #13189, #20224 ) ;
#9587=CARTESIAN_POINT ( 'NONE',  ( 159.8823591035255731, -12.38010379384060933, -3.486960716177708974 ) ) ;
#9591=DIRECTION ( 'NONE',  ( 1.000000000000000000, -0.000000000000000000, -0.000000000000000000 ) ) ;
#9592=CARTESIAN_POINT ( 'NONE',  ( 135.8363248654052029, 0.000000000000000000, -5.500000000000005329 ) ) ;
#9596=AXIS2_PLACEMENT_3D ( 'NONE', #11575, #20921, #27797 ) ;
#9598=EDGE_CURVE ( 'NONE', #9799, #28361, #25096, .T. ) ;
#9602=FILL_AREA_STYLE_COLOUR ( '', #10918 ) ;
#9603=CARTESIAN_POINT ( 'NONE',  ( 142.9836002691896510, 4.999999999999989342, -2.071067811865468400 ) ) ;
#9605=CARTESIAN_POINT ( 'NONE',  ( 156.1875000000000284, 4.242640687119269671, 4.242640687119298093 ) ) ;
#9607=CIRCLE ( 'NONE', #13564, 16.00000000000000000 ) ;
#9612=ORIENTED_EDGE ( 'NONE', *, *, #26937, .T. ) ;
#9613=CARTESIAN_POINT ( 'NONE',  ( 147.1875000000000284, 4.242640687119269671, 4.242640687119298093 ) ) ;
#9614=CARTESIAN_POINT ( 'NONE',  ( 140.0000000000000284, -11.45643923738959202, 5.000000000000004441 ) ) ;
#9622=CARTESIAN_POINT ( 'NONE',  ( 154.0163997308104342, 4.999999999999989342, 2.071067811865468400 ) ) ;
#9624=( BOUNDED_CURVE ( )  B_SPLINE_CURVE ( 3, ( #25118, #30201, #23160, #6241 ),
 .UNSPECIFIED., .F., .F. ) 
 B_SPLINE_CURVE_WITH_KNOTS ( ( 4, 4 ),
 ( 3.141592653589793116, 4.712388980384689674 ),
 .UNSPECIFIED. ) 
 CURVE ( )  GEOMETRIC_REPRESENTATION_ITEM ( )  RATIONAL_B_SPLINE_CURVE ( ( 1.000000000000000000, 0.8047378541243649375, 0.8047378541243649375, 1.000000000000000000 ) ) 
 REPRESENTATION_ITEM ( '' )  );
#9629=CARTESIAN_POINT ( 'NONE',  ( 160.4136751345948824, 0.000000000000000000, -5.500000000000005329 ) ) ;
#9635=SURFACE_STYLE_FILL_AREA ( #18569 ) ;
#9636=CARTESIAN_POINT ( 'NONE',  ( 145.3199251345948539, -2.278174593052027408, -5.499999999999996447 ) ) ;
#9643=UNCERTAINTY_MEASURE_WITH_UNIT (LENGTH_MEASURE( 1.000000000000000082E-05 ), #14009, 'distance_accuracy_value', 'NONE');
#9649=AXIS2_PLACEMENT_3D ( 'NONE', #18071, #3426, #3888 ) ;
#9654=ORIENTED_EDGE ( 'NONE', *, *, #23025, .F. ) ;
#9655=CARTESIAN_POINT ( 'NONE',  ( 153.0000000000000284, 6.000000000000005329, 0.000000000000000000 ) ) ;
#9658=( GEOMETRIC_REPRESENTATION_CONTEXT ( 3 ) GLOBAL_UNCERTAINTY_ASSIGNED_CONTEXT ( ( #19291 ) ) GLOBAL_UNIT_ASSIGNED_CONTEXT ( ( #16842, #10509, #10211 ) ) REPRESENTATION_CONTEXT ( 'NONE', 'WORKASPACE' ) );
#9661=UNCERTAINTY_MEASURE_WITH_UNIT (LENGTH_MEASURE( 1.000000000000000082E-05 ), #29131, 'distance_accuracy_value', 'NONE');
#9669=DIRECTION ( 'NONE',  ( -0.000000000000000000, -0.000000000000000000, -1.000000000000000000 ) ) ;
#9676=CARTESIAN_POINT ( 'NONE',  ( 161.0000000000000284, -11.67610212985248452, -2.769230769230773603 ) ) ;
#9677=UNCERTAINTY_MEASURE_WITH_UNIT (LENGTH_MEASURE( 1.000000000000000082E-05 ), #14808, 'distance_accuracy_value', 'NONE');
#9679=( BOUNDED_CURVE ( )  B_SPLINE_CURVE ( 2, ( #25328, #9378, #4755, #28090, #4603, #27630, #20910, #20438, #13879 ),
 .UNSPECIFIED., .F., .T. ) 
 B_SPLINE_CURVE_WITH_KNOTS ( ( 3, 2, 2, 2, 3 ),
 ( 0.3624999999999989342, 0.3687499999999991895, 0.3749999999999994449, 0.3812499999999996447, 0.3874999999999999001 ),
 .UNSPECIFIED. ) 
 CURVE ( )  GEOMETRIC_REPRESENTATION_ITEM ( )  RATIONAL_B_SPLINE_CURVE ( ( 1.000000000000013545, 0.9238795325112731938, 1.000000000000000000, 0.9238795325112867385, 1.000000000000000000, 0.9238795325112867385, 1.000000000000000000, 0.9238795325112874046, 0.9999999999999993339 ) ) 
 REPRESENTATION_ITEM ( '' )  );
#9699=CARTESIAN_POINT ( 'NONE',  ( 134.3437500000000568, -6.000000000000005329, -2.485281374238555774 ) ) ;
#9702=FACE_OUTER_BOUND ( 'NONE', #800, .T. ) ;
#9706=AXIS2_PLACEMENT_3D ( 'NONE', #11921, #9267, #27980 ) ;
#9708=CARTESIAN_POINT ( 'NONE',  ( 136.0163997308104626, 4.999999999999989342, 2.071067811865468400 ) ) ;
#9715=EDGE_CURVE ( 'NONE', #9387, #12037, #27044, .T. ) ;
#9716=AXIS2_PLACEMENT_3D ( 'NONE', #22287, #3363, #29638 ) ;
#9717=CYLINDRICAL_SURFACE ( 'NONE', #26917, 5.500000000000000000 ) ;
#9721=CARTESIAN_POINT ( 'NONE',  ( 1.000000000000000888, 2.020667218593133494E-15, 16.50000000000000355 ) ) ;
#9723=ADVANCED_FACE ( 'NONE', ( #12986 ), #27525, .T. ) ;
#9726=EDGE_LOOP ( 'NONE', ( #4985, #24699, #2281, #25776 ) ) ;
#9729=CIRCLE ( 'NONE', #14175, 0.5000000000000004441 ) ;
#9730=CARTESIAN_POINT ( 'NONE',  ( 138.6488248654052313, -3.889087296526011706, -3.889087296526011706 ) ) ;
#9732=AXIS2_PLACEMENT_3D ( 'NONE', #14637, #627, #28270 ) ;
#9733=CARTESIAN_POINT ( 'NONE',  ( 160.7663997308104058, -4.999999999999989342, -2.071067811865468400 ) ) ;
#9737=DIRECTION ( 'NONE',  ( 1.000000000000000000, -0.000000000000000000, -0.000000000000000000 ) ) ;
#9741=CARTESIAN_POINT ( 'NONE',  ( 154.4136751345948539, 0.000000000000000000, -5.500000000000005329 ) ) ;
#9748=DIRECTION ( 'NONE',  ( -3.469446951953694061E-16, -1.000000000000000000, 0.000000000000000000 ) ) ;
#9753=CARTESIAN_POINT ( 'NONE',  ( 144.8586002691896510, 2.071067811865468400, 4.999999999999989342 ) ) ;
#9754=CARTESIAN_POINT ( 'NONE',  ( 160.0000000000000284, -59.99999999999980105, -3.000000000000002665 ) ) ;
#9755=CARTESIAN_POINT ( 'NONE',  ( 158.1562500000000284, -6.000000000000005329, 2.485281374238556218 ) ) ;
#9756=CARTESIAN_POINT ( 'NONE',  ( 135.0000000000000284, -8.662318014469933658, -7.546724076495860523 ) ) ;
#9759=CYLINDRICAL_SURFACE ( 'NONE', #11093, 1.000000000000000000 ) ;
#9760=( BOUNDED_CURVE ( )  B_SPLINE_CURVE ( 2, ( #11823, #18261, #16429, #4243, #4397, #8874, #18867, #9169, #28188 ),
 .UNSPECIFIED., .F., .F. ) 
 B_SPLINE_CURVE_WITH_KNOTS ( ( 3, 2, 2, 2, 3 ),
 ( 0.4625000000000009104, 0.4687500000000006661, 0.4750000000000004219, 0.4812500000000002887, 0.4875000000000000444 ),
 .UNSPECIFIED. ) 
 CURVE ( )  GEOMETRIC_REPRESENTATION_ITEM ( )  RATIONAL_B_SPLINE_CURVE ( ( 0.9999999999999892308, 0.9238795325112975076, 1.000000000000000000, 0.9238795325112867385, 1.000000000000000000, 0.9238795325112867385, 1.000000000000000000, 0.9238795325112860723, 1.000000000000000666 ) ) 
 REPRESENTATION_ITEM ( '' )  );
#9761=ORIENTED_EDGE ( 'NONE', *, *, #683, .T. ) ;
#9762=CARTESIAN_POINT ( 'NONE',  ( 152.5312500000000000, -2.485281374238555774, -6.000000000000005329 ) ) ;
#9771=ORIENTED_EDGE ( 'NONE', *, *, #29842, .F. ) ;
#9775=DIRECTION ( 'NONE',  ( -1.000000000000000000, -6.938893903907222067E-15, 0.000000000000000000 ) ) ;
#9776=CARTESIAN_POINT ( 'NONE',  ( 155.4226497308104058, 5.000000000000004441, 0.000000000000000000 ) ) ;
#9777=LINE ( 'NONE', #26187, #29424 ) ;
#9779=CARTESIAN_POINT ( 'NONE',  ( 140.5000000000000284, -10.99818166789400919, 4.800000000000004263 ) ) ;
#9785=STYLED_ITEM ( 'NONE', ( #4429 ), #25177 ) ;
#9787=DIRECTION ( 'NONE',  ( 0.000000000000000000, 0.000000000000000000, 1.000000000000000000 ) ) ;
#9793=FACE_OUTER_BOUND ( 'NONE', #4509, .T. ) ;
#9797=CARTESIAN_POINT ( 'NONE',  ( -0.04562205425674009662, -14.50000000000001243, -8.291335958003937634 ) ) ;
#9799=VERTEX_POINT ( 'NONE', #3248 ) ;
#9801=CARTESIAN_POINT ( 'NONE',  ( 146.9062500000000284, 6.000000000000005329, -2.485281374238555774 ) ) ;
#9812=COLOUR_RGB ( '', 0.31764706, 0.68627451, 0.89019608) ;
#9813=SURFACE_STYLE_FILL_AREA ( #26374 ) ;
#9814=VERTEX_POINT ( 'NONE', #949 ) ;
#9815=EDGE_CURVE ( 'NONE', #17555, #25961, #9478, .T. ) ;
#9816=CARTESIAN_POINT ( 'NONE',  ( 158.8199251345948824, -2.278174593051888408, -5.500000000000135891 ) ) ;
#9827=ORIENTED_EDGE ( 'NONE', *, *, #29732, .T. ) ;
#9829=CARTESIAN_POINT ( 'NONE',  ( -0.004068020306998300362, -15.42148939562913945, -6.273618375958268878 ) ) ;
#9830=AXIS2_PLACEMENT_3D ( 'NONE', #25968, #7671, #9392 ) ;
#9833=ORIENTED_EDGE ( 'NONE', *, *, #15571, .F. ) ;
#9836=FILL_AREA_STYLE_COLOUR ( '', #17565 ) ;
#9838=CARTESIAN_POINT ( 'NONE',  ( -20.99999999999998224, -54.99999999999990763, -5.000000000000004441 ) ) ;
#9839=VERTEX_POINT ( 'NONE', #16471 ) ;
#9840=ORIENTED_EDGE ( 'NONE', *, *, #25544, .T. ) ;
#9841=CARTESIAN_POINT ( 'NONE',  ( 132.5625000000000284, -4.242640687119298093, 4.242640687119298093 ) ) ;
#9842=CARTESIAN_POINT ( 'NONE',  ( 162.0000000000000284, 6.000000000000005329, 0.000000000000000000 ) ) ;
#9843=EDGE_CURVE ( 'NONE', #28330, #18627, #12015, .T. ) ;
#9848=DIRECTION ( 'NONE',  ( 0.000000000000000000, 0.000000000000000000, -1.000000000000000000 ) ) ;
#9850=CARTESIAN_POINT ( 'NONE',  ( 161.0000000000000284, 0.000000000000000000, 0.000000000000000000 ) ) ;
#9851=AXIS2_PLACEMENT_3D ( 'NONE', #24408, #29152, #8112 ) ;
#9852=VERTEX_POINT ( 'NONE', #28382 ) ;
#9858=EDGE_CURVE ( 'NONE', #4225, #30104, #6937, .T. ) ;
#9860=CARTESIAN_POINT ( 'NONE',  ( 140.9851497308104058, -3.535533905932725318, 3.535533905932725318 ) ) ;
#9863=CYLINDRICAL_SURFACE ( 'NONE', #8669, 5.500000000000000000 ) ;
#9869=CARTESIAN_POINT ( 'NONE',  ( -0.5000000000000004441, -9.500000000000008882, 8.000000000000007105 ) ) ;
#9870=CARTESIAN_POINT ( 'NONE',  ( 153.8511751345948539, -3.889087296526011706, 3.889087296526011706 ) ) ;
#9875=CARTESIAN_POINT ( 'NONE',  ( 136.3125000000000284, 4.242640687119298093, -4.242640687119298093 ) ) ;
#9879=CARTESIAN_POINT ( 'NONE',  ( 160.4851497308104058, -3.535533905932725318, 3.535533905932725318 ) ) ;
#9883=EDGE_CURVE ( 'NONE', #5798, #23261, #2062, .T. ) ;
#9885=ORIENTED_EDGE ( 'NONE', *, *, #19488, .F. ) ;
#9897=AXIS2_PLACEMENT_3D ( 'NONE', #8083, #17810, #17351 ) ;
#9903=CARTESIAN_POINT ( 'NONE',  ( 139.6949251345948255, 5.500000000000012434, -2.278174593052012309 ) ) ;
#9906=FACE_OUTER_BOUND ( 'NONE', #24079, .T. ) ;
#9907=CARTESIAN_POINT ( 'NONE',  ( 145.9836002691896510, 4.999999999999989342, -2.071067811865468400 ) ) ;
#9908=CARTESIAN_POINT ( 'NONE',  ( 154.5937500000000284, 6.000000000000005329, 2.485281374238585972 ) ) ;
#9914=CARTESIAN_POINT ( 'NONE',  ( 150.0937500000000284, 6.000000000000005329, 2.485281374238585972 ) ) ;
#9916=( GEOMETRIC_REPRESENTATION_CONTEXT ( 3 ) GLOBAL_UNCERTAINTY_ASSIGNED_CONTEXT ( ( #26321 ) ) GLOBAL_UNIT_ASSIGNED_CONTEXT ( ( #12459, #19502, #28834 ) ) REPRESENTATION_CONTEXT ( 'NONE', 'WORKASPACE' ) );
#9923=ORIENTED_EDGE ( 'NONE', *, *, #7373, .T. ) ;
#9927=CARTESIAN_POINT ( 'NONE',  ( 139.5000000000000284, -54.99999999999990763, -7.500000000000007105 ) ) ;
#9930=CYLINDRICAL_SURFACE ( 'NONE', #15219, 5.500000000000000000 ) ;
#9934=DIRECTION ( 'NONE',  ( 0.000000000000000000, -1.000000000000000000, 0.000000000000000000 ) ) ;
#9936=DIRECTION ( 'NONE',  ( 0.000000000000000000, 0.000000000000000000, 1.000000000000000000 ) ) ;
#9942=CARTESIAN_POINT ( 'NONE',  ( 135.0863248654052313, 0.000000000000000000, 5.500000000000005329 ) ) ;
#9952=EDGE_LOOP ( 'NONE', ( #23677, #28860, #24374, #28680 ) ) ;
#9953=EDGE_CURVE ( 'NONE', #12660, #9038, #22260, .T. ) ;
#9955=ORIENTED_EDGE ( 'NONE', *, *, #7383, .F. ) ;
#9964=CARTESIAN_POINT ( 'NONE',  ( 132.5476497308104058, 0.000000000000000000, -5.000000000000004441 ) ) ;
#9968=CARTESIAN_POINT ( 'NONE',  ( 158.1636751345948255, 0.000000000000000000, 5.500000000000005329 ) ) ;
#9969=CARTESIAN_POINT ( 'NONE',  ( 141.8363248654052029, 0.000000000000000000, -5.500000000000005329 ) ) ;
#9972=CARTESIAN_POINT ( 'NONE',  ( 0.000000000000000000, -14.26420856792215552, 8.432299132049415391 ) ) ;
#9974=DIRECTION ( 'NONE',  ( 0.000000000000000000, 1.224646799147353454E-16, 1.000000000000000000 ) ) ;
#9977=CARTESIAN_POINT ( 'NONE',  ( 135.8074773656872765, -8.774755822434132213, 8.164331751096858270 ) ) ;
#9979=DIRECTION ( 'NONE',  ( -6.938893903907222067E-15, -1.000000000000000000, 0.000000000000000000 ) ) ;
#9983=EDGE_CURVE ( 'NONE', #3651, #2002, #12433, .T. ) ;
#9984=CARTESIAN_POINT ( 'NONE',  ( 0.9867564579130563285, -16.18227523715626504, 6.671628312105942982 ) ) ;
#9986=ORIENTED_EDGE ( 'NONE', *, *, #14649, .F. ) ;
#9987=DIRECTION ( 'NONE',  ( 0.000000000000000000, 0.000000000000000000, 1.000000000000000000 ) ) ;
#9989=AXIS2_PLACEMENT_3D ( 'NONE', #22637, #29207, #3560 ) ;
#9997=CARTESIAN_POINT ( 'NONE',  ( 132.6711002691896795, 4.999999999999989342, 2.071067811865468400 ) ) ;
#9999=DIRECTION ( 'NONE',  ( 0.000000000000000000, 0.000000000000000000, -1.000000000000000000 ) ) ;
#10003=CARTESIAN_POINT ( 'NONE',  ( 144.2886751345948539, 5.500000000000005329, 0.000000000000000000 ) ) ;
#10006=DIRECTION ( 'NONE',  ( 0.000000000000000000, 0.000000000000000000, 1.000000000000000000 ) ) ;
#10008=CARTESIAN_POINT ( 'NONE',  ( 139.0163997308104342, 4.999999999999989342, 2.071067811865468400 ) ) ;
#10010=CARTESIAN_POINT ( 'NONE',  ( 0.000000000000000000, -14.50000000000001243, 8.000000000000007105 ) ) ;
#10011=CIRCLE ( 'NONE', #17881, 15.00000000000000000 ) ;
#10017=ADVANCED_FACE ( 'NONE', ( #24387 ), #19201, .F. ) ;
#10020=CARTESIAN_POINT ( 'NONE',  ( 153.5550748654052029, -5.500000000000012434, -2.278174593052012309 ) ) ;
#10021=ORIENTED_EDGE ( 'NONE', *, *, #11941, .F. ) ;
#10026=( NAMED_UNIT ( * ) PLANE_ANGLE_UNIT ( ) SI_UNIT ( $, .RADIAN. ) );
#10028=( BOUNDED_CURVE ( )  B_SPLINE_CURVE ( 2, ( #23326, #1796, #20390, #11363, #13362, #2116, #6716, #11202, #22707 ),
 .UNSPECIFIED., .F., .T. ) 
 B_SPLINE_CURVE_WITH_KNOTS ( ( 3, 2, 2, 2, 3 ),
 ( 0.5125000000000009548, 0.5187500000000008216, 0.5250000000000005773, 0.5312500000000002220, 0.5374999999999999778 ),
 .UNSPECIFIED. ) 
 CURVE ( )  GEOMETRIC_REPRESENTATION_ITEM ( )  RATIONAL_B_SPLINE_CURVE ( ( 0.9999999999999877875, 0.9238795325112989509, 1.000000000000000000, 0.9238795325112867385, 1.000000000000000000, 0.9238795325112867385, 1.000000000000000000, 0.9238795325112867385, 1.000000000000000000 ) ) 
 REPRESENTATION_ITEM ( '' )  );
#10031=CIRCLE ( 'NONE', #27178, 16.00000000000000000 ) ;
#10039=SURFACE_STYLE_FILL_AREA ( #2404 ) ;
#10042=CYLINDRICAL_SURFACE ( 'NONE', #2020, 0.5000000000000004441 ) ;
#10044=DIRECTION ( 'NONE',  ( -1.000000000000000000, -0.000000000000000000, 0.000000000000000000 ) ) ;
#10047=CARTESIAN_POINT ( 'NONE',  ( 140.3314506832066400, -9.164856574046146065, 7.747256842543193578 ) ) ;
#10051=EDGE_CURVE ( 'NONE', #26257, #42, #5335, .T. ) ;
#10052=AXIS2_PLACEMENT_3D ( 'NONE', #21271, #21125, #64 ) ;
#10058=CARTESIAN_POINT ( 'NONE',  ( 144.2023502691896510, 0.000000000000000000, -5.000000000000004441 ) ) ;
#10059=CARTESIAN_POINT ( 'NONE',  ( 149.8125000000000568, 4.242640687119298093, -4.242640687119298093 ) ) ;
#10064=EDGE_CURVE ( 'NONE', #25253, #22372, #28566, .T. ) ;
#10068=CARTESIAN_POINT ( 'NONE',  ( 146.8125000000000284, 4.242640687119298093, -4.242640687119298093 ) ) ;
#10073=ORIENTED_EDGE ( 'NONE', *, *, #6322, .T. ) ;
#10076=ORIENTED_EDGE ( 'NONE', *, *, #3639, .F. ) ;
#10077=COLOUR_RGB ( '', 0.66274510, 0.83137255, 0.94901961) ;
#10082=FACE_OUTER_BOUND ( 'NONE', #22835, .T. ) ;
#10085=CARTESIAN_POINT ( 'NONE',  ( 143.9925748654052313, 2.278174593052043395, 5.499999999999981348 ) ) ;
#10095=DIRECTION ( 'NONE',  ( 1.000000000000000000, -0.000000000000000000, -0.000000000000000000 ) ) ;
#10096=LINE ( 'NONE', #19033, #20428 ) ;
#10098=DIRECTION ( 'NONE',  ( 1.000000000000000000, 0.000000000000000000, 0.000000000000000000 ) ) ;
#10099=DIRECTION ( 'NONE',  ( -1.000000000000000000, -6.938893903907221278E-15, -0.000000000000000000 ) ) ;
#10101=AXIS2_PLACEMENT_3D ( 'NONE', #23945, #874, #7783 ) ;
#10106=CARTESIAN_POINT ( 'NONE',  ( 145.1250000000000284, 0.000000000000000000, -6.000000000000005329 ) ) ;
#10108=CIRCLE ( 'NONE', #10620, 0.5000000000000004441 ) ;
#10112=ORIENTED_EDGE ( 'NONE', *, *, #24317, .T. ) ;
#10116=CARTESIAN_POINT ( 'NONE',  ( 132.3601497308104342, -3.535533905932725318, -3.535533905932725318 ) ) ;
#10119=CARTESIAN_POINT ( 'NONE',  ( 0.1053031288715393921, -15.23283975038561344, -8.619984219653437307 ) ) ;
#10121=CARTESIAN_POINT ( 'NONE',  ( 158.3511751345948539, -3.889087296526011706, 3.889087296526011706 ) ) ;
#10122=SURFACE_SIDE_STYLE ('',( #19059 ) ) ;
#10125=AXIS2_PLACEMENT_3D ( 'NONE', #22102, #10902, #17969 ) ;
#10128=DIRECTION ( 'NONE',  ( -1.000000000000000000, 0.000000000000000000, 0.000000000000000000 ) ) ;
#10130=EDGE_CURVE ( 'NONE', #25655, #1053, #18362, .T. ) ;
#10135=CARTESIAN_POINT ( 'NONE',  ( -9.999999999999980460, -60.00000000000001421, -3.000000000000002665 ) ) ;
#10136=ORIENTED_EDGE ( 'NONE', *, *, #25014, .F. ) ;
#10142=SURFACE_STYLE_FILL_AREA ( #756 ) ;
#10144=ORIENTED_EDGE ( 'NONE', *, *, #18958, .T. ) ;
#10148=CARTESIAN_POINT ( 'NONE',  ( 132.1875000000000284, 4.242640687119269671, 4.242640687119298093 ) ) ;
#10149=CARTESIAN_POINT ( 'NONE',  ( 135.2023502691896510, 0.000000000000000000, -5.000000000000004441 ) ) ;
#10158=CARTESIAN_POINT ( 'NONE',  ( 138.7351497308104058, 3.535533905932725318, -3.535533905932725318 ) ) ;
#10159=CARTESIAN_POINT ( 'NONE',  ( 137.5238248654052029, 3.889087296526011706, -3.889087296526011706 ) ) ;
#10164=DIRECTION ( 'NONE',  ( -3.469446951953694061E-16, -1.000000000000000000, 0.000000000000000000 ) ) ;
#10165=AXIS2_PLACEMENT_3D ( 'NONE', #17288, #18052, #20020 ) ;
#10166=AXIS2_PLACEMENT_3D ( 'NONE', #4142, #20599, #27935 ) ;
#10169=CARTESIAN_POINT ( 'NONE',  ( -19.49999999999998224, -25.00000000000010658, 8.000000000000007105 ) ) ;
#10170=MECHANICAL_DESIGN_GEOMETRIC_PRESENTATION_REPRESENTATION('',(#12176),#29766);
#10171=ORIENTED_EDGE ( 'NONE', *, *, #16267, .T. ) ;
#10174=ORIENTED_EDGE ( 'NONE', *, *, #28278, .F. ) ;
#10185=EDGE_CURVE ( 'NONE', #24857, #2252, #30103, .T. ) ;
#10186=ORIENTED_EDGE ( 'NONE', *, *, #15779, .F. ) ;
#10190=CARTESIAN_POINT ( 'NONE',  ( 159.0074251345947971, 2.278174593052136210, -5.499999999999888978 ) ) ;
#10192=DIRECTION ( 'NONE',  ( -0.000000000000000000, -0.000000000000000000, -1.000000000000000000 ) ) ;
#10194=FACE_OUTER_BOUND ( 'NONE', #25741, .T. ) ;
#10198=CYLINDRICAL_SURFACE ( 'NONE', #27349, 5.500000000000000000 ) ;
#10200=EDGE_CURVE ( 'NONE', #4935, #10891, #22247, .T. ) ;
#10205=( NAMED_UNIT ( * ) PLANE_ANGLE_UNIT ( ) SI_UNIT ( $, .RADIAN. ) );
#10208=CARTESIAN_POINT ( 'NONE',  ( 145.3050748654052029, 5.500000000000012434, 2.278174593052012309 ) ) ;
#10211=( NAMED_UNIT ( * ) SI_UNIT ( $, .STERADIAN. ) SOLID_ANGLE_UNIT ( ) );
#10212=EDGE_LOOP ( 'NONE', ( #14967, #26106, #4686, #8644 ) ) ;
#10213=CARTESIAN_POINT ( 'NONE',  ( 138.5773502691896510, 5.000000000000004441, 0.000000000000000000 ) ) ;
#10214=CARTESIAN_POINT ( 'NONE',  ( 154.6875000000000284, 4.242640687119269671, 4.242640687119298093 ) ) ;
#10215=CARTESIAN_POINT ( 'NONE',  ( 135.0000000000000284, -7.311352623425150909, -8.296311145640547835 ) ) ;
#10220=ORIENTED_EDGE ( 'NONE', *, *, #17696, .T. ) ;
#10221=CARTESIAN_POINT ( 'NONE',  ( 141.7500000000000568, -6.000000000000005329, 0.000000000000000000 ) ) ;
#10222=VECTOR ( 'NONE', #3153, 1000.000000000000000 ) ;
#10227=FILL_AREA_STYLE ('',( #831 ) ) ;
#10233=DIRECTION ( 'NONE',  ( 1.000000000000000000, 0.000000000000000000, 0.000000000000000000 ) ) ;
#10235=( LENGTH_UNIT ( ) NAMED_UNIT ( * ) SI_UNIT ( .MILLI., .METRE. ) );
#10240=CARTESIAN_POINT ( 'NONE',  ( 143.4300748654052029, 2.278174593051733421, -5.500000000000292211 ) ) ;
#10242=LINE ( 'NONE', #19601, #22305 ) ;
#10243=CARTESIAN_POINT ( 'NONE',  ( 148.8675748654052029, -5.500000000000012434, 2.278174593052012309 ) ) ;
#10244=B_SPLINE_CURVE_WITH_KNOTS ( 'NONE', 3,
 ( #24818, #15169, #1624, #10553, #12730, #8537 ),
 .UNSPECIFIED., .F., .F.,
 ( 4, 2, 4 ),
 ( 0.000000000000000000, 0.0009324921843552346802, 0.001864984368710469360 ),
 .UNSPECIFIED. ) ;
#10259=ADVANCED_FACE ( 'NONE', ( #27736 ), #11829, .F. ) ;
#10263=ORIENTED_EDGE ( 'NONE', *, *, #25014, .T. ) ;
#10268=VERTEX_POINT ( 'NONE', #107 ) ;
#10269=CARTESIAN_POINT ( 'NONE',  ( -0.05510817352033407085, -14.57581869335689007, -8.269855266334088739 ) ) ;
#10276=DIRECTION ( 'NONE',  ( 0.000000000000000000, 0.000000000000000000, 1.000000000000000000 ) ) ;
#10281=CARTESIAN_POINT ( 'NONE',  ( 159.6636751345948539, 0.000000000000000000, 5.500000000000005329 ) ) ;
#10283=CARTESIAN_POINT ( 'NONE',  ( 149.0699251345948539, 2.278174593052259667, 5.499999999999763745 ) ) ;
#10284=EDGE_LOOP ( 'NONE', ( #21771, #4983, #5159, #7196 ) ) ;
#10285=CARTESIAN_POINT ( 'NONE',  ( 135.2246127425879081, -8.380956232050152721, -8.129726081524356829 ) ) ;
#10289=CIRCLE ( 'NONE', #29871, 0.9999999999999995559 ) ;
#10291=DIRECTION ( 'NONE',  ( 0.000000000000000000, 0.000000000000000000, 1.000000000000000000 ) ) ;
#10295=CARTESIAN_POINT ( 'NONE',  ( 136.0461002691896795, -2.071067811865468400, 4.999999999999989342 ) ) ;
#10296=ADVANCED_FACE ( 'NONE', ( #16131 ), #6864, .F. ) ;
#10299=ORIENTED_EDGE ( 'NONE', *, *, #8019, .T. ) ;
#10301=DIRECTION ( 'NONE',  ( -1.000000000000000000, -0.000000000000000000, -0.000000000000000000 ) ) ;
#10303=ORIENTED_EDGE ( 'NONE', *, *, #7435, .T. ) ;
#10307=CARTESIAN_POINT ( 'NONE',  ( 139.4851497308104058, -3.535533905932725318, 3.535533905932725318 ) ) ;
#10308=CARTESIAN_POINT ( 'NONE',  ( 137.6175748654052597, 5.500000000000012434, -2.278174593052012309 ) ) ;
#10316=STYLED_ITEM ( 'NONE', ( #19733 ), #16057 ) ;
#10317=EDGE_LOOP ( 'NONE', ( #13545, #9041 ) ) ;
#10319=COLOUR_RGB ( '', 0.66274510, 0.83137255, 0.94901961) ;
#10321=DIRECTION ( 'NONE',  ( -1.000000000000000000, -1.067522139062651904E-16, 0.000000000000000000 ) ) ;
#10322=CYLINDRICAL_SURFACE ( 'NONE', #13950, 30.00000000000000000 ) ;
#10323=DIRECTION ( 'NONE',  ( 6.938893903907221278E-15, -1.000000000000000000, 0.000000000000000000 ) ) ;
#10324=ORIENTED_EDGE ( 'NONE', *, *, #6809, .F. ) ;
#10326=CARTESIAN_POINT ( 'NONE',  ( 135.0937500000000284, 5.999999999999970690, 2.485281374238619723 ) ) ;
#10336=AXIS2_PLACEMENT_3D ( 'NONE', #20207, #27238, #13318 ) ;
#10341=( NAMED_UNIT ( * ) PLANE_ANGLE_UNIT ( ) SI_UNIT ( $, .RADIAN. ) );
#10343=DIRECTION ( 'NONE',  ( 0.000000000000000000, 0.000000000000000000, -1.000000000000000000 ) ) ;
#10344=CARTESIAN_POINT ( 'NONE',  ( 156.8288997308103774, 4.999999999999989342, -2.071067811865468400 ) ) ;
#10352=CARTESIAN_POINT ( 'NONE',  ( 147.0863248654052313, 0.000000000000000000, 5.500000000000005329 ) ) ;
#10358=CARTESIAN_POINT ( 'NONE',  ( 138.0148502691896510, -3.535533905932725318, -3.535533905932725318 ) ) ;
#10359=VECTOR ( 'NONE', #1465, 1000.000000000000000 ) ;
#10360=CARTESIAN_POINT ( 'NONE',  ( 153.1875000000000284, 4.242640687119269671, 4.242640687119298093 ) ) ;
#10363=EDGE_CURVE ( 'NONE', #8247, #17248, #22501, .T. ) ;
#10366=CARTESIAN_POINT ( 'NONE',  ( 145.7812500000000284, 2.485281374238585972, 6.000000000000005329 ) ) ;
#10368=CIRCLE ( 'NONE', #10387, 29.00000000000000000 ) ;
#10380=SURFACE_STYLE_USAGE ( .BOTH. , #22043 ) ;
#10383=FACE_OUTER_BOUND ( 'NONE', #1020, .T. ) ;
#10387=AXIS2_PLACEMENT_3D ( 'NONE', #17251, #14934, #6911 ) ;
#10389=CARTESIAN_POINT ( 'NONE',  ( 135.0000000000000000, 4.598116130853834527, 3.436179909522558251 ) ) ;
#10391=AXIS2_PLACEMENT_3D ( 'NONE', #10825, #3556, #26897 ) ;
#10395=LINE ( 'NONE', #3000, #18773 ) ;
#10397=CARTESIAN_POINT ( 'NONE',  ( 0.8631338372297875372, -15.37878787878788067, 8.351220472436777342 ) ) ;
#10399=ADVANCED_FACE ( 'NONE', ( #15635 ), #27098, .T. ) ;
#10403=CARTESIAN_POINT ( 'NONE',  ( 159.2812500000000568, 2.485281374238585972, 6.000000000000005329 ) ) ;
#10410=VERTEX_POINT ( 'NONE', #24488 ) ;
#10415=CARTESIAN_POINT ( 'NONE',  ( 159.6636751345948539, 0.000000000000000000, 5.500000000000005329 ) ) ;
#10420=CARTESIAN_POINT ( 'NONE',  ( 0.1257737839961825255, -15.26928397096460266, -8.555325078616231593 ) ) ;
#10422=CARTESIAN_POINT ( 'NONE',  ( 13.99999999999999822, 2.143131898507868643E-15, -17.50000000000000355 ) ) ;
#10426=CIRCLE ( 'NONE', #19269, 17.50000000000000355 ) ;
#10427=CARTESIAN_POINT ( 'NONE',  ( 152.6175748654052029, 5.500000000000012434, -2.278174593052012309 ) ) ;
#10429=B_SPLINE_CURVE_WITH_KNOTS ( 'NONE', 3,
 ( #27009, #19808, #26410, #17378 ),
 .UNSPECIFIED., .F., .F.,
 ( 4, 4 ),
 ( 0.000000000000000000, 0.0005217984816236547699 ),
 .UNSPECIFIED. ) ;
#10430=CARTESIAN_POINT ( 'NONE',  ( -0.6001665993698097612, -9.799666801260405791, 4.385453238887307315 ) ) ;
#10433=CARTESIAN_POINT ( 'NONE',  ( 135.0000000000000284, -6.982120021884474781, 8.500000000000007105 ) ) ;
#10436=ORIENTED_EDGE ( 'NONE', *, *, #26499, .F. ) ;
#10438=EDGE_CURVE ( 'NONE', #11662, #4075, #2134, .T. ) ;
#10440=ORIENTED_EDGE ( 'NONE', *, *, #30191, .T. ) ;
#10443=DIRECTION ( 'NONE',  ( 1.000000000000000000, -0.000000000000000000, -0.000000000000000000 ) ) ;
#10446=DIRECTION ( 'NONE',  ( 6.938893903907221278E-15, 1.000000000000000000, -0.000000000000000000 ) ) ;
#10447=VERTEX_POINT ( 'NONE', #25719 ) ;
#10448=ORIENTED_EDGE ( 'NONE', *, *, #26299, .F. ) ;
#10449=CARTESIAN_POINT ( 'NONE',  ( 135.4836002691896510, 4.999999999999989342, -2.071067811865468400 ) ) ;
#10455=DIRECTION ( 'NONE',  ( 0.000000000000000000, 0.000000000000000000, 1.000000000000000000 ) ) ;
#10458=CARTESIAN_POINT ( 'NONE',  ( 0.9172299446477815144, -15.89788423467024181, -7.323522863575444575 ) ) ;
#10459=CARTESIAN_POINT ( 'NONE',  ( 149.4449251345948539, -5.500000000000012434, 2.278174593052012309 ) ) ;
#10461=CARTESIAN_POINT ( 'NONE',  ( 139.5863248654052313, 0.000000000000000000, 5.500000000000005329 ) ) ;
#10462=CARTESIAN_POINT ( 'NONE',  ( 8.673617379884035472E-16, -14.99923475244192339, -9.015151515151522688 ) ) ;
#10465=DIRECTION ( 'NONE',  ( 1.000000000000000000, -0.000000000000000000, -0.000000000000000000 ) ) ;
#10466=CARTESIAN_POINT ( 'NONE',  ( 135.0000000000000000, 3.026753582206697324, 4.706811043600045430 ) ) ;
#10468=CARTESIAN_POINT ( 'NONE',  ( -15.49999999999999289, -54.99999999999990763, -7.500000000000007105 ) ) ;
#10470=TOROIDAL_SURFACE ( 'NONE', #7988, 2.000000000000000000, 1.000000000000000000 ) ;
#10472=EDGE_LOOP ( 'NONE', ( #19217, #17329, #30253, #28552 ) ) ;
#10473=LINE ( 'NONE', #15411, #12204 ) ;
#10474=EDGE_CURVE ( 'NONE', #20437, #9337, #29741, .T. ) ;
#10476=CARTESIAN_POINT ( 'NONE',  ( 153.7425748654052029, -2.278174593052213481, -5.499999999999811706 ) ) ;
#10488=DIRECTION ( 'NONE',  ( 1.000000000000000000, -0.000000000000000000, -0.000000000000000000 ) ) ;
#10490=CARTESIAN_POINT ( 'NONE',  ( 140.5573082070725377, -11.11461641399629663, 4.524920606408917578 ) ) ;
#10491=ORIENTED_EDGE ( 'NONE', *, *, #17559, .F. ) ;
#10493=CARTESIAN_POINT ( 'NONE',  ( 161.0000000000000568, -11.64610661123979440, 2.895702980449532227 ) ) ;
#10497=CARTESIAN_POINT ( 'NONE',  ( 150.5476497308104058, 0.000000000000000000, -5.000000000000004441 ) ) ;
#10500=PRESENTATION_STYLE_ASSIGNMENT (( #19852 ) ) ;
#10501=CARTESIAN_POINT ( 'NONE',  ( 135.1658987231415097, -8.213333715523679857, 8.175427762257710285 ) ) ;
#10509=( NAMED_UNIT ( * ) PLANE_ANGLE_UNIT ( ) SI_UNIT ( $, .RADIAN. ) );
#10511=CARTESIAN_POINT ( 'NONE',  ( 151.7812500000000284, 2.485281374238585972, 6.000000000000005329 ) ) ;
#10514=STYLED_ITEM ( 'NONE', ( #3847 ), #9 ) ;
#10517=ORIENTED_EDGE ( 'NONE', *, *, #18961, .F. ) ;
#10518=CARTESIAN_POINT ( 'NONE',  ( 143.3437500000000284, -6.000000000000005329, -2.485281374238555774 ) ) ;
#10519=CARTESIAN_POINT ( 'NONE',  ( 161.2977071193381846, -5.560427160162643823, 1.671920971621268182 ) ) ;
#10529=CARTESIAN_POINT ( 'NONE',  ( -19.99999999999998224, -54.99999999999990763, -5.000000000000004441 ) ) ;
#10530=ADVANCED_FACE ( 'NONE', ( #953 ), #23247, .T. ) ;
#10533=LINE ( 'NONE', #3889, #30393 ) ;
#10539=CARTESIAN_POINT ( 'NONE',  ( 135.0000000000000000, 5.980918879946599098, 0.2920434870148253537 ) ) ;
#10545=CARTESIAN_POINT ( 'NONE',  ( 152.6398502691896510, -3.535533905932752852, 3.535533905932725318 ) ) ;
#10546=CARTESIAN_POINT ( 'NONE',  ( 161.1742592625232930, -5.078550059815297502, -2.565790349115546931 ) ) ;
#10552=CARTESIAN_POINT ( 'NONE',  ( 161.8125000000000284, 4.242640687119298093, -4.242640687119298093 ) ) ;
#10553=CARTESIAN_POINT ( 'NONE',  ( -0.02670840214258772202, -15.33233796376583946, 6.888541525869519511 ) ) ;
#10561=CARTESIAN_POINT ( 'NONE',  ( 160.0000000000000284, -11.67610212985248097, 2.769230769230771827 ) ) ;
#10572=ORIENTED_EDGE ( 'NONE', *, *, #20324, .T. ) ;
#10581=CARTESIAN_POINT ( 'NONE',  ( -9.757819552369539906E-16, -9.499999999869134015, 4.869076758059749821 ) ) ;
#10589=CARTESIAN_POINT ( 'NONE',  ( 135.0000000000000284, -9.047800747817843714, 7.999999999999092282 ) ) ;
#10590=ORIENTED_EDGE ( 'NONE', *, *, #24396, .T. ) ;
#10598=CARTESIAN_POINT ( 'NONE',  ( 135.5000000000000000, -9.047800747817552391, 8.000000000000007105 ) ) ;
#10601=ORIENTED_EDGE ( 'NONE', *, *, #7803, .T. ) ;
#10602=CARTESIAN_POINT ( 'NONE',  ( 154.8750000000000284, 0.000000000000000000, 6.000000000000005329 ) ) ;
#10615=CARTESIAN_POINT ( 'NONE',  ( 159.8052981416689704, -11.45305019762678356, -3.625266920314750951 ) ) ;
#10617=CARTESIAN_POINT ( 'NONE',  ( 0.7566315082547844240, -15.57044312447410483, -7.988287420809495387 ) ) ;
#10620=AXIS2_PLACEMENT_3D ( 'NONE', #21096, #18799, #28126 ) ;
#10625=FACE_OUTER_BOUND ( 'NONE', #19647, .T. ) ;
#10628=ADVANCED_FACE ( 'NONE', ( #28129 ), #1660, .F. ) ;
#10631=ORIENTED_EDGE ( 'NONE', *, *, #4807, .F. ) ;
#10634=DIRECTION ( 'NONE',  ( 0.000000000000000000, -1.000000000000000000, 0.000000000000000000 ) ) ;
#10635=CARTESIAN_POINT ( 'NONE',  ( 153.0863248654052313, 0.000000000000000000, 5.500000000000005329 ) ) ;
#10636=EDGE_LOOP ( 'NONE', ( #12316, #7406, #4553, #11601 ) ) ;
#10640=CARTESIAN_POINT ( 'NONE',  ( 135.0000000000001421, 4.599834066449496994, -3.434280637378118950 ) ) ;
#10645=CARTESIAN_POINT ( 'NONE',  ( 140.6250000000000284, 0.000000000000000000, -6.000000000000005329 ) ) ;
#10647=CARTESIAN_POINT ( 'NONE',  ( 159.8733676508969666, -11.15074878458750085, 4.434313772618972749 ) ) ;
#10649=EDGE_CURVE ( 'NONE', #234, #4156, #26650, .T. ) ;
#10655=CARTESIAN_POINT ( 'NONE',  ( -19.49999999999998224, -54.99999999999990763, -8.000000000000007105 ) ) ;
#10656=CARTESIAN_POINT ( 'NONE',  ( 150.8288997308104058, 4.999999999999989342, -2.071067811865468400 ) ) ;
#10661=FILL_AREA_STYLE_COLOUR ( '', #3463 ) ;
#10664=( BOUNDED_CURVE ( )  B_SPLINE_CURVE ( 2, ( #16446, #30221, #9186, #23021, #1967, #9500, #2427, #4260, #16299 ),
 .UNSPECIFIED., .F., .T. ) 
 B_SPLINE_CURVE_WITH_KNOTS ( ( 3, 2, 2, 2, 3 ),
 ( 0.8375000000000002442, 0.8437500000000000000, 0.8499999999999997558, 0.8562499999999995115, 0.8624999999999993783 ),
 .UNSPECIFIED. ) 
 CURVE ( )  GEOMETRIC_REPRESENTATION_ITEM ( )  RATIONAL_B_SPLINE_CURVE ( ( 0.9999999999999973355, 0.9238795325112894030, 1.000000000000000000, 0.9238795325112867385, 1.000000000000000000, 0.9238795325112867385, 1.000000000000000000, 0.9238795325112948431, 0.9999999999999918954 ) ) 
 REPRESENTATION_ITEM ( '' )  );
#10676=CARTESIAN_POINT ( 'NONE',  ( 144.5625000000000284, -4.242640687119298093, 4.242640687119298093 ) ) ;
#10677=CARTESIAN_POINT ( 'NONE',  ( 142.0386751345948255, -5.500000000000005329, 0.000000000000000000 ) ) ;
#10679=AXIS2_PLACEMENT_3D ( 'NONE', #5699, #3391, #12817 ) ;
#10680=FILL_AREA_STYLE ('',( #8338 ) ) ;
#10681=AXIS2_PLACEMENT_3D ( 'NONE', #9460, #7436, #9150 ) ;
#10683=CIRCLE ( 'NONE', #5243, 1.000000000000000888 ) ;
#10685=CARTESIAN_POINT ( 'NONE',  ( 142.8750000000000284, 0.000000000000000000, 6.000000000000005329 ) ) ;
#10687=ORIENTED_EDGE ( 'NONE', *, *, #11941, .T. ) ;
#10696=ORIENTED_EDGE ( 'NONE', *, *, #15120, .T. ) ;
#10699=CARTESIAN_POINT ( 'NONE',  ( 148.5863248654052313, 0.000000000000000000, 5.500000000000005329 ) ) ;
#10702=COLOUR_RGB ( '', 0.09019608, 0.27058824, 0.51372549) ;
#10713=CARTESIAN_POINT ( 'NONE',  ( 151.5148502691896510, -3.535533905932725318, -3.535533905932725318 ) ) ;
#10714=CARTESIAN_POINT ( 'NONE',  ( 150.3824251345948539, 5.500000000000012434, 2.278174593052012309 ) ) ;
#10715=FACE_OUTER_BOUND ( 'NONE', #22688, .T. ) ;
#10718=CARTESIAN_POINT ( 'NONE',  ( 144.4613248654052313, -5.500000000000005329, 0.000000000000000000 ) ) ;
#10724=CARTESIAN_POINT ( 'NONE',  ( 160.6875000000000284, 4.242640687119269671, 4.242640687119298093 ) ) ;
#10728=ORIENTED_EDGE ( 'NONE', *, *, #24516, .T. ) ;
#10742=CARTESIAN_POINT ( 'NONE',  ( 125.0000000000000568, -55.00000000000000711, 7.500000000000007105 ) ) ;
#10752=FILL_AREA_STYLE_COLOUR ( '', #29999 ) ;
#10753=FILL_AREA_STYLE ('',( #3634 ) ) ;
#10754=CARTESIAN_POINT ( 'NONE',  ( 135.0000000000000284, -8.128268291558169878, 7.787242644550133264 ) ) ;
#10755=ORIENTED_EDGE ( 'NONE', *, *, #1090, .T. ) ;
#10764=CARTESIAN_POINT ( 'NONE',  ( 149.9925748654051745, 2.278174593051981223, 5.500000000000041744 ) ) ;
#10766=( BOUNDED_CURVE ( )  B_SPLINE_CURVE ( 3, ( #6251, #12123, #12270, #16729 ),
 .UNSPECIFIED., .F., .T. ) 
 B_SPLINE_CURVE_WITH_KNOTS ( ( 4, 4 ),
 ( 3.536383773289563326, 4.712388980384689674 ),
 .UNSPECIFIED. ) 
 CURVE ( )  GEOMETRIC_REPRESENTATION_ITEM ( )  RATIONAL_B_SPLINE_CURVE ( ( 1.000000000000000000, 0.8880335295585641830, 0.8880335295585641830, 1.000000000000000000 ) ) 
 REPRESENTATION_ITEM ( '' )  );
#10768=CARTESIAN_POINT ( 'NONE',  ( 158.4375000000000284, -4.242640687119298093, -4.242640687119298093 ) ) ;
#10772=DIRECTION ( 'NONE',  ( 0.000000000000000000, 1.000000000000000000, 0.000000000000000000 ) ) ;
#10773=CIRCLE ( 'NONE', #3861, 1.000000000000000000 ) ;
#10777=CARTESIAN_POINT ( 'NONE',  ( 160.0244396974608208, -11.17509275094623966, 4.373542244167537341 ) ) ;
#10779=ORIENTED_EDGE ( 'NONE', *, *, #23074, .F. ) ;
#10783=DIRECTION ( 'NONE',  ( 1.000000000000000000, 0.000000000000000000, 0.000000000000000000 ) ) ;
#10784=CARTESIAN_POINT ( 'NONE',  ( 8.673617379884035472E-16, -14.14213562373095634, -8.500000000000007105 ) ) ;
#10788=LINE ( 'NONE', #15562, #12671 ) ;
#10793=DIRECTION ( 'NONE',  ( -1.000000000000000000, 0.000000000000000000, 0.000000000000000000 ) ) ;
#10794=AXIS2_PLACEMENT_3D ( 'NONE', #21565, #21260, #16681 ) ;
#10796=CARTESIAN_POINT ( 'NONE',  ( 159.8363248654052313, 0.000000000000000000, -5.500000000000005329 ) ) ;
#10801=DIRECTION ( 'NONE',  ( -1.387778780781444256E-14, -1.000000000000000000, -0.000000000000000000 ) ) ;
#10802=EDGE_CURVE ( 'NONE', #13611, #11502, #19331, .T. ) ;
#10806=ORIENTED_EDGE ( 'NONE', *, *, #23823, .T. ) ;
#10807=CARTESIAN_POINT ( 'NONE',  ( 138.1011751345948539, 3.889087296526011706, -3.889087296526011706 ) ) ;
#10808=CARTESIAN_POINT ( 'NONE',  ( 144.1875000000000284, 4.242640687119269671, 4.242640687119298093 ) ) ;
#10810=EDGE_CURVE ( 'NONE', #17667, #476, #10011, .T. ) ;
#10813=CARTESIAN_POINT ( 'NONE',  ( 136.2113248654052029, 5.500000000000005329, 0.000000000000000000 ) ) ;
#10815=AXIS2_PLACEMENT_3D ( 'NONE', #20458, #27653, #27499 ) ;
#10819=VECTOR ( 'NONE', #28264, 1000.000000000000000 ) ;
#10820=CARTESIAN_POINT ( 'NONE',  ( 147.9226497308104058, 5.000000000000004441, 0.000000000000000000 ) ) ;
#10822=CARTESIAN_POINT ( 'NONE',  ( 140.5384615384615756, -11.07692307692306777, 4.615384615384604317 ) ) ;
#10825=CARTESIAN_POINT ( 'NONE',  ( -0.5000000000000004441, -9.500000000000008882, -7.500000000000007105 ) ) ;
#10834=CARTESIAN_POINT ( 'NONE',  ( 149.0625000000000284, -4.242640687119298093, 4.242640687119298093 ) ) ;
#10838=( GEOMETRIC_REPRESENTATION_CONTEXT ( 3 ) GLOBAL_UNCERTAINTY_ASSIGNED_CONTEXT ( ( #12163 ) ) GLOBAL_UNIT_ASSIGNED_CONTEXT ( ( #769, #24715, #17377 ) ) REPRESENTATION_CONTEXT ( 'NONE', 'WORKASPACE' ) );
#10841=CARTESIAN_POINT ( 'NONE',  ( 140.4375000000000284, -4.242640687119298093, -4.242640687119298093 ) ) ;
#10842=CARTESIAN_POINT ( 'NONE',  ( 161.2636380912115612, -5.033346391500745476, 2.825791916966355011 ) ) ;
#10853=DIRECTION ( 'NONE',  ( 0.000000000000000000, 0.000000000000000000, -1.000000000000000000 ) ) ;
#10854=VECTOR ( 'NONE', #13096, 1000.000000000000000 ) ;
#10861=CARTESIAN_POINT ( 'NONE',  ( 156.6488248654052029, -3.889087296526011706, -3.889087296526011706 ) ) ;
#10864=SURFACE_STYLE_USAGE ( .BOTH. , #19604 ) ;
#10868=CARTESIAN_POINT ( 'NONE',  ( 151.7886751345948255, 5.500000000000005329, 0.000000000000000000 ) ) ;
#10869=CARTESIAN_POINT ( 'NONE',  ( 139.5863248654052313, 0.000000000000000000, 5.500000000000005329 ) ) ;
#10870=ADVANCED_FACE ( 'NONE', ( #3527 ), #29027, .F. ) ;
#10871=CARTESIAN_POINT ( 'NONE',  ( 150.1800748654052029, -2.278174593052043395, 5.499999999999981348 ) ) ;
#10874=VERTEX_POINT ( 'NONE', #5677 ) ;
#10875=CARTESIAN_POINT ( 'NONE',  ( 161.6250000000000568, 0.000000000000000000, -6.000000000000005329 ) ) ;
#10876=DIRECTION ( 'NONE',  ( 0.000000000000000000, 0.000000000000000000, 1.000000000000000000 ) ) ;
#10884=LINE ( 'NONE', #22840, #19043 ) ;
#10891=VERTEX_POINT ( 'NONE', #10796 ) ;
#10893=( NAMED_UNIT ( * ) PLANE_ANGLE_UNIT ( ) SI_UNIT ( $, .RADIAN. ) );
#10894=CARTESIAN_POINT ( 'NONE',  ( 1.000000000000000666, -16.31586670994437682, -6.338163299696071284 ) ) ;
#10897=( NAMED_UNIT ( * ) SI_UNIT ( $, .STERADIAN. ) SOLID_ANGLE_UNIT ( ) );
#10898=AXIS2_PLACEMENT_3D ( 'NONE', #3971, #3665, #6434 ) ;
#10900=DIRECTION ( 'NONE',  ( 0.000000000000000000, 0.000000000000000000, -1.000000000000000000 ) ) ;
#10902=DIRECTION ( 'NONE',  ( 1.000000000000000000, 0.000000000000000000, -0.000000000000000000 ) ) ;
#10904=CARTESIAN_POINT ( 'NONE',  ( 135.4999999999991189, -9.047800747817843714, 8.000000000000007105 ) ) ;
#10905=ORIENTED_EDGE ( 'NONE', *, *, #1432, .F. ) ;
#10909=ADVANCED_FACE ( 'NONE', ( #3372 ), #6155, .F. ) ;
#10915=CARTESIAN_POINT ( 'NONE',  ( 135.0000000000000284, 1.469576158976823947E-15, 12.00000000000000178 ) ) ;
#10916=ORIENTED_EDGE ( 'NONE', *, *, #11013, .F. ) ;
#10918=COLOUR_RGB ( '', 0.66274510, 0.83137255, 0.94901961) ;
#10920=ORIENTED_EDGE ( 'NONE', *, *, #332, .F. ) ;
#10921=CARTESIAN_POINT ( 'NONE',  ( 157.7812500000000568, 2.485281374238585972, 6.000000000000005329 ) ) ;
#10922=VECTOR ( 'NONE', #12198, 1000.000000000000000 ) ;
#10929=FACE_OUTER_BOUND ( 'NONE', #8427, .T. ) ;
#10933=CARTESIAN_POINT ( 'NONE',  ( 159.5092728369245378, -12.11071345234885754, -3.863094837972295803 ) ) ;
#10934=CYLINDRICAL_SURFACE ( 'NONE', #13859, 15.00000000000000000 ) ;
#10947=CARTESIAN_POINT ( 'NONE',  ( 138.9523502691896510, 0.000000000000000000, 5.000000000000004441 ) ) ;
#10951=ORIENTED_EDGE ( 'NONE', *, *, #3720, .F. ) ;
#10961=CARTESIAN_POINT ( 'NONE',  ( 140.7187500000000284, 2.485281374238555774, -6.000000000000005329 ) ) ;
#10964=LINE ( 'NONE', #18335, #13137 ) ;
#10967=CARTESIAN_POINT ( 'NONE',  ( 116.0000000000000142, 0.000000000000000000, 0.000000000000000000 ) ) ;
#10968=DIRECTION ( 'NONE',  ( -0.000000000000000000, -0.000000000000000000, -1.000000000000000000 ) ) ;
#10970=VECTOR ( 'NONE', #16206, 1000.000000000000000 ) ;
#10971=CARTESIAN_POINT ( 'NONE',  ( 150.4538997308104626, -2.071067811865468400, -4.999999999999989342 ) ) ;
#10973=FACE_OUTER_BOUND ( 'NONE', #26184, .T. ) ;
#10976=FACE_OUTER_BOUND ( 'NONE', #22723, .T. ) ;
#10977=CARTESIAN_POINT ( 'NONE',  ( 135.0476735965559101, -7.696154670787128005, 8.313613484422726074 ) ) ;
#10987=CARTESIAN_POINT ( 'NONE',  ( 145.5937500000000284, 6.000000000000005329, 2.485281374238585972 ) ) ;
#10988=CARTESIAN_POINT ( 'NONE',  ( 161.0000000000000284, -11.67610212985246676, -2.769230769230771827 ) ) ;
#10989=LINE ( 'NONE', #8659, #13630 ) ;
#10991=CARTESIAN_POINT ( 'NONE',  ( 135.5625000000000284, -4.242640687119298093, 4.242640687119298093 ) ) ;
#10993=ORIENTED_EDGE ( 'NONE', *, *, #25616, .T. ) ;
#10994=( BOUNDED_CURVE ( )  B_SPLINE_CURVE ( 2, ( #10352, #29058, #7870, #3107, #14671, #5110, #12238, #12381, #14963 ),
 .UNSPECIFIED., .F., .F. ) 
 B_SPLINE_CURVE_WITH_KNOTS ( ( 3, 2, 2, 2, 3 ),
 ( 0.4875000000000000444, 0.4937500000000002998, 0.5000000000000005551, 0.5062500000000007550, 0.5125000000000009548 ),
 .UNSPECIFIED. ) 
 CURVE ( )  GEOMETRIC_REPRESENTATION_ITEM ( )  RATIONAL_B_SPLINE_CURVE ( ( 0.9999999999999993339, 0.9238795325112874046, 1.000000000000000000, 0.9238795325112867385, 1.000000000000000000, 0.9238795325112867385, 1.000000000000000000, 0.9238795325112745260, 1.000000000000012212 ) ) 
 REPRESENTATION_ITEM ( '' )  );
#10998=VERTEX_POINT ( 'NONE', #1386 ) ;
#11005=CARTESIAN_POINT ( 'NONE',  ( 148.3050748654052029, 5.500000000000012434, 2.278174593052012309 ) ) ;
#11006=DIRECTION ( 'NONE',  ( -0.000000000000000000, -0.000000000000000000, -1.000000000000000000 ) ) ;
#11013=EDGE_CURVE ( 'NONE', #16005, #9495, #10368, .T. ) ;
#11018=CARTESIAN_POINT ( 'NONE',  ( 135.2886751345948539, 5.500000000000005329, 0.000000000000000000 ) ) ;
#11023=CARTESIAN_POINT ( 'NONE',  ( 158.7187500000000000, 2.485281374238555774, -6.000000000000005329 ) ) ;
#11027=EDGE_LOOP ( 'NONE', ( #3732, #10993, #897, #11690 ) ) ;
#11032=CARTESIAN_POINT ( 'NONE',  ( -0.5000000000000004441, -14.50000000000001243, -8.000000000000007105 ) ) ;
#11038=DIRECTION ( 'NONE',  ( 0.000000000000000000, 0.000000000000000000, 1.000000000000000000 ) ) ;
#11048=FACE_OUTER_BOUND ( 'NONE', #19289, .T. ) ;
#11049=DIRECTION ( 'NONE',  ( -1.000000000000000000, 0.000000000000000000, 0.000000000000000000 ) ) ;
#11062=ORIENTED_EDGE ( 'NONE', *, *, #28305, .T. ) ;
#11063=CARTESIAN_POINT ( 'NONE',  ( 159.4687500000000568, -2.485281374238585972, 6.000000000000005329 ) ) ;
#11064=AXIS2_PLACEMENT_3D ( 'NONE', #27745, #18424, #2126 ) ;
#11071=FACE_OUTER_BOUND ( 'NONE', #21527, .T. ) ;
#11076=ORIENTED_EDGE ( 'NONE', *, *, #17627, .F. ) ;
#11080=CARTESIAN_POINT ( 'NONE',  ( 159.1714057324313103, -11.33333333361816031, -3.999999999173795562 ) ) ;
#11085=DIRECTION ( 'NONE',  ( 1.000000000000000000, 0.000000000000000000, -0.000000000000000000 ) ) ;
#11087=DIRECTION ( 'NONE',  ( -0.000000000000000000, -0.000000000000000000, -1.000000000000000000 ) ) ;
#11088=CARTESIAN_POINT ( 'NONE',  ( -39.00000000000000000, -20.00000000000001776, 3.000000000000002665 ) ) ;
#11090=( NAMED_UNIT ( * ) PLANE_ANGLE_UNIT ( ) SI_UNIT ( $, .RADIAN. ) );
#11093=AXIS2_PLACEMENT_3D ( 'NONE', #2970, #28764, #12098 ) ;
#11095=CARTESIAN_POINT ( 'NONE',  ( 141.2961002691896510, 2.071067811865468400, -4.999999999999989342 ) ) ;
#11102=AXIS2_PLACEMENT_3D ( 'NONE', #8717, #25125, #20385 ) ;
#11105=CARTESIAN_POINT ( 'NONE',  ( 144.2812500000000284, 2.485281374238585972, 6.000000000000005329 ) ) ;
#11107=ORIENTED_EDGE ( 'NONE', *, *, #5413, .T. ) ;
#11108=( NAMED_UNIT ( * ) PLANE_ANGLE_UNIT ( ) SI_UNIT ( $, .RADIAN. ) );
#11112=FACE_OUTER_BOUND ( 'NONE', #755, .T. ) ;
#11115=CARTESIAN_POINT ( 'NONE',  ( 151.5788997308104058, -4.999999999999989342, 2.071067811865468400 ) ) ;
#11118=CARTESIAN_POINT ( 'NONE',  ( -1.000000000000000888, 9.000000000000007105, -3.000000000000002665 ) ) ;
#11119=CARTESIAN_POINT ( 'NONE',  ( -0.5000000000000004441, -15.00000000000001421, -8.000000000000007105 ) ) ;
#11122=CARTESIAN_POINT ( 'NONE',  ( 137.7261751345948539, -3.889087296526011706, -3.889087296526011706 ) ) ;
#11130=CARTESIAN_POINT ( 'NONE',  ( 148.5937500000000284, 6.000000000000005329, 2.485281374238585972 ) ) ;
#11133=DIRECTION ( 'NONE',  ( -0.3589790793088787901, 0.3589790793088650789, -0.8615497903412834280 ) ) ;
#11135=VECTOR ( 'NONE', #20937, 1000.000000000000000 ) ;
#11136=ORIENTED_EDGE ( 'NONE', *, *, #10051, .F. ) ;
#11137=ADVANCED_FACE ( 'NONE', ( #13566 ), #22904, .F. ) ;
#11138=COLOUR_RGB ( '', 0.40784314, 0.44705882, 0.49803922) ;
#11143=AXIS2_PLACEMENT_3D ( 'NONE', #3706, #4329, #13747 ) ;
#11147=EDGE_CURVE ( 'NONE', #13151, #13576, #4503, .T. ) ;
#11151=DIRECTION ( 'NONE',  ( 0.000000000000000000, 0.000000000000000000, 1.000000000000000000 ) ) ;
#11155=CARTESIAN_POINT ( 'NONE',  ( 0.000000000000000000, -14.26438599474648683, -8.432200732276358579 ) ) ;
#11156=AXIS2_PLACEMENT_3D ( 'NONE', #18671, #20656, #27991 ) ;
#11161=DIRECTION ( 'NONE',  ( -1.000000000000000000, 1.040834085586083310E-14, 0.000000000000000000 ) ) ;
#11163=CARTESIAN_POINT ( 'NONE',  ( 149.3586002691896510, 2.071067811865468400, 4.999999999999989342 ) ) ;
#11166=( GEOMETRIC_REPRESENTATION_CONTEXT ( 3 ) GLOBAL_UNCERTAINTY_ASSIGNED_CONTEXT ( ( #28367 ) ) GLOBAL_UNIT_ASSIGNED_CONTEXT ( ( #26791, #24660, #15168 ) ) REPRESENTATION_CONTEXT ( 'NONE', 'WORKASPACE' ) );
#11167=CARTESIAN_POINT ( 'NONE',  ( 135.0000000000066223, -7.337284433953279894, -8.409043885017243980 ) ) ;
#11170=CARTESIAN_POINT ( 'NONE',  ( 139.2261751345948539, -3.889087296526011706, -3.889087296526011706 ) ) ;
#11174=VERTEX_POINT ( 'NONE', #2005 ) ;
#11175=CARTESIAN_POINT ( 'NONE',  ( 157.5000000000000284, 6.000000000000005329, 0.000000000000000000 ) ) ;
#11180=VERTEX_POINT ( 'NONE', #9535 ) ;
#11181=ORIENTED_EDGE ( 'NONE', *, *, #6922, .T. ) ;
#11182=ORIENTED_EDGE ( 'NONE', *, *, #11786, .T. ) ;
#11188=EDGE_CURVE ( 'NONE', #7302, #15059, #5090, .T. ) ;
#11189=CARTESIAN_POINT ( 'NONE',  ( 116.0000000000000142, 0.000000000000000000, 0.000000000000000000 ) ) ;
#11199=CARTESIAN_POINT ( 'NONE',  ( -0.04562205425674009662, -14.50000000000001243, 8.291335958003937634 ) ) ;
#11202=CARTESIAN_POINT ( 'NONE',  ( 145.6800748654052029, -2.278174593052012309, 5.500000000000012434 ) ) ;
#11204=CARTESIAN_POINT ( 'NONE',  ( 159.4836002691896226, 4.999999999999989342, -2.071067811865468400 ) ) ;
#11205=DIRECTION ( 'NONE',  ( 0.000000000000000000, -1.000000000000000000, 0.000000000000000000 ) ) ;
#11206=CARTESIAN_POINT ( 'NONE',  ( -0.07773347327279958585, -14.92041145833903393, 8.102883078117887550 ) ) ;
#11218=DIRECTION ( 'NONE',  ( -0.000000000000000000, -0.000000000000000000, -1.000000000000000000 ) ) ;
#11219=( BOUNDED_SURFACE ( )  B_SPLINE_SURFACE ( 3, 2, ( 
 ( #29355, #8317, #24762 ),
 ( #22471, #1409, #20931 ),
 ( #25201, #11588, #4164 ),
 ( #25512, #20462, #22774 ),
 ( #23088, #15903, #11272 ),
 ( #22929, #4476, #20625 ),
 ( #2030, #11436, #18635 ),
 ( #6931, #8949, #20318 ) ),
 .UNSPECIFIED., .F., .F., .T. ) 
 B_SPLINE_SURFACE_WITH_KNOTS ( ( 4, 2, 2, 4 ),
 ( 3, 3 ),
 ( 0.006483209092139470726, 0.007220185479632802716, 0.007957161867126135574, 0.009431114642112801288 ),
 ( 0.000000000000000000, 1.000000000000000000 ),
 .UNSPECIFIED. ) 
 GEOMETRIC_REPRESENTATION_ITEM ( )  RATIONAL_B_SPLINE_SURFACE ( (
 ( 1.000000000000000000, 0.9165151389911680990, 1.000000000000000000),
 ( 1.000000000000000000, 0.9165811099392860983, 1.000000000000000000),
 ( 1.000000000000000000, 0.9096513889649350260, 1.000000000000000000),
 ( 1.000000000000000000, 0.8858533194321830395, 1.000000000000000000),
 ( 1.000000000000000000, 0.8692663461313614448, 1.000000000000000000),
 ( 1.000000000000000000, 0.8111162787353217718, 1.000000000000000000),
 ( 1.000000000000000000, 0.7613968795859874517, 1.000000000000000000),
 ( 1.000000000000000000, 0.7050799574960493477, 1.000000000000000000) ) ) 
 REPRESENTATION_ITEM ( '' )  SURFACE ( )  );
#11221=CARTESIAN_POINT ( 'NONE',  ( 156.2812500000000284, 2.485281374238585972, 6.000000000000005329 ) ) ;
#11225=ORIENTED_EDGE ( 'NONE', *, *, #23724, .F. ) ;
#11229=( NAMED_UNIT ( * ) SI_UNIT ( $, .STERADIAN. ) SOLID_ANGLE_UNIT ( ) );
#11230=DIRECTION ( 'NONE',  ( 1.000000000000000000, -0.000000000000000000, -0.000000000000000000 ) ) ;
#11231=ORIENTED_EDGE ( 'NONE', *, *, #14028, .T. ) ;
#11233=CARTESIAN_POINT ( 'NONE',  ( -0.07940172813350243608, -15.22961641030811286, -7.558960887114970717 ) ) ;
#11236=DIRECTION ( 'NONE',  ( 1.000000000000000000, 0.000000000000000000, 0.000000000000000000 ) ) ;
#11237=LINE ( 'NONE', #1988, #26614 ) ;
#11243=CYLINDRICAL_SURFACE ( 'NONE', #15291, 5.500000000000000000 ) ;
#11246=CARTESIAN_POINT ( 'NONE',  ( 154.5863248654052313, 0.000000000000000000, 5.500000000000005329 ) ) ;
#11247=VERTEX_POINT ( 'NONE', #12172 ) ;
#11249=CARTESIAN_POINT ( 'NONE',  ( 135.0000000000000000, 1.949781249179272091, -5.142796231657337458 ) ) ;
#11251=CARTESIAN_POINT ( 'NONE',  ( 139.4211002691896795, -4.999999999999989342, -2.071067811865468400 ) ) ;
#11258=CARTESIAN_POINT ( 'NONE',  ( 140.5000000000000284, -10.99818166789400919, -4.800000000000004263 ) ) ;
#11261=ORIENTED_EDGE ( 'NONE', *, *, #5654, .T. ) ;
#11264=CARTESIAN_POINT ( 'NONE',  ( 142.3125000000000284, 4.242640687119298093, -4.242640687119298093 ) ) ;
#11272=CARTESIAN_POINT ( 'NONE',  ( 134.9486760519935444, -8.594915014407842335, -8.000000000000007105 ) ) ;
#11273=CARTESIAN_POINT ( 'NONE',  ( 142.6726497308104342, -5.000000000000004441, 0.000000000000000000 ) ) ;
#11281=STYLED_ITEM ( 'NONE', ( #20929 ), #25858 ) ;
#11289=DIRECTION ( 'NONE',  ( -0.000000000000000000, -0.000000000000000000, -1.000000000000000000 ) ) ;
#11292=CARTESIAN_POINT ( 'NONE',  ( 146.7187500000000284, 2.485281374238556218, -6.000000000000005329 ) ) ;
#11293=CARTESIAN_POINT ( 'NONE',  ( 159.8704966968991243, -12.37217944490604360, -3.496373867771979782 ) ) ;
#11295=CARTESIAN_POINT ( 'NONE',  ( 140.5384615384615756, -11.53846153846155254, -4.807692307692318145 ) ) ;
#11296=EDGE_CURVE ( 'NONE', #2328, #17215, #27395, .T. ) ;
#11297=CARTESIAN_POINT ( 'NONE',  ( 136.6875000000000284, 4.242640687119269671, 4.242640687119298093 ) ) ;
#11299=VECTOR ( 'NONE', #20500, 1000.000000000000000 ) ;
#11301=CIRCLE ( 'NONE', #6857, 1.000000000000000000 ) ;
#11306=B_SPLINE_CURVE_WITH_KNOTS ( 'NONE', 3,
 ( #25703, #14522, #12075, #9587, #26003, #49, #2950, #24004, #21413, #346 ),
 .UNSPECIFIED., .F., .F.,
 ( 4, 2, 2, 2, 4 ),
 ( 0.000000000000000000, 0.0004268114089743834153, 0.0008536228179487668306, 0.001280434226923150192, 0.001707245635897533228 ),
 .UNSPECIFIED. ) ;
#11312=DIRECTION ( 'NONE',  ( 1.000000000000000000, 6.938893903907222067E-15, 0.000000000000000000 ) ) ;
#11320=CARTESIAN_POINT ( 'NONE',  ( -0.5043617743979548207, -9.495638225601934934, 4.110987936241946805 ) ) ;
#11326=CARTESIAN_POINT ( 'NONE',  ( 147.9523502691896510, 0.000000000000000000, 5.000000000000004441 ) ) ;
#11329=CARTESIAN_POINT ( 'NONE',  ( 144.1800748654052597, -2.278174593051981223, 5.500000000000041744 ) ) ;
#11331=AXIS2_PLACEMENT_3D ( 'NONE', #15079, #12951, #19974 ) ;
#11336=ORIENTED_EDGE ( 'NONE', *, *, #20032, .F. ) ;
#11337=CARTESIAN_POINT ( 'NONE',  ( 153.3750000000000284, 0.000000000000000000, 6.000000000000005329 ) ) ;
#11342=VERTEX_POINT ( 'NONE', #18232 ) ;
#11348=CARTESIAN_POINT ( 'NONE',  ( 140.5000000000000284, -9.510965941585999062, -7.318712077885313860 ) ) ;
#11349=CARTESIAN_POINT ( 'NONE',  ( 0.7660981036491463225, -15.49911073742189416, 8.125819281016111617 ) ) ;
#11354=B_SPLINE_CURVE_WITH_KNOTS ( 'NONE', 3,
 ( #24796, #22200, #15630, #15470, #17458, #29704, #27388, #1602, #22045, #13177, #983, #8513 ),
 .UNSPECIFIED., .F., .F.,
 ( 4, 2, 2, 2, 2, 4 ),
 ( 0.000000000000000000, 0.0002876650772533674311, 0.0005753301545067348623, 0.001150660309013472760, 0.001725990463520215212, 0.002301320618026957664 ),
 .UNSPECIFIED. ) ;
#11356=CARTESIAN_POINT ( 'NONE',  ( 139.5000000000000000, -8.798545334315205579, 8.160000000000000142 ) ) ;
#11363=CARTESIAN_POINT ( 'NONE',  ( 146.0550748654052313, -5.500000000000012434, -2.278174593052012309 ) ) ;
#11365=( NAMED_UNIT ( * ) PLANE_ANGLE_UNIT ( ) SI_UNIT ( $, .RADIAN. ) );
#11366=CARTESIAN_POINT ( 'NONE',  ( 0.7618037995490587466, -15.57909779039840181, 7.971327808482444155 ) ) ;
#11370=VECTOR ( 'NONE', #28776, 1000.000000000000000 ) ;
#11372=EDGE_CURVE ( 'NONE', #27983, #25655, #13334, .T. ) ;
#11374=AXIS2_PLACEMENT_3D ( 'NONE', #1958, #20708, #8724 ) ;
#11375=VERTEX_POINT ( 'NONE', #8692 ) ;
#11378=CIRCLE ( 'NONE', #9394, 1.000000000000000000 ) ;
#11382=CARTESIAN_POINT ( 'NONE',  ( 149.9062500000000568, 6.000000000000005329, -2.485281374238555774 ) ) ;
#11391=FACE_OUTER_BOUND ( 'NONE', #11027, .T. ) ;
#11399=VECTOR ( 'NONE', #24087, 1000.000000000000000 ) ;
#11402=CARTESIAN_POINT ( 'NONE',  ( -9.757819552369539906E-16, -9.500000000000008882, -5.000000000000004441 ) ) ;
#11403=ADVANCED_FACE ( 'NONE', ( #15333 ), #17786, .T. ) ;
#11405=DIRECTION ( 'NONE',  ( 0.000000000000000000, 0.000000000000000000, 1.000000000000000000 ) ) ;
#11409=AXIS2_PLACEMENT_3D ( 'NONE', #18318, #27631, #23064 ) ;
#11412=AXIS2_PLACEMENT_3D ( 'NONE', #28902, #20176, #18311 ) ;
#11415=CARTESIAN_POINT ( 'NONE',  ( 136.1398502691896510, -3.535533905932752852, 3.535533905932725318 ) ) ;
#11417=CIRCLE ( 'NONE', #26082, 12.50000000000000178 ) ;
#11419=CARTESIAN_POINT ( 'NONE',  ( 141.0000000000000284, -54.99999999999989342, 4.000000000000003553 ) ) ;
#11427=CARTESIAN_POINT ( 'NONE',  ( 139.0312500000000853, -2.485281374238555774, -6.000000000000005329 ) ) ;
#11429=ORIENTED_EDGE ( 'NONE', *, *, #21685, .T. ) ;
#11436=CARTESIAN_POINT ( 'NONE',  ( 134.9273262448178627, -7.354674723950151538, -8.000000000000007105 ) ) ;
#11437=CARTESIAN_POINT ( 'NONE',  ( 142.1101497308104058, 3.535533905932725318, 3.535533905932725318 ) ) ;
#11438=CYLINDRICAL_SURFACE ( 'NONE', #12396, 12.00000000000000178 ) ;
#11441=FACE_OUTER_BOUND ( 'NONE', #24147, .T. ) ;
#11446=EDGE_CURVE ( 'NONE', #9337, #13233, #21159, .T. ) ;
#11450=CYLINDRICAL_SURFACE ( 'NONE', #23853, 5.500000000000000000 ) ;
#11451=EDGE_LOOP ( 'NONE', ( #29384, #23643, #5502, #10491 ) ) ;
#11454=DIRECTION ( 'NONE',  ( 0.000000000000000000, 1.000000000000000000, -0.000000000000000000 ) ) ;
#11455=LINE ( 'NONE', #25842, #13128 ) ;
#11456=ORIENTED_EDGE ( 'NONE', *, *, #4870, .F. ) ;
#11458=CARTESIAN_POINT ( 'NONE',  ( 139.0312500000000568, -2.485281374238556218, -6.000000000000005329 ) ) ;
#11459=CARTESIAN_POINT ( 'NONE',  ( 160.0398553692754149, -11.61772494185188265, -3.016142447635661306 ) ) ;
#11461=CARTESIAN_POINT ( 'NONE',  ( 138.0000000000000284, 6.000000000000005329, 0.000000000000000000 ) ) ;
#11462=DIRECTION ( 'NONE',  ( 0.000000000000000000, 0.000000000000000000, 1.000000000000000000 ) ) ;
#11463=EDGE_LOOP ( 'NONE', ( #22020, #29832, #5800, #29454, #24920, #13597, #2287, #27151, #8422, #21400, #26362, #28471, #16967, #23270, #8499, #15459, #11062 ) ) ;
#11467=ORIENTED_EDGE ( 'NONE', *, *, #24839, .F. ) ;
#11472=DIRECTION ( 'NONE',  ( 0.000000000000000000, 0.000000000000000000, -1.000000000000000000 ) ) ;
#11474=ADVANCED_FACE ( 'NONE', ( #2527 ), #11901, .T. ) ;
#11487=CARTESIAN_POINT ( 'NONE',  ( 147.2023502691896510, 0.000000000000000000, -5.000000000000004441 ) ) ;
#11488=LINE ( 'NONE', #8996, #13769 ) ;
#11490=CARTESIAN_POINT ( 'NONE',  ( 156.9375000000000284, -4.242640687119298093, -4.242640687119298093 ) ) ;
#11491=CARTESIAN_POINT ( 'NONE',  ( 13.99999999999999822, 0.000000000000000000, 0.000000000000000000 ) ) ;
#11497=CARTESIAN_POINT ( 'NONE',  ( 156.6562500000000284, -6.000000000000005329, 2.485281374238555774 ) ) ;
#11498=CARTESIAN_POINT ( 'NONE',  ( -4.999999999999984013, -69.50000000000001421, 7.500000000000007105 ) ) ;
#11500=FACE_OUTER_BOUND ( 'NONE', #16293, .T. ) ;
#11502=VERTEX_POINT ( 'NONE', #11954 ) ;
#11504=ORIENTED_EDGE ( 'NONE', *, *, #24710, .T. ) ;
#11515=DIRECTION ( 'NONE',  ( 0.000000000000000000, 0.000000000000000000, -1.000000000000000000 ) ) ;
#11522=CARTESIAN_POINT ( 'NONE',  ( 161.4523502691896510, 0.000000000000000000, 5.000000000000004441 ) ) ;
#11535=CARTESIAN_POINT ( 'NONE',  ( 152.3437500000000568, -6.000000000000005329, -2.485281374238555774 ) ) ;
#11537=EDGE_CURVE ( 'NONE', #9814, #23810, #4030, .T. ) ;
#11542=DIRECTION ( 'NONE',  ( 0.000000000000000000, 1.000000000000000000, -0.000000000000000000 ) ) ;
#11545=CARTESIAN_POINT ( 'NONE',  ( 160.0396984632319572, -11.61764268043064696, 3.016434873857221088 ) ) ;
#11550=DIRECTION ( 'NONE',  ( -0.000000000000000000, -0.000000000000000000, -1.000000000000000000 ) ) ;
#11552=CARTESIAN_POINT ( 'NONE',  ( 153.1949251345948539, 5.500000000000012434, -2.278174593052012309 ) ) ;
#11553=FACE_OUTER_BOUND ( 'NONE', #26924, .T. ) ;
#11558=CARTESIAN_POINT ( 'NONE',  ( -0.8691260360719468281, -9.261747927856070817, -4.026027341348647148 ) ) ;
#11560=VECTOR ( 'NONE', #17514, 1000.000000000000000 ) ;
#11561=CARTESIAN_POINT ( 'NONE',  ( 159.8739699821186093, -11.15087202985791848, -4.434002056370806244 ) ) ;
#11563=CARTESIAN_POINT ( 'NONE',  ( 135.0000000000000284, -8.301012159643168076, -7.690749534758824169 ) ) ;
#11565=ORIENTED_EDGE ( 'NONE', *, *, #28923, .F. ) ;
#11567=VERTEX_POINT ( 'NONE', #7577 ) ;
#11575=CARTESIAN_POINT ( 'NONE',  ( 1.000000000000000888, 0.000000000000000000, -16.50000000000000355 ) ) ;
#11576=CARTESIAN_POINT ( 'NONE',  ( 138.9375000000000568, -4.242640687119298093, -4.242640687119298093 ) ) ;
#11584=EDGE_CURVE ( 'NONE', #14826, #27080, #4006, .T. ) ;
#11588=CARTESIAN_POINT ( 'NONE',  ( 135.6059727065479876, -8.864963804572132844, -8.000000000000007105 ) ) ;
#11589=EDGE_CURVE ( 'NONE', #4075, #28330, #4970, .T. ) ;
#11590=CARTESIAN_POINT ( 'NONE',  ( 145.2976497308104058, 0.000000000000000000, 5.000000000000004441 ) ) ;
#11593=CARTESIAN_POINT ( 'NONE',  ( 124.9999999999999432, -69.50000000000000000, 8.000000000000007105 ) ) ;
#11601=ORIENTED_EDGE ( 'NONE', *, *, #28996, .F. ) ;
#11605=CARTESIAN_POINT ( 'NONE',  ( -4.999999999999920952, -65.00000000000001421, 8.000000000000007105 ) ) ;
#11606=AXIS2_PLACEMENT_3D ( 'NONE', #10742, #3782, #27426 ) ;
#11607=ORIENTED_EDGE ( 'NONE', *, *, #8945, .T. ) ;
#11609=CARTESIAN_POINT ( 'NONE',  ( 137.6250000000000284, 0.000000000000000000, -6.000000000000005329 ) ) ;
#11611=DIRECTION ( 'NONE',  ( -0.000000000000000000, -0.000000000000000000, -1.000000000000000000 ) ) ;
#11612=CARTESIAN_POINT ( 'NONE',  ( 160.3913997308104058, -2.071067811865468400, 4.999999999999989342 ) ) ;
#11614=CIRCLE ( 'NONE', #26271, 16.50000000000000355 ) ;
#11615=EDGE_CURVE ( 'NONE', #9180, #3348, #29219, .T. ) ;
#11622=EDGE_CURVE ( 'NONE', #25006, #234, #28466, .T. ) ;
#11624=AXIS2_PLACEMENT_3D ( 'NONE', #20694, #13504, #13973 ) ;
#11627=FACE_OUTER_BOUND ( 'NONE', #26579, .T. ) ;
#11639=CARTESIAN_POINT ( 'NONE',  ( 150.6711002691896226, 4.999999999999989342, 2.071067811865468400 ) ) ;
#11642=CARTESIAN_POINT ( 'NONE',  ( 159.4687500000000568, -2.485281374238585972, 6.000000000000005329 ) ) ;
#11643=PRESENTATION_STYLE_ASSIGNMENT (( #28167 ) ) ;
#11646=CARTESIAN_POINT ( 'NONE',  ( 160.0000000000000284, -59.99999999999980105, 4.000000000000003553 ) ) ;
#11648=SURFACE_STYLE_USAGE ( .BOTH. , #13960 ) ;
#11650=CARTESIAN_POINT ( 'NONE',  ( 154.9687500000000284, -2.485281374238585972, 6.000000000000005329 ) ) ;
#11656=EDGE_LOOP ( 'NONE', ( #18060, #10144, #4912, #3420 ) ) ;
#11662=VERTEX_POINT ( 'NONE', #15610 ) ;
#11663=FACE_OUTER_BOUND ( 'NONE', #20996, .T. ) ;
#11664=CARTESIAN_POINT ( 'NONE',  ( 0.000000000000000000, -10.50000000000000888, 7.500000000000007105 ) ) ;
#11665=AXIS2_PLACEMENT_3D ( 'NONE', #902, #10301, #15548 ) ;
#11667=ORIENTED_EDGE ( 'NONE', *, *, #17666, .T. ) ;
#11669=AXIS2_PLACEMENT_3D ( 'NONE', #29062, #21877, #17433 ) ;
#11675=( BOUNDED_SURFACE ( )  B_SPLINE_SURFACE ( 3, 2, ( 
 ( #19674, #15556, #6142 ),
 ( #12787, #15233, #22131 ),
 ( #29321, #12945, #29161 ),
 ( #10784, #10462, #1209 ) ),
 .UNSPECIFIED., .F., .F., .F. ) 
 B_SPLINE_SURFACE_WITH_KNOTS ( ( 4, 4 ),
 ( 3, 3 ),
 ( 2.710505431213761085E-18, 0.0007339382808609110857 ),
 ( 0.000000000000000000, 1.000000000000000000 ),
 .UNSPECIFIED. ) 
 GEOMETRIC_REPRESENTATION_ITEM ( )  RATIONAL_B_SPLINE_SURFACE ( (
 ( 1.000000000000000000, 0.7743236465966895077, 1.000000000000000000),
 ( 1.000000000000000000, 0.7550843754125133866, 1.000000000000000000),
 ( 1.000000000000000000, 0.7330092777270662552, 1.000000000000000000),
 ( 1.000000000000000000, 0.7071067811865475727, 1.000000000000000000) ) ) 
 REPRESENTATION_ITEM ( '' )  SURFACE ( )  );
#11677=CARTESIAN_POINT ( 'NONE',  ( 0.1257426365907835797, -15.26923055284497366, 8.555419898867683060 ) ) ;
#11686=VECTOR ( 'NONE', #28625, 1000.000000000000000 ) ;
#11690=ORIENTED_EDGE ( 'NONE', *, *, #18893, .F. ) ;
#11692=VERTEX_POINT ( 'NONE', #1112 ) ;
#11693=CARTESIAN_POINT ( 'NONE',  ( 151.6875000000000284, 4.242640687119269671, 4.242640687119298093 ) ) ;
#11694=VERTEX_POINT ( 'NONE', #29540 ) ;
#11698=EDGE_LOOP ( 'NONE', ( #2492, #410, #22541, #28577, #2197, #13001, #2866, #26130, #763, #25012, #10590, #8749, #2500, #15382, #18903, #16333 ) ) ;
#11699=DIRECTION ( 'NONE',  ( 0.000000000000000000, 0.000000000000000000, -1.000000000000000000 ) ) ;
#11702=CARTESIAN_POINT ( 'NONE',  ( 0.2138663749889929133, -15.56976101427718362, -7.989719758726499421 ) ) ;
#11704=DIRECTION ( 'NONE',  ( 1.000000000000000000, 0.000000000000000000, 0.000000000000000000 ) ) ;
#11707=FACE_OUTER_BOUND ( 'NONE', #8543, .T. ) ;
#11717=CARTESIAN_POINT ( 'NONE',  ( 130.0000000000000284, -60.00000000000001421, 4.000000000000003553 ) ) ;
#11720=ORIENTED_EDGE ( 'NONE', *, *, #15265, .F. ) ;
#11724=SURFACE_SIDE_STYLE ('',( #2324 ) ) ;
#11726=EDGE_CURVE ( 'NONE', #11694, #27377, #13927, .T. ) ;
#11728=STYLED_ITEM ( 'NONE', ( #12810 ), #3252 ) ;
#11730=CARTESIAN_POINT ( 'NONE',  ( 151.9613248654052029, -5.500000000000005329, 0.000000000000000000 ) ) ;
#11731=CARTESIAN_POINT ( 'NONE',  ( 134.6250000000000284, 0.000000000000000000, -6.000000000000005329 ) ) ;
#11740=CARTESIAN_POINT ( 'NONE',  ( 145.7663997308104342, -4.999999999999989342, -2.071067811865468400 ) ) ;
#11744=CARTESIAN_POINT ( 'NONE',  ( -4.999999999999920952, -65.00000000000001421, -7.500000000000007105 ) ) ;
#11748=FACE_OUTER_BOUND ( 'NONE', #28402, .T. ) ;
#11749=SURFACE_STYLE_FILL_AREA ( #25525 ) ;
#11757=ORIENTED_EDGE ( 'NONE', *, *, #29874, .T. ) ;
#11759=CARTESIAN_POINT ( 'NONE',  ( 137.2500000000000284, -6.000000000000005329, 0.000000000000000000 ) ) ;
#11763=ADVANCED_FACE ( 'NONE', ( #19866 ), #15765, .T. ) ;
#11764=CARTESIAN_POINT ( 'NONE',  ( 160.1101497308104058, 3.535533905932725318, 3.535533905932725318 ) ) ;
#11767=( BOUNDED_CURVE ( )  B_SPLINE_CURVE ( 2, ( #19312, #28631, #5592, #12563, #3141, #10243, #23908, #28942, #2851 ),
 .UNSPECIFIED., .F., .T. ) 
 B_SPLINE_CURVE_WITH_KNOTS ( ( 3, 2, 2, 2, 3 ),
 ( 0.4125000000000008105, 0.4187500000000006217, 0.4250000000000003775, 0.4312500000000001887, 0.4374999999999999445 ),
 .UNSPECIFIED. ) 
 CURVE ( )  GEOMETRIC_REPRESENTATION_ITEM ( )  RATIONAL_B_SPLINE_CURVE ( ( 0.9999999999999898970, 0.9238795325112968415, 1.000000000000000000, 0.9238795325112867385, 1.000000000000000000, 0.9238795325112867385, 1.000000000000000000, 0.9238795325112874046, 0.9999999999999993339 ) ) 
 REPRESENTATION_ITEM ( '' )  );
#11774=CIRCLE ( 'NONE', #24957, 1.000000000000000888 ) ;
#11775=CARTESIAN_POINT ( 'NONE',  ( 152.5386751345948539, -5.500000000000005329, 0.000000000000000000 ) ) ;
#11786=EDGE_CURVE ( 'NONE', #379, #1732, #14844, .T. ) ;
#11788=DIRECTION ( 'NONE',  ( 0.000000000000000000, 0.000000000000000000, -1.000000000000000000 ) ) ;
#11790=DIRECTION ( 'NONE',  ( -0.000000000000000000, -0.000000000000000000, -1.000000000000000000 ) ) ;
#11791=CARTESIAN_POINT ( 'NONE',  ( 145.7023502691896510, 0.000000000000000000, -5.000000000000004441 ) ) ;
#11794=CARTESIAN_POINT ( 'NONE',  ( 159.0937500000000284, 6.000000000000005329, 2.485281374238585972 ) ) ;
#11795=CARTESIAN_POINT ( 'NONE',  ( 144.2738248654052313, -3.889087296526011706, 3.889087296526011706 ) ) ;
#11803=CARTESIAN_POINT ( 'NONE',  ( 147.6562500000000284, -6.000000000000005329, 2.485281374238555774 ) ) ;
#11814=VERTEX_POINT ( 'NONE', #22643 ) ;
#11816=CARTESIAN_POINT ( 'NONE',  ( 158.2351497308104058, 3.535533905932725318, -3.535533905932725318 ) ) ;
#11819=AXIS2_PLACEMENT_3D ( 'NONE', #9239, #21229, #21382 ) ;
#11820=CARTESIAN_POINT ( 'NONE',  ( 135.5105870461044617, -9.078052452533968975, 8.000000000000007105 ) ) ;
#11821=AXIS2_PLACEMENT_3D ( 'NONE', #24327, #836, #10233 ) ;
#11823=CARTESIAN_POINT ( 'NONE',  ( 147.8363248654052029, 0.000000000000000000, -5.500000000000005329 ) ) ;
#11825=CIRCLE ( 'NONE', #1954, 12.00000000000000178 ) ;
#11827=ADVANCED_FACE ( 'NONE', ( #6034 ), #19977, .F. ) ;
#11829=PLANE ( 'NONE',  #16403 ) ;
#11830=CARTESIAN_POINT ( 'NONE',  ( -9.999999999999994671, -9.000000000000007105, 5.000000000000004441 ) ) ;
#11833=DIRECTION ( 'NONE',  ( 1.000000000000000000, -0.000000000000000000, -0.000000000000000000 ) ) ;
#11834=( LENGTH_UNIT ( ) NAMED_UNIT ( * ) SI_UNIT ( .MILLI., .METRE. ) );
#11848=CARTESIAN_POINT ( 'NONE',  ( 149.8125000000000568, 4.242640687119298093, -4.242640687119298093 ) ) ;
#11856=CARTESIAN_POINT ( 'NONE',  ( 131.7038997308104342, 2.071067811865468400, 4.999999999999989342 ) ) ;
#11858=CARTESIAN_POINT ( 'NONE',  ( 0.7667967985550546706, -15.49901982636443343, -8.125930293112922698 ) ) ;
#11865=CARTESIAN_POINT ( 'NONE',  ( -0.8012806810451161832, -9.198719318954823976, -4.013103574300090237 ) ) ;
#11867=MECHANICAL_DESIGN_GEOMETRIC_PRESENTATION_REPRESENTATION('',(#28458),#12829);
#11868=CARTESIAN_POINT ( 'NONE',  ( 160.9860446771581621, -11.61458924544450966, -3.019433540031084551 ) ) ;
#11869=EDGE_CURVE ( 'NONE', #12687, #8567, #29016, .T. ) ;
#11872=CARTESIAN_POINT ( 'NONE',  ( 134.9999999999992895, -6.982120021884475669, -8.500000000000007105 ) ) ;
#11876=CARTESIAN_POINT ( 'NONE',  ( 0.1991573574402268343, -15.94692260098227621, 7.215108609433896092 ) ) ;
#11880=VECTOR ( 'NONE', #351, 1000.000000000000000 ) ;
#11883=CYLINDRICAL_SURFACE ( 'NONE', #26827, 15.00000000000000000 ) ;
#11885=CARTESIAN_POINT ( 'NONE',  ( 140.5238248654052029, 3.889087296526011706, -3.889087296526011706 ) ) ;
#11888=CARTESIAN_POINT ( 'NONE',  ( 151.6800748654052029, -2.278174593052058938, 5.499999999999964473 ) ) ;
#11889=CARTESIAN_POINT ( 'NONE',  ( 134.1562500000000568, -6.000000000000005329, 2.485281374238555774 ) ) ;
#11896=CARTESIAN_POINT ( 'NONE',  ( -0.01457429254692333212, -14.38985900264256834, 8.358944243794823592 ) ) ;
#11899=CARTESIAN_POINT ( 'NONE',  ( 146.4226497308104342, 5.000000000000004441, 0.000000000000000000 ) ) ;
#11901=TOROIDAL_SURFACE ( 'NONE', #26544, 16.50000000000000355, 1.000000000000000000 ) ;
#11907=EDGE_CURVE ( 'NONE', #6421, #17999, #19720, .T. ) ;
#11908=( LENGTH_UNIT ( ) NAMED_UNIT ( * ) SI_UNIT ( .MILLI., .METRE. ) );
#11912=AXIS2_PLACEMENT_3D ( 'NONE', #20584, #29932, #8912 ) ;
#11916=CARTESIAN_POINT ( 'NONE',  ( 139.5000000000000284, -54.99999999999990763, 8.000000000000007105 ) ) ;
#11919=CARTESIAN_POINT ( 'NONE',  ( 141.2812500000000284, 2.485281374238585972, 6.000000000000005329 ) ) ;
#11921=CARTESIAN_POINT ( 'NONE',  ( 161.0000000000000284, 0.000000000000000000, 0.000000000000000000 ) ) ;
#11922=CARTESIAN_POINT ( 'NONE',  ( 135.0937500000000284, 6.000000000000005329, 2.485281374238585972 ) ) ;
#11927=ORIENTED_EDGE ( 'NONE', *, *, #6301, .F. ) ;
#11936=CARTESIAN_POINT ( 'NONE',  ( 152.1636751345948255, 0.000000000000000000, 5.500000000000005329 ) ) ;
#11938=CARTESIAN_POINT ( 'NONE',  ( 140.5000000000000284, -11.02592621076652790, 4.736429266082377687 ) ) ;
#11941=EDGE_CURVE ( 'NONE', #8039, #25268, #3820, .T. ) ;
#11942=EDGE_CURVE ( 'NONE', #17742, #1935, #18909, .T. ) ;
#11951=CARTESIAN_POINT ( 'NONE',  ( 143.7336002691896795, -4.999999999999989342, 2.071067811865468400 ) ) ;
#11952=CARTESIAN_POINT ( 'NONE',  ( 0.8619745489090032686, -15.74670610583283548, 7.642883928913009939 ) ) ;
#11953=CARTESIAN_POINT ( 'NONE',  ( 155.1562500000000284, -6.000000000000005329, 2.485281374238556218 ) ) ;
#11954=CARTESIAN_POINT ( 'NONE',  ( 160.0000000000000284, -59.99999999999980105, 3.000000000000002665 ) ) ;
#11961=CARTESIAN_POINT ( 'NONE',  ( 148.5000000000000284, 6.000000000000005329, 0.000000000000000000 ) ) ;
#11967=EDGE_LOOP ( 'NONE', ( #9031, #3769, #8472, #20570 ) ) ;
#11971=ORIENTED_EDGE ( 'NONE', *, *, #19553, .F. ) ;
#11972=CARTESIAN_POINT ( 'NONE',  ( 155.7038997308104058, 2.071067811865468400, 4.999999999999989342 ) ) ;
#11978=CARTESIAN_POINT ( 'NONE',  ( 143.8988248654052313, 3.889087296526011706, 3.889087296526011706 ) ) ;
#11984=CARTESIAN_POINT ( 'NONE',  ( 156.0148502691896510, -3.535533905932725318, -3.535533905932725318 ) ) ;
#11986=ORIENTED_EDGE ( 'NONE', *, *, #14124, .F. ) ;
#11989=DIRECTION ( 'NONE',  ( 0.000000000000000000, 0.000000000000000000, 1.000000000000000000 ) ) ;
#11991=CARTESIAN_POINT ( 'NONE',  ( 161.0701415566729509, 1.250657853440976686, 5.437060510562927718 ) ) ;
#11992=VERTEX_POINT ( 'NONE', #30241 ) ;
#11993=DIRECTION ( 'NONE',  ( 0.000000000000000000, 0.2307692307692307543, 0.9730085108210398959 ) ) ;
#11997=CARTESIAN_POINT ( 'NONE',  ( 148.0312500000000284, -2.485281374238555774, -6.000000000000005329 ) ) ;
#12003=ORIENTED_EDGE ( 'NONE', *, *, #20230, .T. ) ;
#12008=EDGE_CURVE ( 'NONE', #6343, #6339, #6237, .T. ) ;
#12013=CARTESIAN_POINT ( 'NONE',  ( 135.0000000000000284, -9.165151389911669000, 8.500000000000007105 ) ) ;
#12014=( NAMED_UNIT ( * ) SI_UNIT ( $, .STERADIAN. ) SOLID_ANGLE_UNIT ( ) );
#12015=LINE ( 'NONE', #18762, #14352 ) ;
#12017=DIRECTION ( 'NONE',  ( 0.000000000000000000, 0.000000000000000000, -1.000000000000000000 ) ) ;
#12021=DIRECTION ( 'NONE',  ( 1.000000000000000000, 0.000000000000000000, 0.000000000000000000 ) ) ;
#12024=EDGE_LOOP ( 'NONE', ( #20486, #16916, #21513, #20723 ) ) ;
#12031=ORIENTED_EDGE ( 'NONE', *, *, #10185, .T. ) ;
#12033=CARTESIAN_POINT ( 'NONE',  ( 137.2500000000000284, -6.000000000000005329, 0.000000000000000000 ) ) ;
#12037=VERTEX_POINT ( 'NONE', #24101 ) ;
#12039=SURFACE_STYLE_FILL_AREA ( #21378 ) ;
#12044=CARTESIAN_POINT ( 'NONE',  ( -4.999999999999886313, -14.50000000000001243, 7.500000000000007105 ) ) ;
#12045=CARTESIAN_POINT ( 'NONE',  ( 136.2038997308104058, 2.071067811865468400, 4.999999999999989342 ) ) ;
#12053=ORIENTED_EDGE ( 'NONE', *, *, #21571, .F. ) ;
#12055=DIRECTION ( 'NONE',  ( 0.000000000000000000, 1.000000000000000000, 0.000000000000000000 ) ) ;
#12059=DIRECTION ( 'NONE',  ( 1.000000000000000000, 0.000000000000000000, 0.000000000000000000 ) ) ;
#12063=CARTESIAN_POINT ( 'NONE',  ( 132.0000000000000284, 6.000000000000005329, 0.000000000000000000 ) ) ;
#12067=EDGE_CURVE ( 'NONE', #3090, #25526, #16483, .T. ) ;
#12069=CIRCLE ( 'NONE', #14516, 29.00000000000000000 ) ;
#12072=CIRCLE ( 'NONE', #28688, 16.50000000000000355 ) ;
#12075=CARTESIAN_POINT ( 'NONE',  ( 159.9752036821340653, -12.51993663517088429, -3.254295310666532437 ) ) ;
#12077=DIRECTION ( 'NONE',  ( 0.000000000000000000, 0.000000000000000000, -1.000000000000000000 ) ) ;
#12080=CARTESIAN_POINT ( 'NONE',  ( 140.6818792730027496, -11.36375854600486690, -4.222310544175439162 ) ) ;
#12083=CARTESIAN_POINT ( 'NONE',  ( 140.0000000000000000, -9.600000000000004974, 7.199999999999999289 ) ) ;
#12091=CARTESIAN_POINT ( 'NONE',  ( 139.7187733625200394, -9.255022275057855907, 7.951101893190698711 ) ) ;
#12092=CARTESIAN_POINT ( 'NONE',  ( 160.8750000000000568, 0.000000000000000000, 6.000000000000005329 ) ) ;
#12095=SURFACE_STYLE_USAGE ( .BOTH. , #2529 ) ;
#12096=CARTESIAN_POINT ( 'NONE',  ( 1.000000000000000888, 0.000000000000000000, 0.000000000000000000 ) ) ;
#12098=DIRECTION ( 'NONE',  ( 0.000000000000000000, 0.000000000000000000, -1.000000000000000000 ) ) ;
#12100=CARTESIAN_POINT ( 'NONE',  ( 148.9687500000000284, -2.485281374238585972, 6.000000000000005329 ) ) ;
#12102=CARTESIAN_POINT ( 'NONE',  ( 0.000000000000000000, 0.000000000000000000, 8.500000000000007105 ) ) ;
#12104=EDGE_CURVE ( 'NONE', #3609, #3090, #28536, .T. ) ;
#12109=STYLED_ITEM ( 'NONE', ( #15676 ), #7443 ) ;
#12113=FILL_AREA_STYLE_COLOUR ( '', #22619 ) ;
#12114=CARTESIAN_POINT ( 'NONE',  ( 153.4538997308104058, -2.071067811865468400, -4.999999999999989342 ) ) ;
#12115=AXIS2_PLACEMENT_3D ( 'NONE', #21577, #12380, #14962 ) ;
#12123=CARTESIAN_POINT ( 'NONE',  ( 140.6185434356032715, -11.23708687120643646, 4.230991509104588211 ) ) ;
#12125=CARTESIAN_POINT ( 'NONE',  ( 142.2113248654052313, 5.500000000000005329, 0.000000000000000000 ) ) ;
#12126=CARTESIAN_POINT ( 'NONE',  ( 161.5000000000000853, -2.984449860524901688, -5.205099329504969674 ) ) ;
#12130=UNCERTAINTY_MEASURE_WITH_UNIT (LENGTH_MEASURE( 1.000000000000000082E-05 ), #678, 'distance_accuracy_value', 'NONE');
#12132=ADVANCED_FACE ( 'NONE', ( #4902 ), #302, .T. ) ;
#12133=CARTESIAN_POINT ( 'NONE',  ( -0.5000000000000004441, -10.50000000000000888, 7.500000000000007105 ) ) ;
#12140=VERTEX_POINT ( 'NONE', #14758 ) ;
#12142=CARTESIAN_POINT ( 'NONE',  ( 145.3125000000000284, 4.242640687119298093, -4.242640687119298093 ) ) ;
#12147=UNCERTAINTY_MEASURE_WITH_UNIT (LENGTH_MEASURE( 1.000000000000000082E-05 ), #28013, 'distance_accuracy_value', 'NONE');
#12152=CARTESIAN_POINT ( 'NONE',  ( 132.8288997308104342, 4.999999999999989342, -2.071067811865468400 ) ) ;
#12155=CARTESIAN_POINT ( 'NONE',  ( 158.4449251345948255, -5.500000000000012434, 2.278174593052012309 ) ) ;
#12156=FACE_OUTER_BOUND ( 'NONE', #29378, .T. ) ;
#12163=UNCERTAINTY_MEASURE_WITH_UNIT (LENGTH_MEASURE( 1.000000000000000082E-05 ), #769, 'distance_accuracy_value', 'NONE');
#12165=CARTESIAN_POINT ( 'NONE',  ( 135.0000000000000284, -9.047800747816998168, -7.500000000000007105 ) ) ;
#12169=CARTESIAN_POINT ( 'NONE',  ( -2.117582368135750848E-19, -15.46244542726873306, -5.965557206115555289 ) ) ;
#12172=CARTESIAN_POINT ( 'NONE',  ( -4.999999999999886313, -14.50000000000001243, 8.000000000000007105 ) ) ;
#12173=TOROIDAL_SURFACE ( 'NONE', #16574, 16.50000000000000355, 1.000000000000000000 ) ;
#12174=AXIS2_PLACEMENT_3D ( 'NONE', #15245, #13113, #8293 ) ;
#12176=STYLED_ITEM ( 'NONE', ( #15736 ), #6884 ) ;
#12177=SURFACE_SIDE_STYLE ('',( #10142 ) ) ;
#12179=( BOUNDED_SURFACE ( )  B_SPLINE_SURFACE ( 3, 2, ( 
 ( #28263, #19090, #18790 ),
 ( #16352, #4776, #7391 ),
 ( #11896, #318, #7242 ),
 ( #16650, #463, #12336 ) ),
 .UNSPECIFIED., .F., .F., .F. ) 
 B_SPLINE_SURFACE_WITH_KNOTS ( ( 4, 4 ),
 ( 3, 3 ),
 ( 0.005369593351152912065, 0.006104230743885358246 ),
 ( 0.000000000000000000, 1.000000000000000000 ),
 .UNSPECIFIED. ) 
 GEOMETRIC_REPRESENTATION_ITEM ( )  RATIONAL_B_SPLINE_SURFACE ( (
 ( 1.000000000000000000, 0.7071067811865475727, 1.000000000000000000),
 ( 1.000000000000000000, 0.7328765725615882243, 1.000000000000000000),
 ( 1.000000000000000000, 0.7551281783742019860, 1.000000000000000000),
 ( 1.000000000000000000, 0.7743236465966906179, 1.000000000000000000) ) ) 
 REPRESENTATION_ITEM ( '' )  SURFACE ( )  );
#12180=DIRECTION ( 'NONE',  ( 0.000000000000000000, 0.000000000000000000, -1.000000000000000000 ) ) ;
#12181=ORIENTED_EDGE ( 'NONE', *, *, #17955, .T. ) ;
#12182=EDGE_CURVE ( 'NONE', #20260, #29031, #3454, .T. ) ;
#12184=AXIS2_PLACEMENT_3D ( 'NONE', #9215, #6444, #18606 ) ;
#12185=ORIENTED_EDGE ( 'NONE', *, *, #10200, .F. ) ;
#12186=EDGE_LOOP ( 'NONE', ( #10696, #8897, #7480, #8613 ) ) ;
#12188=CARTESIAN_POINT ( 'NONE',  ( 135.9523502691896510, 0.000000000000000000, 5.000000000000004441 ) ) ;
#12193=ORIENTED_EDGE ( 'NONE', *, *, #1820, .F. ) ;
#12194=AXIS2_PLACEMENT_3D ( 'NONE', #7616, #15008, #850 ) ;
#12195=FACE_OUTER_BOUND ( 'NONE', #8179, .T. ) ;
#12197=CARTESIAN_POINT ( 'NONE',  ( 140.7038997308104058, 2.071067811865468400, 4.999999999999989342 ) ) ;
#12198=DIRECTION ( 'NONE',  ( -0.000000000000000000, 1.000000000000000000, -0.000000000000000000 ) ) ;
#12204=VECTOR ( 'NONE', #19826, 1000.000000000000000 ) ;
#12210=EDGE_CURVE ( 'NONE', #22270, #9839, #17037, .T. ) ;
#12211=ORIENTED_EDGE ( 'NONE', *, *, #25214, .T. ) ;
#12214=( GEOMETRIC_REPRESENTATION_CONTEXT ( 3 ) GLOBAL_UNCERTAINTY_ASSIGNED_CONTEXT ( ( #523 ) ) GLOBAL_UNIT_ASSIGNED_CONTEXT ( ( #26176, #374, #7442 ) ) REPRESENTATION_CONTEXT ( 'NONE', 'WORKASPACE' ) );
#12218=CARTESIAN_POINT ( 'NONE',  ( 161.3288997308104626, 4.999999999999989342, -2.071067811865468400 ) ) ;
#12222=CIRCLE ( 'NONE', #7736, 0.5000000000000004441 ) ;
#12232=CARTESIAN_POINT ( 'NONE',  ( 140.5384615384615756, -11.07692307692306777, 4.615384615384604317 ) ) ;
#12238=CARTESIAN_POINT ( 'NONE',  ( 146.5238248654052029, 3.889087296526011706, -3.889087296526011706 ) ) ;
#12243=CARTESIAN_POINT ( 'NONE',  ( 144.7648502691896510, 3.535533905932725318, 3.535533905932752852 ) ) ;
#12244=CARTESIAN_POINT ( 'NONE',  ( -4.999999999999990230, -24.99999999999999289, 7.500000000000007105 ) ) ;
#12245=CARTESIAN_POINT ( 'NONE',  ( 150.6562500000000568, -6.000000000000005329, 2.485281374238556218 ) ) ;
#12246=DIRECTION ( 'NONE',  ( 0.000000000000000000, 1.000000000000000000, -0.000000000000000000 ) ) ;
#12251=CARTESIAN_POINT ( 'NONE',  ( 150.6562500000000284, -6.000000000000005329, 2.485281374238555774 ) ) ;
#12257=VERTEX_POINT ( 'NONE', #29298 ) ;
#12260=EDGE_CURVE ( 'NONE', #42, #4270, #21659, .T. ) ;
#12270=CARTESIAN_POINT ( 'NONE',  ( 140.7917870674316987, -11.58357413486331566, 4.000000000000005329 ) ) ;
#12273=CARTESIAN_POINT ( 'NONE',  ( 145.1324251345948539, -5.500000000000012434, -2.278174593052012309 ) ) ;
#12276=CARTESIAN_POINT ( 'NONE',  ( 135.6488248654052597, -3.889087296526011706, -3.889087296526011706 ) ) ;
#12277=CARTESIAN_POINT ( 'NONE',  ( 157.7023502691896510, 0.000000000000000000, -5.000000000000004441 ) ) ;
#12288=CARTESIAN_POINT ( 'NONE',  ( 145.2187500000000000, 2.485281374238555774, -6.000000000000005329 ) ) ;
#12290=VECTOR ( 'NONE', #22390, 1000.000000000000000 ) ;
#12294=AXIS2_PLACEMENT_3D ( 'NONE', #20460, #10968, #29819 ) ;
#12298=CARTESIAN_POINT ( 'NONE',  ( 134.0476497308104058, 0.000000000000000000, -5.000000000000004441 ) ) ;
#12301=ORIENTED_EDGE ( 'NONE', *, *, #11615, .F. ) ;
#12302=FACE_OUTER_BOUND ( 'NONE', #3504, .T. ) ;
#12316=ORIENTED_EDGE ( 'NONE', *, *, #21573, .T. ) ;
#12317=CARTESIAN_POINT ( 'NONE',  ( 0.1950273200666236550, -15.66255992321437951, 7.807776097887586531 ) ) ;
#12318=MECHANICAL_DESIGN_GEOMETRIC_PRESENTATION_REPRESENTATION('',(#25508),#10838);
#12320=AXIS2_PLACEMENT_3D ( 'NONE', #7314, #9057, #26046 ) ;
#12321=ORIENTED_EDGE ( 'NONE', *, *, #22224, .T. ) ;
#12325=ORIENTED_EDGE ( 'NONE', *, *, #18332, .T. ) ;
#12328=CARTESIAN_POINT ( 'NONE',  ( 160.7812500000000568, 2.485281374238585972, 6.000000000000005329 ) ) ;
#12331=DIRECTION ( 'NONE',  ( 1.734723475976843579E-16, -1.000000000000000000, 0.000000000000000000 ) ) ;
#12333=DIRECTION ( 'NONE',  ( 1.000000000000000000, 0.000000000000000000, 0.000000000000000000 ) ) ;
#12336=CARTESIAN_POINT ( 'NONE',  ( 0.8631338372299254269, -15.37878787878792686, 8.351220472436690301 ) ) ;
#12337=CARTESIAN_POINT ( 'NONE',  ( 139.9538997308103774, -2.071067811865468400, -4.999999999999989342 ) ) ;
#12342=EDGE_CURVE ( 'NONE', #13173, #14623, #15287, .T. ) ;
#12344=VECTOR ( 'NONE', #10044, 1000.000000000000000 ) ;
#12346=ORIENTED_EDGE ( 'NONE', *, *, #2292, .F. ) ;
#12358=DIRECTION ( 'NONE',  ( 1.000000000000000000, 0.000000000000000000, 0.000000000000000000 ) ) ;
#12365=DIRECTION ( 'NONE',  ( -1.000000000000000000, 0.000000000000000000, 0.000000000000000000 ) ) ;
#12366=CARTESIAN_POINT ( 'NONE',  ( 140.5126539824821634, -11.05214782318283184, -4.674845224361170004 ) ) ;
#12368=ADVANCED_FACE ( 'NONE', ( #13529 ), #27748, .F. ) ;
#12372=CARTESIAN_POINT ( 'NONE',  ( 140.4831164018241054, -11.48311640182297388, -4.126236462591093002 ) ) ;
#12373=( GEOMETRIC_REPRESENTATION_CONTEXT ( 3 ) GLOBAL_UNCERTAINTY_ASSIGNED_CONTEXT ( ( #18916 ) ) GLOBAL_UNIT_ASSIGNED_CONTEXT ( ( #19637, #7356, #4883 ) ) REPRESENTATION_CONTEXT ( 'NONE', 'WORKASPACE' ) );
#12374=LINE ( 'NONE', #21722, #12344 ) ;
#12377=CARTESIAN_POINT ( 'NONE',  ( 139.8749506744242410, -9.075050735211396713, 7.854018104365544595 ) ) ;
#12378=CIRCLE ( 'NONE', #29505, 28.99999999999999645 ) ;
#12380=DIRECTION ( 'NONE',  ( 0.000000000000000000, 1.000000000000000000, -1.224646799147353207E-16 ) ) ;
#12381=CARTESIAN_POINT ( 'NONE',  ( 146.4300748654051745, 2.278174593051733421, -5.500000000000292211 ) ) ;
#12387=CARTESIAN_POINT ( 'NONE',  ( 146.0773502691896510, 5.000000000000004441, 0.000000000000000000 ) ) ;
#12389=CARTESIAN_POINT ( 'NONE',  ( 150.9375000000000284, -4.242640687119298093, -4.242640687119298093 ) ) ;
#12390=DIRECTION ( 'NONE',  ( 0.7071067811865555663, 8.659560562354835483E-17, 0.7071067811865394681 ) ) ;
#12395=CARTESIAN_POINT ( 'NONE',  ( 143.1562500000000284, -6.000000000000005329, 2.485281374238555774 ) ) ;
#12396=AXIS2_PLACEMENT_3D ( 'NONE', #14203, #6634, #25830 ) ;
#12401=ORIENTED_EDGE ( 'NONE', *, *, #12104, .T. ) ;
#12405=EDGE_CURVE ( 'NONE', #14826, #5798, #682, .T. ) ;
#12412=CARTESIAN_POINT ( 'NONE',  ( 134.9273262448254798, -7.354674723977097983, 8.000000000000005329 ) ) ;
#12418=CARTESIAN_POINT ( 'NONE',  ( 145.0386751345948539, -5.500000000000005329, 0.000000000000000000 ) ) ;
#12420=CARTESIAN_POINT ( 'NONE',  ( 157.6086002691896795, -2.071067811865468400, -4.999999999999989342 ) ) ;
#12422=DIRECTION ( 'NONE',  ( -0.000000000000000000, -0.000000000000000000, 1.000000000000000000 ) ) ;
#12427=VERTEX_POINT ( 'NONE', #7336 ) ;
#12431=EDGE_LOOP ( 'NONE', ( #10687, #14120, #8504, #30388 ) ) ;
#12433=B_SPLINE_CURVE_WITH_KNOTS ( 'NONE', 3,
 ( #10433, #5190, #17358, #26674, #19354, #22099, #17505, #1033, #5635, #9977, #21948, #23801 ),
 .UNSPECIFIED., .F., .F.,
 ( 4, 2, 2, 2, 2, 4 ),
 ( 0.000000000000000000, 0.0005736249320795650149, 0.001147249864159130030, 0.001720874796238695045, 0.002007687262278479504, 0.002294499728318263529 ),
 .UNSPECIFIED. ) ;
#12436=ADVANCED_FACE ( 'NONE', ( #26358 ), #4720, .F. ) ;
#12443=CARTESIAN_POINT ( 'NONE',  ( 132.1726497308104058, -5.000000000000004441, 0.000000000000000000 ) ) ;
#12446=CARTESIAN_POINT ( 'NONE',  ( 0.1513474785670624878, -15.31721424822544542, -8.468282902864297412 ) ) ;
#12448=CARTESIAN_POINT ( 'NONE',  ( -4.999999999999886313, -10.50000000000000888, -7.500000000000007105 ) ) ;
#12449=CARTESIAN_POINT ( 'NONE',  ( 141.3675748654052313, -5.500000000000012434, 2.278174593052012309 ) ) ;
#12452=CARTESIAN_POINT ( 'NONE',  ( 153.0863248654052313, 0.000000000000000000, 5.500000000000005329 ) ) ;
#12454=LINE ( 'NONE', #14465, #6740 ) ;
#12457=CARTESIAN_POINT ( 'NONE',  ( 159.7574251345948824, -2.278174593051888408, 5.500000000000135891 ) ) ;
#12459=( LENGTH_UNIT ( ) NAMED_UNIT ( * ) SI_UNIT ( .MILLI., .METRE. ) );
#12461=CARTESIAN_POINT ( 'NONE',  ( 148.8824251345948824, 5.500000000000012434, 2.278174593052012309 ) ) ;
#12465=CARTESIAN_POINT ( 'NONE',  ( 0.000000000000000000, 10.00000000000000888, 3.000000000000002665 ) ) ;
#12468=ORIENTED_EDGE ( 'NONE', *, *, #12853, .F. ) ;
#12474=EDGE_LOOP ( 'NONE', ( #15679, #8740, #6992, #1045 ) ) ;
#12478=CARTESIAN_POINT ( 'NONE',  ( 132.3750000000000284, 0.000000000000000000, 6.000000000000005329 ) ) ;
#12479=CARTESIAN_POINT ( 'NONE',  ( 133.3273502691896510, -5.000000000000004441, 0.000000000000000000 ) ) ;
#12480=EDGE_CURVE ( 'NONE', #1192, #15961, #2985, .T. ) ;
#12483=ORIENTED_EDGE ( 'NONE', *, *, #11942, .T. ) ;
#12485=SURFACE_SIDE_STYLE ('',( #12039 ) ) ;
#12492=SURFACE_SIDE_STYLE ('',( #1070 ) ) ;
#12493=CARTESIAN_POINT ( 'NONE',  ( 135.1726497308104058, -5.000000000000004441, 0.000000000000000000 ) ) ;
#12500=( LENGTH_UNIT ( ) NAMED_UNIT ( * ) SI_UNIT ( .MILLI., .METRE. ) );
#12501=VERTEX_POINT ( 'NONE', #16743 ) ;
#12506=CARTESIAN_POINT ( 'NONE',  ( 136.8750000000000284, 0.000000000000000000, 6.000000000000005329 ) ) ;
#12507=EDGE_CURVE ( 'NONE', #765, #12660, #9345, .T. ) ;
#12509=SURFACE_SIDE_STYLE ('',( #8002 ) ) ;
#12510=LINE ( 'NONE', #22302, #24371 ) ;
#12512=CARTESIAN_POINT ( 'NONE',  ( 140.1146164139961456, -11.55730820707152695, 4.524920606409397195 ) ) ;
#12513=VECTOR ( 'NONE', #3189, 1000.000000000000000 ) ;
#12521=CARTESIAN_POINT ( 'NONE',  ( 137.0699251345947971, 2.278174593052352925, 5.499999999999671374 ) ) ;
#12527=LINE ( 'NONE', #23722, #27986 ) ;
#12530=CARTESIAN_POINT ( 'NONE',  ( 140.0346817368759673, -9.544509217149149904, 7.273987717135122821 ) ) ;
#12531=DIRECTION ( 'NONE',  ( 1.000000000000000000, -0.000000000000000000, -0.000000000000000000 ) ) ;
#12532=SURFACE_STYLE_USAGE ( .BOTH. , #14822 ) ;
#12536=CARTESIAN_POINT ( 'NONE',  ( 140.9211002691896510, -4.999999999999989342, -2.071067811865468400 ) ) ;
#12537=CARTESIAN_POINT ( 'NONE',  ( 149.4375000000000284, -4.242640687119298093, -4.242640687119298093 ) ) ;
#12543=CARTESIAN_POINT ( 'NONE',  ( 141.9375000000000284, -4.242640687119298093, -4.242640687119298093 ) ) ;
#12546=DIRECTION ( 'NONE',  ( 0.000000000000000000, 0.000000000000000000, -1.000000000000000000 ) ) ;
#12550=( NAMED_UNIT ( * ) SI_UNIT ( $, .STERADIAN. ) SOLID_ANGLE_UNIT ( ) );
#12554=CARTESIAN_POINT ( 'NONE',  ( 136.0000000000000284, -9.165151389911695645, -8.000000000000007105 ) ) ;
#12555=( NAMED_UNIT ( * ) SI_UNIT ( $, .STERADIAN. ) SOLID_ANGLE_UNIT ( ) );
#12560=CARTESIAN_POINT ( 'NONE',  ( 143.7113248654052313, 5.500000000000005329, 0.000000000000000000 ) ) ;
#12563=CARTESIAN_POINT ( 'NONE',  ( 149.0550748654052029, -5.500000000000012434, -2.278174593052012309 ) ) ;
#12569=DIRECTION ( 'NONE',  ( -1.000000000000000000, 0.000000000000000000, 0.000000000000000000 ) ) ;
#12572=CARTESIAN_POINT ( 'NONE',  ( 1.000000000000000888, -14.99923475244191451, -9.015151515151503148 ) ) ;
#12574=SURFACE_STYLE_USAGE ( .BOTH. , #7472 ) ;
#12578=VECTOR ( 'NONE', #2131, 1000.000000000000000 ) ;
#12579=CARTESIAN_POINT ( 'NONE',  ( 160.4062500000000284, 6.000000000000005329, -2.485281374238555774 ) ) ;
#12580=CARTESIAN_POINT ( 'NONE',  ( 161.0000000000000284, -12.64911064067353408, 3.000000000000002665 ) ) ;
#12588=VERTEX_POINT ( 'NONE', #28359 ) ;
#12592=DIRECTION ( 'NONE',  ( 0.000000000000000000, 0.000000000000000000, -1.000000000000000000 ) ) ;
#12594=ORIENTED_EDGE ( 'NONE', *, *, #29730, .F. ) ;
#12596=CARTESIAN_POINT ( 'NONE',  ( 141.7425748654051745, -2.278174593052322283, -5.499999999999701572 ) ) ;
#12599=( GEOMETRIC_REPRESENTATION_CONTEXT ( 3 ) GLOBAL_UNCERTAINTY_ASSIGNED_CONTEXT ( ( #21337 ) ) GLOBAL_UNIT_ASSIGNED_CONTEXT ( ( #21194, #2584, #7353 ) ) REPRESENTATION_CONTEXT ( 'NONE', 'WORKASPACE' ) );
#12609=CARTESIAN_POINT ( 'NONE',  ( 148.6011751345948539, 3.889087296526011706, -3.889087296526011706 ) ) ;
#12613=DIRECTION ( 'NONE',  ( 1.000000000000000000, 0.000000000000000000, 0.000000000000000000 ) ) ;
#12614=EDGE_CURVE ( 'NONE', #15017, #6232, #2572, .T. ) ;
#12615=ORIENTED_EDGE ( 'NONE', *, *, #20191, .T. ) ;
#12619=ORIENTED_EDGE ( 'NONE', *, *, #10474, .T. ) ;
#12622=CARTESIAN_POINT ( 'NONE',  ( 161.9062500000000568, 6.000000000000005329, -2.485281374238555774 ) ) ;
#12624=DIRECTION ( 'NONE',  ( 0.000000000000000000, 0.000000000000000000, 1.000000000000000000 ) ) ;
#12625=CARTESIAN_POINT ( 'NONE',  ( -9.999999999999779732, -89.00000000000001421, -4.000000000000003553 ) ) ;
#12628=CARTESIAN_POINT ( 'NONE',  ( 149.3511751345948255, -3.889087296526011706, 3.889087296526011706 ) ) ;
#12630=CARTESIAN_POINT ( 'NONE',  ( 139.6726497308104342, -5.000000000000004441, 0.000000000000000000 ) ) ;
#12635=CARTESIAN_POINT ( 'NONE',  ( -0.5000000000000004441, -14.50000000000001243, 7.500000000000007105 ) ) ;
#12639=CARTESIAN_POINT ( 'NONE',  ( 135.0000000000000284, 0.000000000000000000, 0.000000000000000000 ) ) ;
#12640=CARTESIAN_POINT ( 'NONE',  ( 153.6636751345948255, 0.000000000000000000, 5.500000000000005329 ) ) ;
#12642=VERTEX_POINT ( 'NONE', #7765 ) ;
#12646=DIRECTION ( 'NONE',  ( -1.000000000000000000, -0.000000000000000000, -0.000000000000000000 ) ) ;
#12654=( BOUNDED_CURVE ( )  B_SPLINE_CURVE ( 2, ( #16225, #28285, #14222, #6953, #18660, #7264, #25539, #20953, #2207 ),
 .UNSPECIFIED., .F., .T. ) 
 B_SPLINE_CURVE_WITH_KNOTS ( ( 3, 2, 2, 2, 3 ),
 ( 0.3374999999999998557, 0.3437499999999996114, 0.3499999999999993117, 0.3562499999999990674, 0.3624999999999989342 ),
 .UNSPECIFIED. ) 
 CURVE ( )  GEOMETRIC_REPRESENTATION_ITEM ( )  RATIONAL_B_SPLINE_CURVE ( ( 1.000000000000001998, 0.9238795325112847401, 1.000000000000000000, 0.9238795325112867385, 1.000000000000000000, 0.9238795325112867385, 1.000000000000000000, 0.9238795325113002832, 0.9999999999999864553 ) ) 
 REPRESENTATION_ITEM ( '' )  );
#12655=CARTESIAN_POINT ( 'NONE',  ( 124.9999999999999432, -65.50000000000000000, -8.000000000000007105 ) ) ;
#12657=AXIS2_PLACEMENT_3D ( 'NONE', #5737, #22044, #10853 ) ;
#12658=CARTESIAN_POINT ( 'NONE',  ( 140.0769230769231228, -11.53846153846154898, 4.615384615384614087 ) ) ;
#12659=AXIS2_PLACEMENT_3D ( 'NONE', #9418, #29990, #4493 ) ;
#12660=VERTEX_POINT ( 'NONE', #19911 ) ;
#12662=ORIENTED_EDGE ( 'NONE', *, *, #8184, .F. ) ;
#12670=CARTESIAN_POINT ( 'NONE',  ( 158.5163997308104342, 4.999999999999989342, 2.071067811865468400 ) ) ;
#12671=VECTOR ( 'NONE', #27328, 1000.000000000000000 ) ;
#12674=CARTESIAN_POINT ( 'NONE',  ( 15.00000000000000000, 2.143131898507868643E-15, -17.50000000000000355 ) ) ;
#12675=FILL_AREA_STYLE ('',( #29053 ) ) ;
#12676=CARTESIAN_POINT ( 'NONE',  ( 135.5000000000000000, -9.047800747817552391, 8.000000000000007105 ) ) ;
#12681=DIRECTION ( 'NONE',  ( 1.000000000000000000, 0.000000000000000000, 0.000000000000000000 ) ) ;
#12682=( GEOMETRIC_REPRESENTATION_CONTEXT ( 3 ) GLOBAL_UNCERTAINTY_ASSIGNED_CONTEXT ( ( #16736 ) ) GLOBAL_UNIT_ASSIGNED_CONTEXT ( ( #21866, #21570, #25865 ) ) REPRESENTATION_CONTEXT ( 'NONE', 'WORKASPACE' ) );
#12687=VERTEX_POINT ( 'NONE', #3154 ) ;
#12688=CARTESIAN_POINT ( 'NONE',  ( 136.8898502691896510, 3.535533905932725318, -3.535533905932725318 ) ) ;
#12689=CARTESIAN_POINT ( 'NONE',  ( 154.2187500000000568, 2.485281374238556218, -6.000000000000005329 ) ) ;
#12694=ORIENTED_EDGE ( 'NONE', *, *, #2523, .T. ) ;
#12695=CARTESIAN_POINT ( 'NONE',  ( 141.3750000000000284, 0.000000000000000000, 6.000000000000005329 ) ) ;
#12696=CARTESIAN_POINT ( 'NONE',  ( 142.9613248654052597, -5.500000000000005329, 0.000000000000000000 ) ) ;
#12697=AXIS2_PLACEMENT_3D ( 'NONE', #1823, #24863, #27606 ) ;
#12698=DIRECTION ( 'NONE',  ( 1.000000000000000000, -0.000000000000000000, -0.000000000000000000 ) ) ;
#12702=VERTEX_POINT ( 'NONE', #19759 ) ;
#12706=EDGE_CURVE ( 'NONE', #22119, #12588, #17860, .T. ) ;
#12707=SURFACE_STYLE_FILL_AREA ( #14988 ) ;
#12708=DIRECTION ( 'NONE',  ( -1.000000000000000000, -1.734723475976843579E-16, 0.000000000000000000 ) ) ;
#12710=LINE ( 'NONE', #22046, #18180 ) ;
#12717=CARTESIAN_POINT ( 'NONE',  ( 142.3050748654052597, 5.500000000000012434, 2.278174593052012309 ) ) ;
#12718=FILL_AREA_STYLE_COLOUR ( '', #29962 ) ;
#12721=CARTESIAN_POINT ( 'NONE',  ( 135.4613248654052313, -5.500000000000005329, 0.000000000000000000 ) ) ;
#12722=CARTESIAN_POINT ( 'NONE',  ( 151.6086002691896795, -2.071067811865468400, -4.999999999999989342 ) ) ;
#12723=CARTESIAN_POINT ( 'NONE',  ( 139.7195358716536475, -9.255744405766421323, -7.950703011861615543 ) ) ;
#12730=CARTESIAN_POINT ( 'NONE',  ( -0.04481861813794070504, -15.28417525976993652, 7.195112359326359730 ) ) ;
#12743=EDGE_CURVE ( 'NONE', #28619, #11692, #17944, .T. ) ;
#12745=( GEOMETRIC_REPRESENTATION_CONTEXT ( 3 ) GLOBAL_UNCERTAINTY_ASSIGNED_CONTEXT ( ( #9643 ) ) GLOBAL_UNIT_ASSIGNED_CONTEXT ( ( #14009, #14163, #20885 ) ) REPRESENTATION_CONTEXT ( 'NONE', 'WORKASPACE' ) );
#12747=CARTESIAN_POINT ( 'NONE',  ( -0.06480180424034547026, -14.68233348625668988, -8.233331871529086854 ) ) ;
#12759=DIRECTION ( 'NONE',  ( 1.000000000000000000, -0.000000000000000000, -0.000000000000000000 ) ) ;
#12761=FACE_OUTER_BOUND ( 'NONE', #4392, .T. ) ;
#12771=ORIENTED_EDGE ( 'NONE', *, *, #16966, .T. ) ;
#12775=CARTESIAN_POINT ( 'NONE',  ( 135.7648502691896510, 3.535533905932725318, 3.535533905932752852 ) ) ;
#12776=ORIENTED_EDGE ( 'NONE', *, *, #13847, .F. ) ;
#12783=CARTESIAN_POINT ( 'NONE',  ( 140.0000000000000284, -11.45643923738959202, -5.000000000000004441 ) ) ;
#12787=CARTESIAN_POINT ( 'NONE',  ( -0.01452156813450973180, -14.38967195594448611, -8.359059054233915376 ) ) ;
#12790=( NAMED_UNIT ( * ) SI_UNIT ( $, .STERADIAN. ) SOLID_ANGLE_UNIT ( ) );
#12792=LINE ( 'NONE', #3672, #19517 ) ;
#12794=MECHANICAL_DESIGN_GEOMETRIC_PRESENTATION_REPRESENTATION('',(#27467),#4418);
#12796=DIRECTION ( 'NONE',  ( 0.000000000000000000, 0.000000000000000000, -1.000000000000000000 ) ) ;
#12797=CARTESIAN_POINT ( 'NONE',  ( 154.4136751345948539, 0.000000000000000000, -5.500000000000005329 ) ) ;
#12798=ORIENTED_EDGE ( 'NONE', *, *, #10802, .T. ) ;
#12801=DIRECTION ( 'NONE',  ( -0.000000000000000000, -0.000000000000000000, -1.000000000000000000 ) ) ;
#12804=DIRECTION ( 'NONE',  ( 0.000000000000000000, 0.000000000000000000, -1.000000000000000000 ) ) ;
#12808=DIRECTION ( 'NONE',  ( 1.000000000000000000, -0.000000000000000000, -0.000000000000000000 ) ) ;
#12810=PRESENTATION_STYLE_ASSIGNMENT (( #21997 ) ) ;
#12815=CARTESIAN_POINT ( 'NONE',  ( 160.7356042043084585, -11.41176159196295004, 3.718407753375058800 ) ) ;
#12817=DIRECTION ( 'NONE',  ( 1.000000000000000000, 0.000000000000000000, 0.000000000000000000 ) ) ;
#12822=CARTESIAN_POINT ( 'NONE',  ( 151.0163997308104058, 4.999999999999989342, 2.071067811865468400 ) ) ;
#12824=( NAMED_UNIT ( * ) SI_UNIT ( $, .STERADIAN. ) SOLID_ANGLE_UNIT ( ) );
#12828=LINE ( 'NONE', #19713, #22870 ) ;
#12829=( GEOMETRIC_REPRESENTATION_CONTEXT ( 3 ) GLOBAL_UNCERTAINTY_ASSIGNED_CONTEXT ( ( #16770 ) ) GLOBAL_UNIT_ASSIGNED_CONTEXT ( ( #4619, #172, #15898 ) ) REPRESENTATION_CONTEXT ( 'NONE', 'WORKASPACE' ) );
#12833=AXIS2_PLACEMENT_3D ( 'NONE', #108, #9489, #4706 ) ;
#12835=ORIENTED_EDGE ( 'NONE', *, *, #3402, .T. ) ;
#12836=CARTESIAN_POINT ( 'NONE',  ( 153.8437500000000284, -6.000000000000005329, -2.485281374238556218 ) ) ;
#12841=CARTESIAN_POINT ( 'NONE',  ( 142.2187500000000284, 2.485281374238555774, -6.000000000000005329 ) ) ;
#12842=CARTESIAN_POINT ( 'NONE',  ( 161.3705918646423925, -5.766246672886522262, -1.146283980155012205 ) ) ;
#12843=ADVANCED_FACE ( 'NONE', ( #7064 ), #5343, .T. ) ;
#12853=EDGE_CURVE ( 'NONE', #12642, #13611, #5948, .T. ) ;
#12855=EDGE_CURVE ( 'NONE', #5798, #17671, #25142, .T. ) ;
#12856=CIRCLE ( 'NONE', #1040, 2.000000000000000000 ) ;
#12859=DIRECTION ( 'NONE',  ( 1.734723475976842100E-16, -1.000000000000000000, 0.000000000000000000 ) ) ;
#12861=CARTESIAN_POINT ( 'NONE',  ( 134.4977709871204468, -7.448582144743035371, 8.000000000000007105 ) ) ;
#12871=CIRCLE ( 'NONE', #1054, 16.50000000000000355 ) ;
#12872=CARTESIAN_POINT ( 'NONE',  ( 153.1086002691896510, -2.071067811865468400, -4.999999999999989342 ) ) ;
#12874=CARTESIAN_POINT ( 'NONE',  ( 151.4136751345948539, 0.000000000000000000, -5.500000000000005329 ) ) ;
#12875=CARTESIAN_POINT ( 'NONE',  ( 135.6636751345948255, 0.000000000000000000, 5.500000000000005329 ) ) ;
#12879=DIRECTION ( 'NONE',  ( 1.000000000000000000, -0.000000000000000000, -0.000000000000000000 ) ) ;
#12881=VERTEX_POINT ( 'NONE', #25949 ) ;
#12882=CARTESIAN_POINT ( 'NONE',  ( 160.9687500000000000, -2.485281374238585972, 6.000000000000005329 ) ) ;
#12889=AXIS2_PLACEMENT_3D ( 'NONE', #21584, #24310, #24173 ) ;
#12890=ORIENTED_EDGE ( 'NONE', *, *, #20670, .F. ) ;
#12893=ADVANCED_FACE ( 'NONE', ( #9533 ), #22952, .T. ) ;
#12904=CARTESIAN_POINT ( 'NONE',  ( 0.8619745489090037127, -15.74670610583283903, -7.642883928913010827 ) ) ;
#12912=SURFACE_SIDE_STYLE ('',( #1036 ) ) ;
#12917=DIRECTION ( 'NONE',  ( 1.000000000000000000, 0.000000000000000000, 0.000000000000000000 ) ) ;
#12918=CARTESIAN_POINT ( 'NONE',  ( 135.0000000000000284, -6.982120021884474781, -8.500000000000007105 ) ) ;
#12919=EDGE_LOOP ( 'NONE', ( #17289, #29628, #27932, #22868 ) ) ;
#12929=VERTEX_POINT ( 'NONE', #5197 ) ;
#12930=CARTESIAN_POINT ( 'NONE',  ( 156.0000000000000284, 6.000000000000005329, 0.000000000000000000 ) ) ;
#12934=VERTEX_POINT ( 'NONE', #19649 ) ;
#12939=ORIENTED_EDGE ( 'NONE', *, *, #28996, .T. ) ;
#12943=CARTESIAN_POINT ( 'NONE',  ( 159.7528503973856857, -11.43509073697069311, -3.684568878343219112 ) ) ;
#12944=LINE ( 'NONE', #15400, #25585 ) ;
#12945=CARTESIAN_POINT ( 'NONE',  ( 0.07065350754911334241, -15.06982159471415805, -8.897710498417703562 ) ) ;
#12949=CARTESIAN_POINT ( 'NONE',  ( 135.0000000000001421, 3.980162674786793975, 4.050973044690350910 ) ) ;
#12951=DIRECTION ( 'NONE',  ( 1.000000000000000000, 1.734723475976824844E-16, -0.000000000000000000 ) ) ;
#12954=ORIENTED_EDGE ( 'NONE', *, *, #18715, .T. ) ;
#12956=CARTESIAN_POINT ( 'NONE',  ( 136.0000000000000284, -8.798545334315205579, 8.160000000000000142 ) ) ;
#12964=ADVANCED_FACE ( 'NONE', ( #17662 ), #26985, .T. ) ;
#12965=EDGE_CURVE ( 'NONE', #14623, #1710, #12378, .T. ) ;
#12968=CARTESIAN_POINT ( 'NONE',  ( 140.5828481527998974, -11.16569630559838444, 4.440052304731517019 ) ) ;
#12969=ORIENTED_EDGE ( 'NONE', *, *, #23559, .F. ) ;
#12971=AXIS2_PLACEMENT_3D ( 'NONE', #26978, #27137, #1176 ) ;
#12972=CONICAL_SURFACE ( 'NONE', #27650, 5.500000000000000000, 0.7853981633974369547 ) ;
#12973=CARTESIAN_POINT ( 'NONE',  ( 160.5832898866354981, -11.34230189387781884, 3.922211216774294851 ) ) ;
#12975=CARTESIAN_POINT ( 'NONE',  ( 136.4136751345948539, 0.000000000000000000, -5.500000000000005329 ) ) ;
#12980=CARTESIAN_POINT ( 'NONE',  ( 150.2663997308104058, -4.999999999999989342, -2.071067811865468400 ) ) ;
#12981=LINE ( 'NONE', #22316, #13888 ) ;
#12982=DIRECTION ( 'NONE',  ( 0.000000000000000000, 0.000000000000000000, 1.000000000000000000 ) ) ;
#12983=DIRECTION ( 'NONE',  ( 0.000000000000000000, 0.000000000000000000, -1.000000000000000000 ) ) ;
#12984=SURFACE_STYLE_FILL_AREA ( #12675 ) ;
#12986=FACE_OUTER_BOUND ( 'NONE', #6883, .T. ) ;
#12994=CARTESIAN_POINT ( 'NONE',  ( 148.1250000000000284, 0.000000000000000000, -6.000000000000005329 ) ) ;
#13000=CARTESIAN_POINT ( 'NONE',  ( 147.0937500000000284, 6.000000000000005329, 2.485281374238585972 ) ) ;
#13001=ORIENTED_EDGE ( 'NONE', *, *, #4031, .T. ) ;
#13009=( BOUNDED_SURFACE ( )  B_SPLINE_SURFACE ( 3, 2, ( 
 ( #10904, #10589, #17659 ),
 ( #19940, #29134, #1492 ),
 ( #13072, #22406, #29289 ),
 ( #8246, #26982, #5947 ),
 ( #1341, #15370, #10754 ),
 ( #8415, #17821, #3792 ),
 ( #7021, #6721, #18877 ),
 ( #4565, #23482, #2120 ),
 ( #4710, #25281, #13991 ),
 ( #28049, #21019, #2420 ) ),
 .UNSPECIFIED., .F., .F., .T. ) 
 B_SPLINE_SURFACE_WITH_KNOTS ( ( 4, 2, 2, 2, 4 ),
 ( 3, 3 ),
 ( 0.0003766318053149186927, 0.0009617798311713785311, 0.001546927857027838261, 0.002132075882884297991, 0.002717223908740757938 ),
 ( 0.000000000000000000, 1.000000000000000000 ),
 .UNSPECIFIED. ) 
 GEOMETRIC_REPRESENTATION_ITEM ( )  RATIONAL_B_SPLINE_SURFACE ( (
 ( 1.000000000000000000, 0.7071067811871951658, 1.000000000000000000),
 ( 1.000000000000000000, 0.7334558377629624148, 1.000000000000000000),
 ( 1.000000000000000000, 0.7720829478853132866, 1.000000000000000000),
 ( 1.000000000000000000, 0.8526052345356729401, 1.000000000000000000),
 ( 1.000000000000000000, 0.8923351120859769336, 1.000000000000000000),
 ( 1.000000000000000000, 0.9508075038259667933, 1.000000000000000000),
 ( 1.000000000000000000, 0.9705468812199546935, 1.000000000000000000),
 ( 1.000000000000000000, 0.9949883423647858383, 1.000000000000000000),
 ( 1.000000000000000000, 0.9999576422882877624, 1.000000000000000000),
 ( 1.000000000000000000, 1.000000000000000000, 1.000000000000000000) ) ) 
 REPRESENTATION_ITEM ( '' )  SURFACE ( )  );
#13024=( LENGTH_UNIT ( ) NAMED_UNIT ( * ) SI_UNIT ( .MILLI., .METRE. ) );
#13026=CARTESIAN_POINT ( 'NONE',  ( 155.3363248654052313, 0.000000000000000000, -5.500000000000005329 ) ) ;
#13027=CARTESIAN_POINT ( 'NONE',  ( 153.9523502691896510, 0.000000000000000000, 5.000000000000004441 ) ) ;
#13028=CARTESIAN_POINT ( 'NONE',  ( -0.5000000000000004441, -10.50000000000000888, -7.500000000000007105 ) ) ;
#13029=CARTESIAN_POINT ( 'NONE',  ( 152.0699251345948255, 2.278174593052229469, 5.499999999999796607 ) ) ;
#13030=CARTESIAN_POINT ( 'NONE',  ( 144.6488248654052029, -3.889087296526011706, -3.889087296526011706 ) ) ;
#13037=PLANE ( 'NONE',  #3269 ) ;
#13038=DIRECTION ( 'NONE',  ( 0.000000000000000000, 0.000000000000000000, -1.000000000000000000 ) ) ;
#13044=UNCERTAINTY_MEASURE_WITH_UNIT (LENGTH_MEASURE( 1.000000000000000082E-05 ), #10235, 'distance_accuracy_value', 'NONE');
#13051=DIRECTION ( 'NONE',  ( 0.000000000000000000, -1.000000000000000000, 0.000000000000000000 ) ) ;
#13052=CARTESIAN_POINT ( 'NONE',  ( 135.0000000000000284, -7.797609721147493289, 7.985501965054816687 ) ) ;
#13053=DIRECTION ( 'NONE',  ( 1.000000000000000000, 0.000000000000000000, -0.000000000000000000 ) ) ;
#13063=CARTESIAN_POINT ( 'NONE',  ( -0.06529312629391929856, -14.68416511718297990, 8.236104995426456910 ) ) ;
#13065=CARTESIAN_POINT ( 'NONE',  ( -0.5000000001309222730, -10.00000000000000888, 4.869076758059741827 ) ) ;
#13072=CARTESIAN_POINT ( 'NONE',  ( 135.4055088883162909, -8.802581727796308542, 8.024171615095424315 ) ) ;
#13079=ORIENTED_EDGE ( 'NONE', *, *, #3218, .F. ) ;
#13087=ORIENTED_EDGE ( 'NONE', *, *, #20453, .F. ) ;
#13088=CARTESIAN_POINT ( 'NONE',  ( 158.7187500000000000, 2.485281374238555774, -6.000000000000005329 ) ) ;
#13095=CARTESIAN_POINT ( 'NONE',  ( 159.5293203550124872, -11.10241815267761289, 4.553791194299030565 ) ) ;
#13096=DIRECTION ( 'NONE',  ( 1.000000000000000000, -0.000000000000000000, -0.000000000000000000 ) ) ;
#13097=ORIENTED_EDGE ( 'NONE', *, *, #5382, .T. ) ;
#13098=DIRECTION ( 'NONE',  ( 1.734723475976824844E-16, -1.000000000000000000, 0.000000000000000000 ) ) ;
#13099=CARTESIAN_POINT ( 'NONE',  ( 125.0000000000000568, -55.00000000000000711, -4.000000000000003553 ) ) ;
#13101=FACE_OUTER_BOUND ( 'NONE', #28358, .T. ) ;
#13104=CIRCLE ( 'NONE', #3210, 30.00000000000000355 ) ;
#13109=DIRECTION ( 'NONE',  ( 0.000000000000000000, 1.000000000000000000, -0.000000000000000000 ) ) ;
#13113=DIRECTION ( 'NONE',  ( -1.734723475976806897E-15, 0.000000000000000000, 1.000000000000000000 ) ) ;
#13115=EDGE_CURVE ( 'NONE', #8808, #1192, #12856, .T. ) ;
#13121=CARTESIAN_POINT ( 'NONE',  ( 140.0000000000000284, -11.45643923738959202, -5.000000000000004441 ) ) ;
#13125=CARTESIAN_POINT ( 'NONE',  ( 143.3437500000000284, -6.000000000000005329, -2.485281374238555774 ) ) ;
#13128=VECTOR ( 'NONE', #6651, 1000.000000000000000 ) ;
#13129=CARTESIAN_POINT ( 'NONE',  ( 136.8824251345948539, 5.500000000000012434, 2.278174593052012309 ) ) ;
#13134=CARTESIAN_POINT ( 'NONE',  ( 148.0163997308104058, 4.999999999999989342, 2.071067811865468400 ) ) ;
#13137=VECTOR ( 'NONE', #16196, 1000.000000000000000 ) ;
#13139=SURFACE_STYLE_USAGE ( .BOTH. , #29525 ) ;
#13144=AXIS2_PLACEMENT_3D ( 'NONE', #15616, #15458, #14975 ) ;
#13151=VERTEX_POINT ( 'NONE', #26302 ) ;
#13153=CARTESIAN_POINT ( 'NONE',  ( 146.6250000000000284, 0.000000000000000000, -6.000000000000005329 ) ) ;
#13154=CARTESIAN_POINT ( 'NONE',  ( 142.1324251345948539, -5.500000000000012434, -2.278174593052012309 ) ) ;
#13156=TOROIDAL_SURFACE ( 'NONE', #10679, 16.00000000000000000, 1.000000000000000000 ) ;
#13159=VECTOR ( 'NONE', #30257, 1000.000000000000000 ) ;
#13160=ORIENTED_EDGE ( 'NONE', *, *, #8303, .T. ) ;
#13161=CARTESIAN_POINT ( 'NONE',  ( 140.5312500000000284, -2.485281374238555774, -6.000000000000005329 ) ) ;
#13166=ORIENTED_EDGE ( 'NONE', *, *, #21634, .F. ) ;
#13173=VERTEX_POINT ( 'NONE', #5256 ) ;
#13176=CARTESIAN_POINT ( 'NONE',  ( 140.0000000000000284, -10.00000000000000888, -7.500000000000007105 ) ) ;
#13177=CARTESIAN_POINT ( 'NONE',  ( 135.0124395110251498, -7.358370994720393909, -8.428830671791343931 ) ) ;
#13179=VECTOR ( 'NONE', #11611, 1000.000000000000000 ) ;
#13180=EDGE_CURVE ( 'NONE', #8862, #13151, #3101, .T. ) ;
#13187=( NAMED_UNIT ( * ) PLANE_ANGLE_UNIT ( ) SI_UNIT ( $, .RADIAN. ) );
#13189=DIRECTION ( 'NONE',  ( -1.000000000000000000, -0.000000000000000000, -0.000000000000000000 ) ) ;
#13195=CARTESIAN_POINT ( 'NONE',  ( 162.0000000000000284, 6.000000000000005329, 0.000000000000000000 ) ) ;
#13196=CARTESIAN_POINT ( 'NONE',  ( -0.5000000000000004441, -14.50000000000001243, 7.500000000000007105 ) ) ;
#13199=LINE ( 'NONE', #20686, #25884 ) ;
#13200=ORIENTED_EDGE ( 'NONE', *, *, #27470, .F. ) ;
#13209=CARTESIAN_POINT ( 'NONE',  ( 0.8631338372297875372, -14.49999999999998579, -7.874007874011823560 ) ) ;
#13212=FILL_AREA_STYLE_COLOUR ( '', #140 ) ;
#13214=CARTESIAN_POINT ( 'NONE',  ( 146.3511751345948255, -3.889087296526011706, 3.889087296526011706 ) ) ;
#13220=CARTESIAN_POINT ( 'NONE',  ( 135.0000000000000284, 0.000000000000000000, 0.000000000000000000 ) ) ;
#13230=LINE ( 'NONE', #4109, #25379 ) ;
#13233=VERTEX_POINT ( 'NONE', #23092 ) ;
#13235=CARTESIAN_POINT ( 'NONE',  ( 154.3125000000000284, 4.242640687119298093, -4.242640687119298093 ) ) ;
#13236=EDGE_CURVE ( 'NONE', #18697, #15961, #23156, .T. ) ;
#13244=FACE_OUTER_BOUND ( 'NONE', #15929, .T. ) ;
#13248=DIRECTION ( 'NONE',  ( 0.000000000000000000, 0.000000000000000000, -1.000000000000000000 ) ) ;
#13249=EDGE_CURVE ( 'NONE', #7272, #14299, #15749, .T. ) ;
#13251=FACE_OUTER_BOUND ( 'NONE', #17956, .T. ) ;
#13252=CARTESIAN_POINT ( 'NONE',  ( -19.99999999999998224, -25.00000000000010658, 8.000000000000007105 ) ) ;
#13263=VECTOR ( 'NONE', #11542, 1000.000000000000000 ) ;
#13266=CARTESIAN_POINT ( 'NONE',  ( 140.3586002691896226, 2.071067811865468400, 4.999999999999989342 ) ) ;
#13271=CARTESIAN_POINT ( 'NONE',  ( 135.0000000000000284, 3.279024082124037065, -4.561124296770755038 ) ) ;
#13274=CARTESIAN_POINT ( 'NONE',  ( 159.3477600650482486, -12.04942537661511714, 3.940026486796909477 ) ) ;
#13275=CARTESIAN_POINT ( 'NONE',  ( 144.6562500000000568, -6.000000000000005329, 2.485281374238555774 ) ) ;
#13276=ADVANCED_FACE ( 'NONE', ( #29524 ), #13593, .T. ) ;
#13277=VERTEX_POINT ( 'NONE', #24909 ) ;
#13278=SURFACE_STYLE_FILL_AREA ( #3848 ) ;
#13280=AXIS2_PLACEMENT_3D ( 'NONE', #28705, #14918, #905 ) ;
#13284=CARTESIAN_POINT ( 'NONE',  ( -1.000000000000000888, 11.00000000000001066, -3.000000000000002665 ) ) ;
#13286=ADVANCED_FACE ( 'NONE', ( #8639 ), #18042, .T. ) ;
#13287=( GEOMETRIC_REPRESENTATION_CONTEXT ( 3 ) GLOBAL_UNCERTAINTY_ASSIGNED_CONTEXT ( ( #1452 ) ) GLOBAL_UNIT_ASSIGNED_CONTEXT ( ( #15146, #26475, #12555 ) ) REPRESENTATION_CONTEXT ( 'NONE', 'WORKASPACE' ) );
#13288=CARTESIAN_POINT ( 'NONE',  ( 147.1726497308104058, -5.000000000000004441, 0.000000000000000000 ) ) ;
#13300=CARTESIAN_POINT ( 'NONE',  ( 146.4375000000000284, -4.242640687119298093, -4.242640687119298093 ) ) ;
#13303=CIRCLE ( 'NONE', #22077, 1.000000000000000000 ) ;
#13306=AXIS2_PLACEMENT_3D ( 'NONE', #2071, #27845, #11472 ) ;
#13307=CARTESIAN_POINT ( 'NONE',  ( 141.1875000000000284, 4.242640687119269671, 4.242640687119298093 ) ) ;
#13310=ADVANCED_FACE ( 'NONE', ( #6485 ), #25359, .F. ) ;
#13311=ADVANCED_FACE ( 'NONE', ( #11441 ), #6638, .F. ) ;
#13318=DIRECTION ( 'NONE',  ( 1.000000000000000000, 0.000000000000000000, 0.000000000000000000 ) ) ;
#13329=FILL_AREA_STYLE_COLOUR ( '', #1217 ) ;
#13331=CIRCLE ( 'NONE', #25545, 0.5000000000000004441 ) ;
#13334=LINE ( 'NONE', #29715, #29488 ) ;
#13339=CARTESIAN_POINT ( 'NONE',  ( 155.5312500000000568, -2.485281374238555774, -6.000000000000005329 ) ) ;
#13346=VERTEX_POINT ( 'NONE', #7399 ) ;
#13349=VERTEX_POINT ( 'NONE', #4923 ) ;
#13351=CARTESIAN_POINT ( 'NONE',  ( -40.00000000000000000, -20.00000000000021316, 3.000000000000002665 ) ) ;
#13352=AXIS2_PLACEMENT_3D ( 'NONE', #6366, #1766, #6072 ) ;
#13353=LINE ( 'NONE', #13659, #16537 ) ;
#13359=MECHANICAL_DESIGN_GEOMETRIC_PRESENTATION_REPRESENTATION('',(#24109),#12373);
#13362=CARTESIAN_POINT ( 'NONE',  ( 145.9613248654052313, -5.500000000000005329, 0.000000000000000000 ) ) ;
#13367=ORIENTED_EDGE ( 'NONE', *, *, #7882, .T. ) ;
#13379=EDGE_CURVE ( 'NONE', #8771, #12929, #3244, .T. ) ;
#13382=CARTESIAN_POINT ( 'NONE',  ( 157.4062500000000284, 6.000000000000005329, -2.485281374238555774 ) ) ;
#13383=CIRCLE ( 'NONE', #9433, 1.000000000000000000 ) ;
#13391=CARTESIAN_POINT ( 'NONE',  ( 160.2454070297168300, -11.22992225825531065, 4.233399354748597965 ) ) ;
#13393=ORIENTED_EDGE ( 'NONE', *, *, #4064, .F. ) ;
#13395=CARTESIAN_POINT ( 'NONE',  ( 160.2350387298822909, -11.23134877322066849, -4.226361252505896893 ) ) ;
#13396=CARTESIAN_POINT ( 'NONE',  ( 140.1488248654052029, -3.889087296526011706, -3.889087296526011706 ) ) ;
#13402=CYLINDRICAL_SURFACE ( 'NONE', #15113, 9.999999999999996447 ) ;
#13407=EDGE_CURVE ( 'NONE', #3582, #5729, #8578, .T. ) ;
#13410=CARTESIAN_POINT ( 'NONE',  ( 139.1398502691896510, -3.535533905932752852, 3.535533905932725318 ) ) ;
#13415=CARTESIAN_POINT ( 'NONE',  ( 135.0000000000000284, 2.227160363700459556, -5.061403124386353980 ) ) ;
#13419=CARTESIAN_POINT ( 'NONE',  ( 159.8821365566051895, -12.37993144645533938, 3.487185471932420011 ) ) ;
#13420=CARTESIAN_POINT ( 'NONE',  ( 139.3125000000000284, 4.242640687119298093, -4.242640687119298093 ) ) ;
#13423=( LENGTH_UNIT ( ) NAMED_UNIT ( * ) SI_UNIT ( .MILLI., .METRE. ) );
#13429=AXIS2_PLACEMENT_3D ( 'NONE', #18601, #27322, #27459 ) ;
#13430=CARTESIAN_POINT ( 'NONE',  ( 149.8913997308104058, -2.071067811865468400, 4.999999999999989342 ) ) ;
#13433=DIRECTION ( 'NONE',  ( 0.000000000000000000, 0.000000000000000000, -1.000000000000000000 ) ) ;
#13434=SURFACE_SIDE_STYLE ('',( #18346 ) ) ;
#13436=CARTESIAN_POINT ( 'NONE',  ( 137.5386751345948255, -5.500000000000005329, 0.000000000000000000 ) ) ;
#13443=DIRECTION ( 'NONE',  ( 1.000000000000000000, 0.000000000000000000, 0.000000000000000000 ) ) ;
#13445=ORIENTED_EDGE ( 'NONE', *, *, #25187, .F. ) ;
#13447=CARTESIAN_POINT ( 'NONE',  ( 146.1562500000000568, -6.000000000000005329, 2.485281374238556218 ) ) ;
#13448=DIRECTION ( 'NONE',  ( 1.000000000000000000, 6.938893903907222067E-15, 0.000000000000000000 ) ) ;
#13451=ADVANCED_FACE ( 'NONE', ( #20936 ), #28121, .F. ) ;
#13452=AXIS2_PLACEMENT_3D ( 'NONE', #26427, #21699, #8137 ) ;
#13453=CARTESIAN_POINT ( 'NONE',  ( 136.8750000000000284, 0.000000000000000000, 6.000000000000005329 ) ) ;
#13455=COLOUR_RGB ( '', 0.31764706, 0.68627451, 0.89019608) ;
#13456=VERTEX_POINT ( 'NONE', #11744 ) ;
#13459=ORIENTED_EDGE ( 'NONE', *, *, #28782, .T. ) ;
#13466=B_SPLINE_CURVE_WITH_KNOTS ( 'NONE', 3,
 ( #26640, #22526, #17934, #10546, #19903, #29404, #27250, #19749, #24342, #24809 ),
 .UNSPECIFIED., .F., .F.,
 ( 4, 2, 2, 2, 4 ),
 ( 0.000000000000000000, 0.001275962895115241537, 0.002551925790230482639, 0.003827888685345722658, 0.005103851580460961809 ),
 .UNSPECIFIED. ) ;
#13473=CARTESIAN_POINT ( 'NONE',  ( 139.9451382466496057, -9.135892426262346433, -7.783435338407951321 ) ) ;
#13474=AXIS2_PLACEMENT_3D ( 'NONE', #23102, #30145, #23260 ) ;
#13475=DIRECTION ( 'NONE',  ( -1.000000000000000000, -1.734723475976843579E-16, 0.000000000000000000 ) ) ;
#13481=CARTESIAN_POINT ( 'NONE',  ( 149.7336002691896226, -4.999999999999989342, 2.071067811865468400 ) ) ;
#13484=CARTESIAN_POINT ( 'NONE',  ( 135.4369327280547566, -8.875721941249034685, -8.012675569329063663 ) ) ;
#13490=DIRECTION ( 'NONE',  ( 1.000000000000000000, 0.000000000000000000, 0.000000000000000000 ) ) ;
#13492=CARTESIAN_POINT ( 'NONE',  ( 155.8125000000000284, 4.242640687119298093, -4.242640687119298093 ) ) ;
#13502=ORIENTED_EDGE ( 'NONE', *, *, #6301, .T. ) ;
#13504=DIRECTION ( 'NONE',  ( -0.000000000000000000, -0.000000000000000000, -1.000000000000000000 ) ) ;
#13519=EDGE_CURVE ( 'NONE', #26206, #23261, #17092, .T. ) ;
#13521=CARTESIAN_POINT ( 'NONE',  ( 160.7961002691896510, 2.071067811865468400, -4.999999999999989342 ) ) ;
#13522=CARTESIAN_POINT ( 'NONE',  ( -0.04562205425673543369, -14.50000000000001243, 8.291335958003944739 ) ) ;
#13527=CARTESIAN_POINT ( 'NONE',  ( 116.0000000000000142, 6.735557395310442023E-16, 5.500000000000000000 ) ) ;
#13528=ORIENTED_EDGE ( 'NONE', *, *, #12480, .T. ) ;
#13529=FACE_OUTER_BOUND ( 'NONE', #5767, .T. ) ;
#13535=CARTESIAN_POINT ( 'NONE',  ( 157.8750000000000568, 0.000000000000000000, 6.000000000000005329 ) ) ;
#13540=ORIENTED_EDGE ( 'NONE', *, *, #23519, .T. ) ;
#13541=CARTESIAN_POINT ( 'NONE',  ( 156.9300748654052313, 2.278174593051842223, -5.500000000000182077 ) ) ;
#13544=CARTESIAN_POINT ( 'NONE',  ( 159.8766298123001093, -12.37305747749753415, 3.498085420967321113 ) ) ;
#13545=ORIENTED_EDGE ( 'NONE', *, *, #17310, .T. ) ;
#13547=FACE_OUTER_BOUND ( 'NONE', #2972, .T. ) ;
#13558=ADVANCED_FACE ( 'NONE', ( #8127 ), #9863, .F. ) ;
#13564=AXIS2_PLACEMENT_3D ( 'NONE', #22488, #29536, #17898 ) ;
#13566=FACE_OUTER_BOUND ( 'NONE', #6759, .T. ) ;
#13567=CARTESIAN_POINT ( 'NONE',  ( 137.2648502691896510, 3.535533905932725318, 3.535533905932752852 ) ) ;
#13568=VERTEX_POINT ( 'NONE', #24569 ) ;
#13570=CARTESIAN_POINT ( 'NONE',  ( -14.99999999999999289, -25.00000000000007816, 7.500000000000007105 ) ) ;
#13573=AXIS2_PLACEMENT_3D ( 'NONE', #29765, #11218, #6730 ) ;
#13576=VERTEX_POINT ( 'NONE', #16943 ) ;
#13578=CARTESIAN_POINT ( 'NONE',  ( 142.0312500000000284, -2.485281374238555774, -6.000000000000005329 ) ) ;
#13586=DIRECTION ( 'NONE',  ( 1.000000000000000000, -0.000000000000000000, -0.000000000000000000 ) ) ;
#13587=DIRECTION ( 'NONE',  ( -1.000000000000000000, 0.000000000000000000, 0.000000000000000000 ) ) ;
#13589=CARTESIAN_POINT ( 'NONE',  ( 144.0788997308104058, -4.999999999999989342, 2.071067811865468400 ) ) ;
#13593=CYLINDRICAL_SURFACE ( 'NONE', #15311, 12.00000000000000178 ) ;
#13597=ORIENTED_EDGE ( 'NONE', *, *, #28715, .T. ) ;
#13602=VERTEX_POINT ( 'NONE', #22441 ) ;
#13604=CARTESIAN_POINT ( 'NONE',  ( 147.8437500000000284, -6.000000000000005329, -2.485281374238556218 ) ) ;
#13607=CARTESIAN_POINT ( 'NONE',  ( 136.9687500000000000, -2.485281374238585972, 6.000000000000005329 ) ) ;
#13611=VERTEX_POINT ( 'NONE', #27022 ) ;
#13614=EDGE_CURVE ( 'NONE', #23117, #18461, #15060, .T. ) ;
#13619=CARTESIAN_POINT ( 'NONE',  ( 140.1146164139961456, -11.55730820707150919, -4.524920606409365220 ) ) ;
#13625=CARTESIAN_POINT ( 'NONE',  ( 140.1633619592320770, -9.008502785496828480, -7.928502883319133332 ) ) ;
#13630=VECTOR ( 'NONE', #6336, 1000.000000000000000 ) ;
#13631=VECTOR ( 'NONE', #6609, 1000.000000000000000 ) ;
#13635=LINE ( 'NONE', #13795, #30181 ) ;
#13636=AXIS2_PLACEMENT_3D ( 'NONE', #26583, #15097, #7699 ) ;
#13644=CARTESIAN_POINT ( 'NONE',  ( 153.5625000000000568, -4.242640687119298093, 4.242640687119298093 ) ) ;
#13649=CARTESIAN_POINT ( 'NONE',  ( -20.99999999999998224, -54.99999999999990763, 4.000000000000003553 ) ) ;
#13650=ORIENTED_EDGE ( 'NONE', *, *, #168, .F. ) ;
#13651=ORIENTED_EDGE ( 'NONE', *, *, #11537, .T. ) ;
#13655=EDGE_CURVE ( 'NONE', #1119, #1053, #15748, .T. ) ;
#13658=CARTESIAN_POINT ( 'NONE',  ( 140.0493945286584108, -8.932592928453178871, -8.013407610087551092 ) ) ;
#13659=CARTESIAN_POINT ( 'NONE',  ( -4.999999999999984013, -69.50000000000001421, -8.000000000000007105 ) ) ;
#13663=EDGE_CURVE ( 'NONE', #9581, #26206, #3905, .T. ) ;
#13666=CARTESIAN_POINT ( 'NONE',  ( 139.7940636821621752, -8.829150386088183922, 8.127229673620972150 ) ) ;
#13673=CARTESIAN_POINT ( 'NONE',  ( 158.3586002691896510, 2.071067811865468400, 4.999999999999989342 ) ) ;
#13674=CARTESIAN_POINT ( 'NONE',  ( 0.2071426722869369463, -15.61926834800564023, 7.893137763387031214 ) ) ;
#13675=ORIENTED_EDGE ( 'NONE', *, *, #14028, .F. ) ;
#13681=ORIENTED_EDGE ( 'NONE', *, *, #17566, .T. ) ;
#13685=ADVANCED_BREP_SHAPE_REPRESENTATION ( '', ( #13969, #18805 ), #19755 ) ;
#13692=CARTESIAN_POINT ( 'NONE',  ( 148.7812500000000284, 2.485281374238585972, 6.000000000000005329 ) ) ;
#13703=ORIENTED_EDGE ( 'NONE', *, *, #15885, .T. ) ;
#13704=CARTESIAN_POINT ( 'NONE',  ( -0.07769256095282929542, -15.23231281889968969, -7.500000000000007105 ) ) ;
#13707=FACE_OUTER_BOUND ( 'NONE', #10212, .T. ) ;
#13708=CARTESIAN_POINT ( 'NONE',  ( -40.00000000000000000, -20.00000000000021316, -3.000000000000002665 ) ) ;
#13713=CARTESIAN_POINT ( 'NONE',  ( -0.6927266194436478841, -9.614546761112784168, -4.200333198739684804 ) ) ;
#13719=CARTESIAN_POINT ( 'NONE',  ( 154.2113248654052313, 5.500000000000005329, 0.000000000000000000 ) ) ;
#13720=ORIENTED_EDGE ( 'NONE', *, *, #28341, .F. ) ;
#13724=CARTESIAN_POINT ( 'NONE',  ( 136.3273502691896510, -5.000000000000004441, 0.000000000000000000 ) ) ;
#13725=EDGE_LOOP ( 'NONE', ( #9885, #7850, #8342, #23154 ) ) ;
#13734=CARTESIAN_POINT ( 'NONE',  ( 140.8125000000000284, 4.242640687119298093, -4.242640687119298093 ) ) ;
#13738=FACE_OUTER_BOUND ( 'NONE', #17070, .T. ) ;
#13739=SURFACE_STYLE_FILL_AREA ( #30277 ) ;
#13743=CARTESIAN_POINT ( 'NONE',  ( 143.6101497308104058, 3.535533905932725318, 3.535533905932725318 ) ) ;
#13747=DIRECTION ( 'NONE',  ( 0.000000000000000000, -0.000000000000000000, 1.000000000000000000 ) ) ;
#13748=LINE ( 'NONE', #1874, #11135 ) ;
#13751=MECHANICAL_DESIGN_GEOMETRIC_PRESENTATION_REPRESENTATION('',(#924),#25958);
#13752=DIRECTION ( 'NONE',  ( 1.000000000000000000, -0.000000000000000000, -0.000000000000000000 ) ) ;
#13758=ORIENTED_EDGE ( 'NONE', *, *, #18744, .T. ) ;
#13760=CARTESIAN_POINT ( 'NONE',  ( 142.8750000000000284, 0.000000000000000000, 6.000000000000005329 ) ) ;
#13763=CARTESIAN_POINT ( 'NONE',  ( 138.6562500000000568, -6.000000000000005329, 2.485281374238555774 ) ) ;
#13765=ORIENTED_EDGE ( 'NONE', *, *, #10051, .T. ) ;
#13766=AXIS2_PLACEMENT_3D ( 'NONE', #17235, #10006, #1203 ) ;
#13768=EDGE_CURVE ( 'NONE', #13277, #2002, #7352, .T. ) ;
#13769=VECTOR ( 'NONE', #18838, 1000.000000000000000 ) ;
#13779=CARTESIAN_POINT ( 'NONE',  ( 154.5074251345949108, 2.278174593052074925, -5.499999999999950262 ) ) ;
#13780=DIRECTION ( 'NONE',  ( 0.000000000000000000, 0.000000000000000000, -1.000000000000000000 ) ) ;
#13784=CARTESIAN_POINT ( 'NONE',  ( 140.0000000000000284, -9.819569584722252387, -7.620286941409521120 ) ) ;
#13788=STYLED_ITEM ( 'NONE', ( #24968 ), #26910 ) ;
#13793=CARTESIAN_POINT ( 'NONE',  ( 150.5773502691896510, 5.000000000000004441, 0.000000000000000000 ) ) ;
#13795=CARTESIAN_POINT ( 'NONE',  ( -4.999999999999886313, -10.50000000000000888, 8.000000000000007105 ) ) ;
#13797=CARTESIAN_POINT ( 'NONE',  ( 157.5000000000000284, 6.000000000000005329, 0.000000000000000000 ) ) ;
#13803=CARTESIAN_POINT ( 'NONE',  ( 158.6250000000000568, 0.000000000000000000, -6.000000000000005329 ) ) ;
#13804=CARTESIAN_POINT ( 'NONE',  ( -20.99999999999998224, -25.00000000000010658, -4.000000000000003553 ) ) ;
#13816=MECHANICAL_DESIGN_GEOMETRIC_PRESENTATION_REPRESENTATION('',(#14778),#7398);
#13821=CIRCLE ( 'NONE', #519, 1.000000000000000000 ) ;
#13830=CARTESIAN_POINT ( 'NONE',  ( 158.9211002691896795, -4.999999999999989342, -2.071067811865468400 ) ) ;
#13831=CARTESIAN_POINT ( 'NONE',  ( -0.07769256095284231278, -15.23231281889969857, 7.499999999999993783 ) ) ;
#13835=EDGE_CURVE ( 'NONE', #20658, #28850, #26422, .T. ) ;
#13841=VERTEX_POINT ( 'NONE', #14740 ) ;
#13843=AXIS2_PLACEMENT_3D ( 'NONE', #30068, #20560, #17978 ) ;
#13844=ORIENTED_EDGE ( 'NONE', *, *, #17707, .F. ) ;
#13845=ADVANCED_FACE ( 'NONE', ( #5030 ), #16907, .T. ) ;
#13846=LINE ( 'NONE', #20875, #12578 ) ;
#13847=EDGE_CURVE ( 'NONE', #30104, #13277, #11825, .T. ) ;
#13848=( GEOMETRIC_REPRESENTATION_CONTEXT ( 3 ) GLOBAL_UNCERTAINTY_ASSIGNED_CONTEXT ( ( #7178 ) ) GLOBAL_UNIT_ASSIGNED_CONTEXT ( ( #3707, #5858, #12824 ) ) REPRESENTATION_CONTEXT ( 'NONE', 'WORKASPACE' ) );
#13850=CARTESIAN_POINT ( 'NONE',  ( 147.7500000000000284, -6.000000000000005329, 0.000000000000000000 ) ) ;
#13851=ORIENTED_EDGE ( 'NONE', *, *, #17911, .T. ) ;
#13858=CARTESIAN_POINT ( 'NONE',  ( 159.9741911234880547, -12.51693588432441651, 3.259847203776756075 ) ) ;
#13859=AXIS2_PLACEMENT_3D ( 'NONE', #15707, #22740, #17852 ) ;
#13861=SURFACE_STYLE_FILL_AREA ( #14695 ) ;
#13872=DIRECTION ( 'NONE',  ( 1.000000000000000000, 0.000000000000000000, -0.000000000000000000 ) ) ;
#13874=CARTESIAN_POINT ( 'NONE',  ( 135.0000000000000284, -8.132376923925228596, -7.784896983692046746 ) ) ;
#13879=CARTESIAN_POINT ( 'NONE',  ( 143.9136751345948539, 0.000000000000000000, -5.500000000000005329 ) ) ;
#13880=DIRECTION ( 'NONE',  ( 0.000000000000000000, -1.000000000000000000, 0.000000000000000000 ) ) ;
#13881=ORIENTED_EDGE ( 'NONE', *, *, #7847, .T. ) ;
#13886=( BOUNDED_CURVE ( )  B_SPLINE_CURVE ( 2, ( #21831, #2920, #2627, #910, #28562, #10308, #10159, #7530, #19673 ),
 .UNSPECIFIED., .F., .F. ) 
 B_SPLINE_CURVE_WITH_KNOTS ( ( 3, 2, 2, 2, 3 ),
 ( 0.7875000000000001998, 0.7937500000000005107, 0.8000000000000008216, 0.8062500000000010214, 0.8125000000000013323 ),
 .UNSPECIFIED. ) 
 CURVE ( )  GEOMETRIC_REPRESENTATION_ITEM ( )  RATIONAL_B_SPLINE_CURVE ( ( 0.9999999999999973355, 0.9238795325112894030, 1.000000000000000000, 0.9238795325112867385, 1.000000000000000000, 0.9238795325112867385, 1.000000000000000000, 0.9238795325112705292, 1.000000000000016209 ) ) 
 REPRESENTATION_ITEM ( '' )  );
#13888=VECTOR ( 'NONE', #1411, 1000.000000000000000 ) ;
#13894=CARTESIAN_POINT ( 'NONE',  ( 134.0625000000000284, -4.242640687119298093, 4.242640687119298093 ) ) ;
#13897=DIRECTION ( 'NONE',  ( 0.000000000000000000, 0.000000000000000000, -1.000000000000000000 ) ) ;
#13900=FILL_AREA_STYLE_COLOUR ( '', #24466 ) ;
#13902=CARTESIAN_POINT ( 'NONE',  ( 141.2663997308104058, -4.999999999999989342, -2.071067811865468400 ) ) ;
#13911=SURFACE_SIDE_STYLE ('',( #18649 ) ) ;
#13913=EDGE_CURVE ( 'NONE', #11180, #14866, #618, .T. ) ;
#13917=DIRECTION ( 'NONE',  ( 1.000000000000000000, -0.000000000000000000, -0.000000000000000000 ) ) ;
#13920=CARTESIAN_POINT ( 'NONE',  ( 138.2812500000000284, 2.485281374238585972, 6.000000000000005329 ) ) ;
#13922=LINE ( 'NONE', #14078, #13179 ) ;
#13923=CARTESIAN_POINT ( 'NONE',  ( 132.0937500000000568, 6.000000000000005329, 2.485281374238585972 ) ) ;
#13927=( BOUNDED_CURVE ( )  B_SPLINE_CURVE ( 2, ( #6335, #24614, #5870, #26906, #10677, #13154, #26749, #8656, #20333 ),
 .UNSPECIFIED., .F., .F. ) 
 B_SPLINE_CURVE_WITH_KNOTS ( ( 3, 2, 2, 2, 3 ),
 ( 0.3124999999999988898, 0.3187499999999990896, 0.3249999999999992895, 0.3312499999999996558, 0.3374999999999998557 ),
 .UNSPECIFIED. ) 
 CURVE ( )  GEOMETRIC_REPRESENTATION_ITEM ( )  RATIONAL_B_SPLINE_CURVE ( ( 1.000000000000013545, 0.9238795325112731938, 1.000000000000000000, 0.9238795325112867385, 1.000000000000000000, 0.9238795325112867385, 1.000000000000000000, 0.9238795325112887369, 0.9999999999999980016 ) ) 
 REPRESENTATION_ITEM ( '' )  );
#13932=CARTESIAN_POINT ( 'NONE',  ( 156.6636751345948255, 0.000000000000000000, 5.500000000000005329 ) ) ;
#13941=CARTESIAN_POINT ( 'NONE',  ( 140.0570668326235193, -8.936721004324988726, -8.008823461752308859 ) ) ;
#13944=CARTESIAN_POINT ( 'NONE',  ( -9.999999999999779732, -89.00000000000001421, -3.000000000000002665 ) ) ;
#13949=EDGE_CURVE ( 'NONE', #13349, #11180, #1709, .T. ) ;
#13950=AXIS2_PLACEMENT_3D ( 'NONE', #19688, #12801, #29028 ) ;
#13951=CARTESIAN_POINT ( 'NONE',  ( 139.8143194369503703, -9.354716546993699922, 7.895755101431983114 ) ) ;
#13952=CARTESIAN_POINT ( 'NONE',  ( 149.9211002691896226, -4.999999999999989342, -2.071067811865468400 ) ) ;
#13955=CARTESIAN_POINT ( 'NONE',  ( 159.3750000000000568, 0.000000000000000000, 6.000000000000005329 ) ) ;
#13960=SURFACE_SIDE_STYLE ('',( #25581 ) ) ;
#13962=CARTESIAN_POINT ( 'NONE',  ( 155.2500000000000284, -6.000000000000005329, 0.000000000000000000 ) ) ;
#13969=MANIFOLD_SOLID_BREP ( 'Cut-Sweep1', #28141 ) ;
#13972=LINE ( 'NONE', #28182, #11 ) ;
#13973=DIRECTION ( 'NONE',  ( 1.000000000000000000, 9.251858538542971828E-16, 0.000000000000000000 ) ) ;
#13975=( BOUNDED_CURVE ( )  B_SPLINE_CURVE ( 3, ( #21416, #2070, #19118, #14091 ),
 .UNSPECIFIED., .F., .F. ) 
 B_SPLINE_CURVE_WITH_KNOTS ( ( 4, 4 ),
 ( 1.570796326794896558, 3.141592653589793116 ),
 .UNSPECIFIED. ) 
 CURVE ( )  GEOMETRIC_REPRESENTATION_ITEM ( )  RATIONAL_B_SPLINE_CURVE ( ( 1.000000000000000000, 0.8047378541243649375, 0.8047378541243649375, 1.000000000000000000 ) ) 
 REPRESENTATION_ITEM ( '' )  );
#13978=CARTESIAN_POINT ( 'NONE',  ( 136.0000000000000284, -8.946933499675676416, 8.000000000000007105 ) ) ;
#13989=CARTESIAN_POINT ( 'NONE',  ( 161.0000000000000284, -12.64911064067353408, -3.000000000000002665 ) ) ;
#13990=CARTESIAN_POINT ( 'NONE',  ( 158.7336002691896510, -4.999999999999989342, 2.071067811865468400 ) ) ;
#13991=CARTESIAN_POINT ( 'NONE',  ( 134.9999999999997158, -7.147106270679951301, 8.399947834374497546 ) ) ;
#13997=CARTESIAN_POINT ( 'NONE',  ( 125.0000000000000568, -55.00000000000000711, -5.000000000000004441 ) ) ;
#13998=ORIENTED_EDGE ( 'NONE', *, *, #13115, .F. ) ;
#14004=CARTESIAN_POINT ( 'NONE',  ( 151.4062500000000000, 6.000000000000005329, -2.485281374238555774 ) ) ;
#14009=( LENGTH_UNIT ( ) NAMED_UNIT ( * ) SI_UNIT ( .MILLI., .METRE. ) );
#14015=CARTESIAN_POINT ( 'NONE',  ( 153.4761751345948255, 3.889087296526011706, 3.889087296526011706 ) ) ;
#14017=CARTESIAN_POINT ( 'NONE',  ( 157.7738248654052029, -3.889087296526011706, 3.889087296526011706 ) ) ;
#14022=( NAMED_UNIT ( * ) PLANE_ANGLE_UNIT ( ) SI_UNIT ( $, .RADIAN. ) );
#14023=STYLED_ITEM ( 'NONE', ( #29339 ), #2852 ) ;
#14024=DIRECTION ( 'NONE',  ( 0.000000000000000000, 0.000000000000000000, -1.000000000000000000 ) ) ;
#14028=EDGE_CURVE ( 'NONE', #28619, #16115, #10766, .T. ) ;
#14030=CARTESIAN_POINT ( 'NONE',  ( 154.3050748654052597, 5.500000000000012434, 2.278174593052012309 ) ) ;
#14033=FACE_OUTER_BOUND ( 'NONE', #2758, .T. ) ;
#14035=ORIENTED_EDGE ( 'NONE', *, *, #8584, .T. ) ;
#14038=CIRCLE ( 'NONE', #19411, 0.5000000000000004441 ) ;
#14040=FILL_AREA_STYLE_COLOUR ( '', #5740 ) ;
#14042=VERTEX_POINT ( 'NONE', #27278 ) ;
#14045=CARTESIAN_POINT ( 'NONE',  ( 135.0937500000000284, 6.000000000000005329, 2.485281374238585972 ) ) ;
#14048=FILL_AREA_STYLE_COLOUR ( '', #19666 ) ;
#14049=EDGE_CURVE ( 'NONE', #20809, #30356, #11767, .T. ) ;
#14051=DIRECTION ( 'NONE',  ( 0.000000000000000000, 0.000000000000000000, -1.000000000000000000 ) ) ;
#14054=CARTESIAN_POINT ( 'NONE',  ( 146.6101497308104058, 3.535533905932725318, 3.535533905932725318 ) ) ;
#14060=FACE_OUTER_BOUND ( 'NONE', #28515, .T. ) ;
#14067=( BOUNDED_CURVE ( )  B_SPLINE_CURVE ( 2, ( #17145, #26469, #1566 ),
 .UNSPECIFIED., .F., .F. ) 
 B_SPLINE_CURVE_WITH_KNOTS ( ( 3, 3 ),
 ( 0.8875000000000003997, 0.8903868608885109337 ),
 .UNSPECIFIED. ) 
 CURVE ( )  GEOMETRIC_REPRESENTATION_ITEM ( )  RATIONAL_B_SPLINE_CURVE ( ( 0.9999999999999945599, 0.9648401279346661141, 0.9621607869126811430 ) ) 
 REPRESENTATION_ITEM ( '' )  );
#14069=ORIENTED_EDGE ( 'NONE', *, *, #14398, .F. ) ;
#14075=CARTESIAN_POINT ( 'NONE',  ( 142.3125000000000284, 4.242640687119298093, -4.242640687119298093 ) ) ;
#14078=CARTESIAN_POINT ( 'NONE',  ( -40.00000000000000000, -20.00000000000021316, 4.000000000000003553 ) ) ;
#14079=CARTESIAN_POINT ( 'NONE',  ( 135.4687500000000853, -2.485281374238585972, 6.000000000000005329 ) ) ;
#14083=ORIENTED_EDGE ( 'NONE', *, *, #25628, .T. ) ;
#14091=CARTESIAN_POINT ( 'NONE',  ( -0.5000000000000004441, -10.00000000000000888, -5.000000000000004441 ) ) ;
#14093=CARTESIAN_POINT ( 'NONE',  ( 161.0000000000000284, 0.000000000000000000, 0.000000000000000000 ) ) ;
#14098=CARTESIAN_POINT ( 'NONE',  ( 140.0000000000000284, -9.600000000000010303, -7.200000000000006395 ) ) ;
#14105=SURFACE_SIDE_STYLE ('',( #25724 ) ) ;
#14108=( GEOMETRIC_REPRESENTATION_CONTEXT ( 3 ) GLOBAL_UNCERTAINTY_ASSIGNED_CONTEXT ( ( #25912 ) ) GLOBAL_UNIT_ASSIGNED_CONTEXT ( ( #22010, #29359, #24298 ) ) REPRESENTATION_CONTEXT ( 'NONE', 'WORKASPACE' ) );
#14109=CARTESIAN_POINT ( 'NONE',  ( 155.4375000000000284, -4.242640687119298093, -4.242640687119298093 ) ) ;
#14115=CARTESIAN_POINT ( 'NONE',  ( 148.5937500000000284, 6.000000000000005329, 2.485281374238585972 ) ) ;
#14120=ORIENTED_EDGE ( 'NONE', *, *, #23526, .T. ) ;
#14121=ORIENTED_EDGE ( 'NONE', *, *, #10064, .F. ) ;
#14124=EDGE_CURVE ( 'NONE', #12257, #20028, #27509, .T. ) ;
#14126=DIRECTION ( 'NONE',  ( 1.000000000000000000, 0.000000000000000000, -0.000000000000000000 ) ) ;
#14127=CARTESIAN_POINT ( 'NONE',  ( 158.6101497308104058, 3.535533905932725318, 3.535533905932725318 ) ) ;
#14140=DIRECTION ( 'NONE',  ( 0.000000000000000000, 1.000000000000000000, 0.000000000000000000 ) ) ;
#14142=CARTESIAN_POINT ( 'NONE',  ( 159.7648502691896510, 3.535533905932725318, 3.535533905932752852 ) ) ;
#14143=CARTESIAN_POINT ( 'NONE',  ( 0.8056953124617616258, -15.44741955337846306, 8.223657085175583248 ) ) ;
#14152=( GEOMETRIC_REPRESENTATION_CONTEXT ( 3 ) GLOBAL_UNCERTAINTY_ASSIGNED_CONTEXT ( ( #23887 ) ) GLOBAL_UNIT_ASSIGNED_CONTEXT ( ( #3816, #23042, #11229 ) ) REPRESENTATION_CONTEXT ( 'NONE', 'WORKASPACE' ) );
#14156=CARTESIAN_POINT ( 'NONE',  ( 148.3125000000000284, 4.242640687119298093, -4.242640687119298093 ) ) ;
#14162=ORIENTED_EDGE ( 'NONE', *, *, #20383, .F. ) ;
#14163=( NAMED_UNIT ( * ) PLANE_ANGLE_UNIT ( ) SI_UNIT ( $, .RADIAN. ) );
#14166=SURFACE_STYLE_USAGE ( .BOTH. , #4737 ) ;
#14167=CARTESIAN_POINT ( 'NONE',  ( 0.1950468348593054624, -15.42105542096816073, -8.274702966242770685 ) ) ;
#14173=CARTESIAN_POINT ( 'NONE',  ( -0.5043617743979594836, -9.495638225602176519, -4.110987936241992102 ) ) ;
#14175=AXIS2_PLACEMENT_3D ( 'NONE', #28451, #7424, #16832 ) ;
#14178=CARTESIAN_POINT ( 'NONE',  ( 135.0976013656030261, -7.965572835763115478, -8.241760388316306418 ) ) ;
#14182=CARTESIAN_POINT ( 'NONE',  ( -0.04479393756897805806, -15.28421419621745692, -7.194883460697197641 ) ) ;
#14183=LINE ( 'NONE', #6761, #13159 ) ;
#14192=ORIENTED_EDGE ( 'NONE', *, *, #11786, .F. ) ;
#14194=CARTESIAN_POINT ( 'NONE',  ( 135.0000000000000284, 6.000000000000005329, 0.000000000000000000 ) ) ;
#14199=FILL_AREA_STYLE ('',( #7081 ) ) ;
#14202=CARTESIAN_POINT ( 'NONE',  ( 144.2663997308104058, -4.999999999999989342, -2.071067811865468400 ) ) ;
#14203=CARTESIAN_POINT ( 'NONE',  ( 135.0000000000000284, 0.000000000000000000, 0.000000000000000000 ) ) ;
#14204=CARTESIAN_POINT ( 'NONE',  ( 0.000000000000000000, -9.500000000000008882, 8.000000000000007105 ) ) ;
#14209=DIRECTION ( 'NONE',  ( -0.000000000000000000, -0.000000000000000000, -1.000000000000000000 ) ) ;
#14215=LINE ( 'NONE', #6948, #17035 ) ;
#14218=CARTESIAN_POINT ( 'NONE',  ( 140.3437500000000284, -6.000000000000005329, -2.485281374238556218 ) ) ;
#14220=EDGE_CURVE ( 'NONE', #3951, #3318, #18039, .T. ) ;
#14222=CARTESIAN_POINT ( 'NONE',  ( 142.6011751345948539, 3.889087296526011706, -3.889087296526011706 ) ) ;
#14223=CARTESIAN_POINT ( 'NONE',  ( 161.2351497308104058, 3.535533905932725318, -3.535533905932725318 ) ) ;
#14226=ADVANCED_FACE ( 'NONE', ( #23255 ), #14502, .F. ) ;
#14228=EDGE_CURVE ( 'NONE', #23810, #10268, #23549, .T. ) ;
#14234=CARTESIAN_POINT ( 'NONE',  ( 140.0000000000000284, -8.500000000000007105, 8.000000000000007105 ) ) ;
#14249=CARTESIAN_POINT ( 'NONE',  ( 143.4523502691896510, 0.000000000000000000, 5.000000000000004441 ) ) ;
#14250=DIRECTION ( 'NONE',  ( 0.000000000000000000, 1.000000000000000000, -0.000000000000000000 ) ) ;
#14251=CARTESIAN_POINT ( 'NONE',  ( 159.8437500000000284, -6.000000000000005329, -2.485281374238556218 ) ) ;
#14253=DIRECTION ( 'NONE',  ( 1.000000000000000000, -0.000000000000000000, -0.000000000000000000 ) ) ;
#14259=ORIENTED_EDGE ( 'NONE', *, *, #3779, .T. ) ;
#14261=CARTESIAN_POINT ( 'NONE',  ( 152.1562500000000284, -6.000000000000005329, 2.485281374238555774 ) ) ;
#14262=COLOUR_RGB ( '', 0.72549020, 0.75294118, 0.79215686) ;
#14270=ORIENTED_EDGE ( 'NONE', *, *, #2285, .T. ) ;
#14271=CARTESIAN_POINT ( 'NONE',  ( 157.8601497308104058, -3.535533905932725318, -3.535533905932725318 ) ) ;
#14272=CARTESIAN_POINT ( 'NONE',  ( 159.2738248654052029, -3.889087296526011706, 3.889087296526011706 ) ) ;
#14273=AXIS2_PLACEMENT_3D ( 'NONE', #838, #4205, #20210 ) ;
#14274=CARTESIAN_POINT ( 'NONE',  ( 135.8007686613932208, -8.946933464891957399, 7.999999999999145572 ) ) ;
#14280=FILL_AREA_STYLE_COLOUR ( '', #13455 ) ;
#14284=( BOUNDED_SURFACE ( )  B_SPLINE_SURFACE ( 3, 2, ( 
 ( #30016, #14098, #4519 ),
 ( #20821, #23287, #13784 ),
 ( #28002, #4665, #16244 ),
 ( #13625, #13473, #20505 ),
 ( #13941, #16092, #30169 ),
 ( #9133, #2228, #2377 ),
 ( #6819, #21122, #60 ),
 ( #6356, #15790, #1757 ) ),
 .UNSPECIFIED., .F., .F., .F. ) 
 B_SPLINE_SURFACE_WITH_KNOTS ( ( 4, 2, 2, 4 ),
 ( 3, 3 ),
 ( 0.0005074624230801699385, 0.001406250641872334528, 0.001855644751268416878, 0.002305038860664499010 ),
 ( 0.000000000000000000, 1.000000000000000000 ),
 .UNSPECIFIED. ) 
 GEOMETRIC_REPRESENTATION_ITEM ( )  RATIONAL_B_SPLINE_SURFACE ( (
 ( 1.000000000000000000, 0.7071067811865475727, 1.000000000000000000),
 ( 1.000000000000000000, 0.7582538634876517802, 1.000000000000000000),
 ( 1.000000000000000000, 0.8074746405292959617, 1.000000000000000000),
 ( 1.000000000000000000, 0.8664425519722945834, 1.000000000000000000),
 ( 1.000000000000000000, 0.8838341264643537754, 1.000000000000000000),
 ( 1.000000000000000000, 0.9091211823109212053, 1.000000000000000000),
 ( 1.000000000000000000, 0.9165811874549500970, 1.000000000000000000),
 ( 1.000000000000000000, 0.9165151389911680990, 1.000000000000000000) ) ) 
 REPRESENTATION_ITEM ( '' )  SURFACE ( )  );
#14285=CARTESIAN_POINT ( 'NONE',  ( 156.2961002691897079, 2.071067811865468400, -4.999999999999989342 ) ) ;
#14288=UNCERTAINTY_MEASURE_WITH_UNIT (LENGTH_MEASURE( 1.000000000000000082E-05 ), #29826, 'distance_accuracy_value', 'NONE');
#14290=CARTESIAN_POINT ( 'NONE',  ( 140.0000000000000284, 0.000000000000000000, 0.000000000000000000 ) ) ;
#14291=EDGE_CURVE ( 'NONE', #25175, #3090, #22511, .T. ) ;
#14293=CARTESIAN_POINT ( 'NONE',  ( 153.0863248654052313, 0.000000000000000000, 5.500000000000005329 ) ) ;
#14299=VERTEX_POINT ( 'NONE', #23402 ) ;
#14302=CARTESIAN_POINT ( 'NONE',  ( 152.6250000000000284, 0.000000000000000000, -6.000000000000005329 ) ) ;
#14307=ORIENTED_EDGE ( 'NONE', *, *, #15085, .F. ) ;
#14310=PRESENTATION_STYLE_ASSIGNMENT (( #14166 ) ) ;
#14311=ORIENTED_EDGE ( 'NONE', *, *, #1432, .T. ) ;
#14319=CIRCLE ( 'NONE', #2496, 13.00000000000000178 ) ;
#14320=CARTESIAN_POINT ( 'NONE',  ( 159.2599382550154985, -11.07692307692306777, -4.615384615384606093 ) ) ;
#14323=CARTESIAN_POINT ( 'NONE',  ( 135.0000000000000568, -8.453200966450170384, -7.964396152078529134 ) ) ;
#14328=CARTESIAN_POINT ( 'NONE',  ( -0.07769256095283699759, -15.23231281889969679, -7.500000000000007105 ) ) ;
#14331=ADVANCED_FACE ( 'NONE', ( #9410 ), #9717, .F. ) ;
#14336=CARTESIAN_POINT ( 'NONE',  ( 156.7574251345948539, -2.278174593051826236, 5.500000000000198064 ) ) ;
#14339=CARTESIAN_POINT ( 'NONE',  ( 137.8125000000000284, 4.242640687119298093, -4.242640687119298093 ) ) ;
#14340=AXIS2_PLACEMENT_3D ( 'NONE', #27505, #20006, #1567 ) ;
#14343=SURFACE_SIDE_STYLE ('',( #4914 ) ) ;
#14349=CARTESIAN_POINT ( 'NONE',  ( 137.5163997308104058, 4.999999999999989342, 2.071067811865468400 ) ) ;
#14352=VECTOR ( 'NONE', #14468, 1000.000000000000000 ) ;
#14354=CARTESIAN_POINT ( 'NONE',  ( 156.1011751345948255, 3.889087296526011706, -3.889087296526011706 ) ) ;
#14358=STYLED_ITEM ( 'NONE', ( #14892 ), #3422 ) ;
#14359=( NAMED_UNIT ( * ) PLANE_ANGLE_UNIT ( ) SI_UNIT ( $, .RADIAN. ) );
#14360=( NAMED_UNIT ( * ) SI_UNIT ( $, .STERADIAN. ) SOLID_ANGLE_UNIT ( ) );
#14361=ORIENTED_EDGE ( 'NONE', *, *, #1090, .F. ) ;
#14366=ORIENTED_EDGE ( 'NONE', *, *, #19654, .T. ) ;
#14368=CARTESIAN_POINT ( 'NONE',  ( 141.9375000000000284, -4.242640687119298093, -4.242640687119298093 ) ) ;
#14370=CARTESIAN_POINT ( 'NONE',  ( 138.5550748654052313, -5.500000000000012434, -2.278174593052012309 ) ) ;
#14372=CARTESIAN_POINT ( 'NONE',  ( 161.1413997308104058, 2.071067811865468400, -4.999999999999989342 ) ) ;
#14376=ORIENTED_EDGE ( 'NONE', *, *, #28341, .T. ) ;
#14380=CARTESIAN_POINT ( 'NONE',  ( 135.0000000000000284, 0.000000000000000000, 0.000000000000000000 ) ) ;
#14384=DIRECTION ( 'NONE',  ( 0.000000000000000000, 0.000000000000000000, 1.000000000000000000 ) ) ;
#14388=FACE_OUTER_BOUND ( 'NONE', #15010, .T. ) ;
#14398=EDGE_CURVE ( 'NONE', #3651, #10998, #1930, .T. ) ;
#14402=CARTESIAN_POINT ( 'NONE',  ( 145.6086002691897079, -2.071067811865468400, -4.999999999999989342 ) ) ;
#14404=CARTESIAN_POINT ( 'NONE',  ( 159.5625000000000284, -4.242640687119298093, 4.242640687119298093 ) ) ;
#14411=CARTESIAN_POINT ( 'NONE',  ( 149.1562500000000284, -6.000000000000005329, 2.485281374238555774 ) ) ;
#14419=CARTESIAN_POINT ( 'NONE',  ( 153.6413997308104342, 2.071067811865468400, -4.999999999999989342 ) ) ;
#14420=EDGE_CURVE ( 'NONE', #12934, #22336, #29827, .T. ) ;
#14423=CARTESIAN_POINT ( 'NONE',  ( 135.6059727065548941, -8.864963804575562989, 8.000000000000007105 ) ) ;
#14431=CARTESIAN_POINT ( 'NONE',  ( 142.4925748654052313, 2.278174593052074925, 5.499999999999950262 ) ) ;
#14435=CARTESIAN_POINT ( 'NONE',  ( 156.9523502691896510, 0.000000000000000000, 5.000000000000004441 ) ) ;
#14436=CARTESIAN_POINT ( 'NONE',  ( 141.6636751345948255, 0.000000000000000000, 5.500000000000005329 ) ) ;
#14442=ORIENTED_EDGE ( 'NONE', *, *, #7435, .F. ) ;
#14445=AXIS2_PLACEMENT_3D ( 'NONE', #28194, #25277, #23910 ) ;
#14446=CARTESIAN_POINT ( 'NONE',  ( 146.0625000000000284, -4.242640687119298093, 4.242640687119298093 ) ) ;
#14451=CARTESIAN_POINT ( 'NONE',  ( 158.4300748654052313, 2.278174593051857766, -5.500000000000166978 ) ) ;
#14454=ADVANCED_FACE ( 'NONE', ( #5375 ), #15082, .F. ) ;
#14455=EDGE_LOOP ( 'NONE', ( #3722, #26999, #14916, #24475 ) ) ;
#14456=CARTESIAN_POINT ( 'NONE',  ( 0.2071745301884423129, -15.61907693555130905, -7.893511971080271472 ) ) ;
#14463=CARTESIAN_POINT ( 'NONE',  ( 15.00000000000000000, 0.000000000000000000, 0.000000000000000000 ) ) ;
#14465=CARTESIAN_POINT ( 'NONE',  ( 116.0000000000000142, 6.735557395310442023E-16, 5.500000000000000000 ) ) ;
#14466=SURFACE_STYLE_USAGE ( .BOTH. , #289 ) ;
#14468=DIRECTION ( 'NONE',  ( -1.000000000000000000, 0.000000000000000000, 0.000000000000000000 ) ) ;
#14471=ORIENTED_EDGE ( 'NONE', *, *, #1400, .T. ) ;
#14481=EDGE_LOOP ( 'NONE', ( #2464, #27267, #23750, #22037 ) ) ;
#14486=CARTESIAN_POINT ( 'NONE',  ( 134.6398502691896510, -3.535533905932752852, 3.535533905932725318 ) ) ;
#14497=CARTESIAN_POINT ( 'NONE',  ( 140.5163997308104342, 4.999999999999989342, 2.071067811865468400 ) ) ;
#14498=LINE ( 'NONE', #22237, #24133 ) ;
#14502=CYLINDRICAL_SURFACE ( 'NONE', #18598, 0.5000000000000000000 ) ;
#14511=CARTESIAN_POINT ( 'NONE',  ( 133.7812500000000284, 2.485281374238585972, 6.000000000000005329 ) ) ;
#14513=ADVANCED_FACE ( 'NONE', ( #1534 ), #15720, .F. ) ;
#14515=ORIENTED_EDGE ( 'NONE', *, *, #24632, .T. ) ;
#14516=AXIS2_PLACEMENT_3D ( 'NONE', #8685, #23292, #25099 ) ;
#14519=CIRCLE ( 'NONE', #9584, 17.50000000000000355 ) ;
#14522=CARTESIAN_POINT ( 'NONE',  ( 160.0000000000000568, -12.58734212865233459, -3.130219457110984926 ) ) ;
#14529=CARTESIAN_POINT ( 'NONE',  ( 139.9468100150023702, -9.635049468574379716, 7.732362477259529854 ) ) ;
#14532=CARTESIAN_POINT ( 'NONE',  ( 144.9300748654052029, 2.278174593051733421, -5.500000000000292211 ) ) ;
#14535=CARTESIAN_POINT ( 'NONE',  ( 144.0148502691896510, -3.535533905932725318, -3.535533905932725318 ) ) ;
#14537=CARTESIAN_POINT ( 'NONE',  ( 150.7500000000000284, -6.000000000000005329, 0.000000000000000000 ) ) ;
#14540=COLOUR_RGB ( '', 0.31764706, 0.68627451, 0.89019608) ;
#14542=CARTESIAN_POINT ( 'NONE',  ( 116.0000000000000142, 0.000000000000000000, 0.000000000000000000 ) ) ;
#14544=CARTESIAN_POINT ( 'NONE',  ( 150.9375000000000284, -4.242640687119298093, -4.242640687119298093 ) ) ;
#14563=DIRECTION ( 'NONE',  ( 0.000000000000000000, 1.000000000000000000, 0.000000000000000000 ) ) ;
#14566=CARTESIAN_POINT ( 'NONE',  ( 156.2023502691896510, 0.000000000000000000, -5.000000000000004441 ) ) ;
#14576=EDGE_CURVE ( 'NONE', #7022, #28218, #5039, .T. ) ;
#14578=CARTESIAN_POINT ( 'NONE',  ( 146.4375000000000284, -4.242640687119298093, -4.242640687119298093 ) ) ;
#14580=( GEOMETRIC_REPRESENTATION_CONTEXT ( 3 ) GLOBAL_UNCERTAINTY_ASSIGNED_CONTEXT ( ( #14685 ) ) GLOBAL_UNIT_ASSIGNED_CONTEXT ( ( #5563, #5414, #24020 ) ) REPRESENTATION_CONTEXT ( 'NONE', 'WORKASPACE' ) );
#14584=UNCERTAINTY_MEASURE_WITH_UNIT (LENGTH_MEASURE( 1.000000000000000082E-05 ), #913, 'distance_accuracy_value', 'NONE');
#14589=AXIS2_PLACEMENT_3D ( 'NONE', #6472, #29512, #13897 ) ;
#14590=CARTESIAN_POINT ( 'NONE',  ( 0.000000000000000000, -9.500000000000008882, 5.000000000000004441 ) ) ;
#14594=FACE_OUTER_BOUND ( 'NONE', #8060, .T. ) ;
#14599=DIRECTION ( 'NONE',  ( 1.000000000000000000, -0.000000000000000000, -0.000000000000000000 ) ) ;
#14604=DIRECTION ( 'NONE',  ( 1.000000000000000000, 0.000000000000000000, 0.000000000000000000 ) ) ;
#14613=EDGE_CURVE ( 'NONE', #9799, #452, #10773, .T. ) ;
#14615=CARTESIAN_POINT ( 'NONE',  ( 156.9449251345948539, -5.500000000000012434, 2.278174593052012309 ) ) ;
#14617=ADVANCED_FACE ( 'NONE', ( #2738 ), #28832, .T. ) ;
#14620=DIRECTION ( 'NONE',  ( 1.000000000000000000, 0.000000000000000000, 0.000000000000000000 ) ) ;
#14621=CARTESIAN_POINT ( 'NONE',  ( 161.7187500000000000, 2.485281374238555774, -6.000000000000005329 ) ) ;
#14623=VERTEX_POINT ( 'NONE', #7213 ) ;
#14625=DIRECTION ( 'NONE',  ( 1.000000000000000000, 1.734723475976843579E-16, 0.000000000000000000 ) ) ;
#14632=DIRECTION ( 'NONE',  ( 0.000000000000000000, -1.000000000000000000, -0.000000000000000000 ) ) ;
#14633=CARTESIAN_POINT ( 'NONE',  ( 135.4538997308104058, -2.071067811865468400, -4.999999999999989342 ) ) ;
#14637=CARTESIAN_POINT ( 'NONE',  ( 161.0000000000000284, 0.000000000000000000, 0.000000000000000000 ) ) ;
#14644=VERTEX_POINT ( 'NONE', #21802 ) ;
#14646=CARTESIAN_POINT ( 'NONE',  ( 136.7812500000000568, 2.485281374238585972, 6.000000000000005329 ) ) ;
#14649=EDGE_CURVE ( 'NONE', #2895, #8039, #11774, .T. ) ;
#14650=PRESENTATION_STYLE_ASSIGNMENT (( #26722 ) ) ;
#14657=LINE ( 'NONE', #21712, #26784 ) ;
#14665=LINE ( 'NONE', #17124, #22968 ) ;
#14668=CARTESIAN_POINT ( 'NONE',  ( -14.99999999999999289, -25.00000000000007816, -7.500000000000007105 ) ) ;
#14670=CARTESIAN_POINT ( 'NONE',  ( 116.0000000000000142, 0.000000000000000000, -5.500000000000000000 ) ) ;
#14671=CARTESIAN_POINT ( 'NONE',  ( 146.7113248654052313, 5.500000000000005329, 0.000000000000000000 ) ) ;
#14676=CARTESIAN_POINT ( 'NONE',  ( 145.5148502691896510, -3.535533905932725318, -3.535533905932725318 ) ) ;
#14677=CARTESIAN_POINT ( 'NONE',  ( 150.1875000000000284, 4.242640687119269671, 4.242640687119298093 ) ) ;
#14684=CARTESIAN_POINT ( 'NONE',  ( 151.2187500000000284, 2.485281374238555774, -6.000000000000005329 ) ) ;
#14685=UNCERTAINTY_MEASURE_WITH_UNIT (LENGTH_MEASURE( 1.000000000000000082E-05 ), #5563, 'distance_accuracy_value', 'NONE');
#14689=ORIENTED_EDGE ( 'NONE', *, *, #88, .T. ) ;
#14691=ORIENTED_EDGE ( 'NONE', *, *, #9815, .T. ) ;
#14693=ORIENTED_EDGE ( 'NONE', *, *, #16069, .T. ) ;
#14695=FILL_AREA_STYLE ('',( #26335 ) ) ;
#14699=CARTESIAN_POINT ( 'NONE',  ( 160.9878691019586654, 3.688149050334593504, 4.090025542717429907 ) ) ;
#14707=FACE_OUTER_BOUND ( 'NONE', #22114, .T. ) ;
#14709=AXIS2_PLACEMENT_3D ( 'NONE', #15070, #22127, #2768 ) ;
#14711=CARTESIAN_POINT ( 'NONE',  ( 157.8898502691896510, 3.535533905932725318, -3.535533905932725318 ) ) ;
#14716=CARTESIAN_POINT ( 'NONE',  ( 145.4136751345948539, 0.000000000000000000, -5.500000000000005329 ) ) ;
#14718=CARTESIAN_POINT ( 'NONE',  ( 0.7669223171414829565, -14.69693845669908860, -7.500000000000007105 ) ) ;
#14719=EDGE_CURVE ( 'NONE', #4838, #9581, #21589, .T. ) ;
#14720=ORIENTED_EDGE ( 'NONE', *, *, #23147, .F. ) ;
#14728=ORIENTED_EDGE ( 'NONE', *, *, #14576, .F. ) ;
#14730=MECHANICAL_DESIGN_GEOMETRIC_PRESENTATION_REPRESENTATION('',(#1477),#13287);
#14732=DIRECTION ( 'NONE',  ( 0.000000000000000000, 0.000000000000000000, 1.000000000000000000 ) ) ;
#14733=CARTESIAN_POINT ( 'NONE',  ( 131.7976497308104058, 0.000000000000000000, 5.000000000000004441 ) ) ;
#14735=ORIENTED_EDGE ( 'NONE', *, *, #15046, .T. ) ;
#14736=CARTESIAN_POINT ( 'NONE',  ( 0.8346751507289797978, -15.41336419498994026, -8.287310550375268647 ) ) ;
#14737=DIRECTION ( 'NONE',  ( 1.000000000000000000, -0.000000000000000000, -0.000000000000000000 ) ) ;
#14740=CARTESIAN_POINT ( 'NONE',  ( -4.999999999999886313, -10.50000000000000888, 8.000000000000007105 ) ) ;
#14744=EDGE_CURVE ( 'NONE', #19344, #11694, #21600, .T. ) ;
#14746=DIRECTION ( 'NONE',  ( 0.000000000000000000, 1.000000000000000000, -0.000000000000000000 ) ) ;
#14748=DIRECTION ( 'NONE',  ( 0.000000000000000000, 0.000000000000000000, -1.000000000000000000 ) ) ;
#14753=AXIS2_PLACEMENT_3D ( 'NONE', #14767, #12331, #14625 ) ;
#14756=COLOUR_RGB ( '', 0.09019608, 0.27058824, 0.51372549) ;
#14758=CARTESIAN_POINT ( 'NONE',  ( 0.000000000000000000, 0.000000000000000000, -16.50000000000000355 ) ) ;
#14760=( LENGTH_UNIT ( ) NAMED_UNIT ( * ) SI_UNIT ( .MILLI., .METRE. ) );
#14762=CARTESIAN_POINT ( 'NONE',  ( 157.2261751345948539, -3.889087296526011706, -3.889087296526011706 ) ) ;
#14763=ORIENTED_EDGE ( 'NONE', *, *, #18299, .T. ) ;
#14764=FACE_OUTER_BOUND ( 'NONE', #20567, .T. ) ;
#14765=CARTESIAN_POINT ( 'NONE',  ( 160.2187500000000000, 2.485281374238555774, -6.000000000000005329 ) ) ;
#14767=CARTESIAN_POINT ( 'NONE',  ( 0.000000000000000000, 10.00000000000000888, 4.000000000000003553 ) ) ;
#14773=CARTESIAN_POINT ( 'NONE',  ( -0.04610858258174108104, -15.28214019190275330, -7.207076054451203362 ) ) ;
#14774=CARTESIAN_POINT ( 'NONE',  ( 0.000000000000000000, -15.50000000000001421, 5.656854249492387687 ) ) ;
#14776=CARTESIAN_POINT ( 'NONE',  ( 136.5788997308104058, -4.999999999999989342, 2.071067811865468400 ) ) ;
#14778=STYLED_ITEM ( 'NONE', ( #17056 ), #328 ) ;
#14785=SURFACE_STYLE_FILL_AREA ( #19824 ) ;
#14791=ORIENTED_EDGE ( 'NONE', *, *, #20411, .T. ) ;
#14793=CARTESIAN_POINT ( 'NONE',  ( -4.999999999999990230, -55.00000000000002132, -4.000000000000003553 ) ) ;
#14797=( NAMED_UNIT ( * ) SI_UNIT ( $, .STERADIAN. ) SOLID_ANGLE_UNIT ( ) );
#14799=CARTESIAN_POINT ( 'NONE',  ( 140.5000000000000284, 0.000000000000000000, 0.000000000000000000 ) ) ;
#14804=ORIENTED_EDGE ( 'NONE', *, *, #2081, .T. ) ;
#14808=( LENGTH_UNIT ( ) NAMED_UNIT ( * ) SI_UNIT ( .MILLI., .METRE. ) );
#14813=SURFACE_STYLE_USAGE ( .BOTH. , #28748 ) ;
#14820=CARTESIAN_POINT ( 'NONE',  ( 139.8009670889181564, -8.830838033386935848, 8.125417887732853117 ) ) ;
#14821=CARTESIAN_POINT ( 'NONE',  ( 139.7886751345948539, 5.500000000000005329, 0.000000000000000000 ) ) ;
#14822=SURFACE_SIDE_STYLE ('',( #21728 ) ) ;
#14825=CARTESIAN_POINT ( 'NONE',  ( -10.00000000000000178, -19.99999999999998934, -4.000000000000003553 ) ) ;
#14826=VERTEX_POINT ( 'NONE', #1301 ) ;
#14827=CARTESIAN_POINT ( 'NONE',  ( 146.7336002691897079, -4.999999999999989342, 2.071067811865468400 ) ) ;
#14829=CARTESIAN_POINT ( 'NONE',  ( 151.9687500000000284, -2.485281374238585972, 6.000000000000005329 ) ) ;
#14833=CARTESIAN_POINT ( 'NONE',  ( 142.4062500000000568, 6.000000000000005329, -2.485281374238555774 ) ) ;
#14834=CIRCLE ( 'NONE', #20228, 0.4999999999999993894 ) ;
#14839=ORIENTED_EDGE ( 'NONE', *, *, #19363, .T. ) ;
#14844=CIRCLE ( 'NONE', #9449, 1.000000000000000888 ) ;
#14845=CARTESIAN_POINT ( 'NONE',  ( -38.99999999999998579, -59.99999999999980105, 4.000000000000003553 ) ) ;
#14847=EDGE_CURVE ( 'NONE', #12257, #691, #16347, .T. ) ;
#14849=CARTESIAN_POINT ( 'NONE',  ( 143.8050748654052313, 5.500000000000012434, 2.278174593052012309 ) ) ;
#14851=LINE ( 'NONE', #24195, #5122 ) ;
#14859=PRESENTATION_STYLE_ASSIGNMENT (( #12574 ) ) ;
#14862=CARTESIAN_POINT ( 'NONE',  ( 161.0625000000000284, -4.242640687119298093, 4.242640687119298093 ) ) ;
#14863=CARTESIAN_POINT ( 'NONE',  ( 116.0000000000000142, 0.000000000000000000, -5.500000000000000000 ) ) ;
#14866=VERTEX_POINT ( 'NONE', #27103 ) ;
#14877=DIRECTION ( 'NONE',  ( 1.000000000000000000, 0.000000000000000000, 0.000000000000000000 ) ) ;
#14880=ORIENTED_EDGE ( 'NONE', *, *, #4768, .T. ) ;
#14886=CARTESIAN_POINT ( 'NONE',  ( 136.0000000000000284, 0.000000000000000000, 0.000000000000000000 ) ) ;
#14888=FACE_OUTER_BOUND ( 'NONE', #13725, .T. ) ;
#14892=PRESENTATION_STYLE_ASSIGNMENT (( #19785 ) ) ;
#14894=ORIENTED_EDGE ( 'NONE', *, *, #11622, .T. ) ;
#14898=AXIS2_PLACEMENT_3D ( 'NONE', #12133, #24202, #556 ) ;
#14909=CARTESIAN_POINT ( 'NONE',  ( 159.6562500000000568, -6.000000000000005329, 2.485281374238555774 ) ) ;
#14910=EDGE_CURVE ( 'NONE', #9387, #4270, #24028, .T. ) ;
#14916=ORIENTED_EDGE ( 'NONE', *, *, #18744, .F. ) ;
#14918=DIRECTION ( 'NONE',  ( -6.938893903907221278E-15, 1.000000000000000000, 0.000000000000000000 ) ) ;
#14919=EDGE_CURVE ( 'NONE', #28771, #29814, #1940, .T. ) ;
#14922=CARTESIAN_POINT ( 'NONE',  ( 140.7976497308104058, 0.000000000000000000, 5.000000000000004441 ) ) ;
#14926=SURFACE_SIDE_STYLE ('',( #24419 ) ) ;
#14934=DIRECTION ( 'NONE',  ( 0.000000000000000000, 0.000000000000000000, 1.000000000000000000 ) ) ;
#14939=CARTESIAN_POINT ( 'NONE',  ( 136.5937500000000853, 6.000000000000005329, 2.485281374238585972 ) ) ;
#14942=CARTESIAN_POINT ( 'NONE',  ( -39.00000000000000000, -20.00000000000001776, -4.000000000000003553 ) ) ;
#14944=DIRECTION ( 'NONE',  ( 0.000000000000000000, -1.000000000000000000, -0.000000000000000000 ) ) ;
#14946=EDGE_CURVE ( 'NONE', #29963, #3655, #27547, .T. ) ;
#14948=CARTESIAN_POINT ( 'NONE',  ( 159.2576787659436661, -11.08176058204349523, 4.603822987175699488 ) ) ;
#14950=CARTESIAN_POINT ( 'NONE',  ( 159.2886751345948255, 5.500000000000005329, 0.000000000000000000 ) ) ;
#14955=CARTESIAN_POINT ( 'NONE',  ( 0.000000000000000000, -9.500000000000008882, 7.500000000000007105 ) ) ;
#14956=CARTESIAN_POINT ( 'NONE',  ( 158.7976497308104342, 0.000000000000000000, 5.000000000000004441 ) ) ;
#14962=DIRECTION ( 'NONE',  ( 0.000000000000000000, 1.224646799147351482E-16, 1.000000000000000000 ) ) ;
#14963=CARTESIAN_POINT ( 'NONE',  ( 146.3363248654052029, 0.000000000000000000, -5.500000000000005329 ) ) ;
#14967=ORIENTED_EDGE ( 'NONE', *, *, #10438, .T. ) ;
#14968=CARTESIAN_POINT ( 'NONE',  ( 139.9836002691896510, 4.999999999999989342, -2.071067811865468400 ) ) ;
#14969=CARTESIAN_POINT ( 'NONE',  ( 150.3750000000000284, 0.000000000000000000, 6.000000000000005329 ) ) ;
#14974=CARTESIAN_POINT ( 'NONE',  ( 141.5625000000000284, -4.242640687119298093, 4.242640687119298093 ) ) ;
#14975=DIRECTION ( 'NONE',  ( 1.000000000000000000, 0.000000000000000000, 0.000000000000000000 ) ) ;
#14976=AXIS2_PLACEMENT_3D ( 'NONE', #8375, #27104, #4368 ) ;
#14986=AXIS2_PLACEMENT_3D ( 'NONE', #23998, #8006, #12358 ) ;
#14988=FILL_AREA_STYLE ('',( #5583 ) ) ;
#14990=SURFACE_STYLE_FILL_AREA ( #23759 ) ;
#14991=CARTESIAN_POINT ( 'NONE',  ( 135.1771402107524693, -8.419396982537390883, 8.000000000000008882 ) ) ;
#14993=CARTESIAN_POINT ( 'NONE',  ( 136.7738248654052313, -3.889087296526011706, 3.889087296526011706 ) ) ;
#15000=CARTESIAN_POINT ( 'NONE',  ( 154.8898502691896795, 3.535533905932725318, -3.535533905932725318 ) ) ;
#15001=CARTESIAN_POINT ( 'NONE',  ( 141.4761751345948255, 3.889087296526011706, 3.889087296526011706 ) ) ;
#15004=CARTESIAN_POINT ( 'NONE',  ( 1.000000000000000888, -15.13429681935021165, 8.790437860111675050 ) ) ;
#15008=DIRECTION ( 'NONE',  ( 1.000000000000000000, 0.000000000000000000, 0.000000000000000000 ) ) ;
#15009=CARTESIAN_POINT ( 'NONE',  ( 149.3363248654052029, 0.000000000000000000, -5.500000000000005329 ) ) ;
#15010=EDGE_LOOP ( 'NONE', ( #6303, #16717, #16563, #11565 ) ) ;
#15012=SURFACE_SIDE_STYLE ('',( #20233 ) ) ;
#15013=CARTESIAN_POINT ( 'NONE',  ( 0.000000000000000000, -15.50000000000001421, -5.656854249492387687 ) ) ;
#15014=CARTESIAN_POINT ( 'NONE',  ( 146.1636751345948255, 0.000000000000000000, 5.500000000000005329 ) ) ;
#15017=VERTEX_POINT ( 'NONE', #4671 ) ;
#15019=CARTESIAN_POINT ( 'NONE',  ( 146.8125000000000284, 4.242640687119298093, -4.242640687119298093 ) ) ;
#15021=AXIS2_PLACEMENT_3D ( 'NONE', #2195, #16213, #9411 ) ;
#15035=CARTESIAN_POINT ( 'NONE',  ( 152.8988248654052313, 3.889087296526011706, 3.889087296526011706 ) ) ;
#15037=CARTESIAN_POINT ( 'NONE',  ( 154.7738248654052029, -3.889087296526011706, 3.889087296526011706 ) ) ;
#15041=CIRCLE ( 'NONE', #4718, 16.50000000000000355 ) ;
#15046=EDGE_CURVE ( 'NONE', #1053, #24844, #11488, .T. ) ;
#15050=CARTESIAN_POINT ( 'NONE',  ( 139.0238248654052029, 3.889087296526011706, -3.889087296526011706 ) ) ;
#15051=COLOUR_RGB ( '', 0.31764706, 0.68627451, 0.89019608) ;
#15059=VERTEX_POINT ( 'NONE', #20673 ) ;
#15060=CIRCLE ( 'NONE', #1792, 1.000000000000000888 ) ;
#15061=CARTESIAN_POINT ( 'NONE',  ( 135.8586002691897079, 2.071067811865468400, 4.999999999999989342 ) ) ;
#15064=FACE_OUTER_BOUND ( 'NONE', #20553, .T. ) ;
#15069=CARTESIAN_POINT ( 'NONE',  ( 0.9867988441837158842, -16.18254354104136539, -6.670981548062425048 ) ) ;
#15070=CARTESIAN_POINT ( 'NONE',  ( 161.0000000000000284, 0.000000000000000000, 0.000000000000000000 ) ) ;
#15072=CARTESIAN_POINT ( 'NONE',  ( 134.9851497308104058, -3.535533905932725318, 3.535533905932725318 ) ) ;
#15073=CARTESIAN_POINT ( 'NONE',  ( -4.999999999999990230, -55.00000000000002132, 7.500000000000007105 ) ) ;
#15074=LINE ( 'NONE', #13252, #30073 ) ;
#15079=CARTESIAN_POINT ( 'NONE',  ( -40.00000000000000000, -20.00000000000021316, 4.000000000000003553 ) ) ;
#15082=CYLINDRICAL_SURFACE ( 'NONE', #7782, 5.500000000000000000 ) ;
#15085=EDGE_CURVE ( 'NONE', #25883, #27076, #1950, .T. ) ;
#15088=DIRECTION ( 'NONE',  ( 0.000000000000000000, 0.000000000000000000, -1.000000000000000000 ) ) ;
#15090=ORIENTED_EDGE ( 'NONE', *, *, #26937, .F. ) ;
#15091=CIRCLE ( 'NONE', #17556, 15.00000000000000000 ) ;
#15095=FILL_AREA_STYLE_COLOUR ( '', #10702 ) ;
#15097=DIRECTION ( 'NONE',  ( -6.938893903907221278E-15, -1.000000000000000000, 0.000000000000000000 ) ) ;
#15099=EDGE_CURVE ( 'NONE', #11502, #20769, #24491, .T. ) ;
#15100=CARTESIAN_POINT ( 'NONE',  ( 152.1636751345948255, 0.000000000000000000, 5.500000000000005329 ) ) ;
#15102=CARTESIAN_POINT ( 'NONE',  ( 140.6985356443576620, -11.69853564435969773, 4.029618091915731171 ) ) ;
#15103=CIRCLE ( 'NONE', #1842, 1.000000000000000000 ) ;
#15111=CARTESIAN_POINT ( 'NONE',  ( 124.9999999999999432, -71.00000000000001421, 5.000000000000004441 ) ) ;
#15112=CARTESIAN_POINT ( 'NONE',  ( 157.1101497308104058, 3.535533905932725318, 3.535533905932725318 ) ) ;
#15113=AXIS2_PLACEMENT_3D ( 'NONE', #1689, #11087, #20432 ) ;
#15114=CARTESIAN_POINT ( 'NONE',  ( 152.9136751345948539, 0.000000000000000000, -5.500000000000005329 ) ) ;
#15120=EDGE_CURVE ( 'NONE', #18727, #22602, #29402, .T. ) ;
#15126=CARTESIAN_POINT ( 'NONE',  ( 151.6875000000000284, 4.242640687119269671, 4.242640687119298093 ) ) ;
#15133=ORIENTED_EDGE ( 'NONE', *, *, #25087, .T. ) ;
#15134=CARTESIAN_POINT ( 'NONE',  ( 146.7187500000000284, 2.485281374238555774, -6.000000000000005329 ) ) ;
#15135=CARTESIAN_POINT ( 'NONE',  ( 143.1488248654052029, -3.889087296526011706, -3.889087296526011706 ) ) ;
#15146=( LENGTH_UNIT ( ) NAMED_UNIT ( * ) SI_UNIT ( .MILLI., .METRE. ) );
#15147=CARTESIAN_POINT ( 'NONE',  ( 148.3988248654052313, 3.889087296526011706, 3.889087296526011706 ) ) ;
#15148=DIRECTION ( 'NONE',  ( 0.000000000000000000, -0.8787878787878796727, 0.4772125984249564468 ) ) ;
#15157=CARTESIAN_POINT ( 'NONE',  ( 116.0000000000000142, 0.000000000000000000, 0.000000000000000000 ) ) ;
#15160=CARTESIAN_POINT ( 'NONE',  ( 152.2648502691896510, 3.535533905932725318, 3.535533905932752852 ) ) ;
#15161=CARTESIAN_POINT ( 'NONE',  ( 150.4761751345948255, 3.889087296526011706, 3.889087296526011706 ) ) ;
#15168=( NAMED_UNIT ( * ) SI_UNIT ( $, .STERADIAN. ) SOLID_ANGLE_UNIT ( ) );
#15169=CARTESIAN_POINT ( 'NONE',  ( -9.529120656610874963E-19, -15.46245447015412111, 5.965482872545659454 ) ) ;
#15172=EDGE_LOOP ( 'NONE', ( #29719, #3619, #24552, #16531, #29418, #6347, #20237, #18356, #25386 ) ) ;
#15180=CARTESIAN_POINT ( 'NONE',  ( -0.5000000000000004441, -15.00000000000001421, 7.500000000000007105 ) ) ;
#15182=MECHANICAL_DESIGN_GEOMETRIC_PRESENTATION_REPRESENTATION('',(#11281),#18644);
#15187=CARTESIAN_POINT ( 'NONE',  ( 146.4449251345949108, -5.500000000000012434, 2.278174593052012309 ) ) ;
#15194=CARTESIAN_POINT ( 'NONE',  ( -0.9018315097318243545, -9.098168490268061959, 4.000092554054210936 ) ) ;
#15196=EDGE_CURVE ( 'NONE', #17215, #19511, #27848, .T. ) ;
#15197=CARTESIAN_POINT ( 'NONE',  ( 159.8511751345948539, -3.889087296526011706, 3.889087296526011706 ) ) ;
#15198=ADVANCED_FACE ( 'NONE', ( #15589 ), #26941, .T. ) ;
#15201=SURFACE_STYLE_USAGE ( .BOTH. , #29604 ) ;
#15203=ORIENTED_EDGE ( 'NONE', *, *, #24816, .T. ) ;
#15206=LINE ( 'NONE', #24394, #12513 ) ;
#15212=CARTESIAN_POINT ( 'NONE',  ( 136.0000000000000284, -9.165151389911669000, 8.000000000000007105 ) ) ;
#15216=ORIENTED_EDGE ( 'NONE', *, *, #28548, .F. ) ;
#15218=CARTESIAN_POINT ( 'NONE',  ( 157.1250000000000284, 0.000000000000000000, -6.000000000000005329 ) ) ;
#15219=AXIS2_PLACEMENT_3D ( 'NONE', #5436, #242, #28339 ) ;
#15226=ORIENTED_EDGE ( 'NONE', *, *, #28782, .F. ) ;
#15228=CARTESIAN_POINT ( 'NONE',  ( 0.8616410392485300829, -15.74614809565155404, -7.643977401085323642 ) ) ;
#15230=CYLINDRICAL_SURFACE ( 'NONE', #1459, 5.500000000000000000 ) ;
#15231=CARTESIAN_POINT ( 'NONE',  ( -4.999999999999990230, -55.00000000000002132, 7.500000000000007105 ) ) ;
#15233=CARTESIAN_POINT ( 'NONE',  ( 0.1092220458218999685, -15.15144499995605365, -8.760684001891156925 ) ) ;
#15236=DIRECTION ( 'NONE',  ( 1.000000000000000000, 0.000000000000000000, 0.000000000000000000 ) ) ;
#15239=AXIS2_PLACEMENT_3D ( 'NONE', #615, #19085, #9848 ) ;
#15240=EDGE_CURVE ( 'NONE', #18697, #8808, #11301, .T. ) ;
#15243=ORIENTED_EDGE ( 'NONE', *, *, #5834, .T. ) ;
#15245=CARTESIAN_POINT ( 'NONE',  ( -0.5000000000000004441, -9.500000000000008882, -5.000000000000004441 ) ) ;
#15248=DIRECTION ( 'NONE',  ( 1.000000000000000000, 0.000000000000000000, 0.000000000000000000 ) ) ;
#15258=VERTEX_POINT ( 'NONE', #4011 ) ;
#15265=EDGE_CURVE ( 'NONE', #18576, #19330, #30281, .T. ) ;
#15267=CARTESIAN_POINT ( 'NONE',  ( 137.1636751345948255, 0.000000000000000000, 5.500000000000005329 ) ) ;
#15271=CARTESIAN_POINT ( 'NONE',  ( 150.6413997308104342, 2.071067811865468400, -4.999999999999989342 ) ) ;
#15281=AXIS2_PLACEMENT_3D ( 'NONE', #20817, #14384, #16385 ) ;
#15284=AXIS2_PLACEMENT_3D ( 'NONE', #17019, #9787, #5295 ) ;
#15287=CIRCLE ( 'NONE', #2023, 1.000000000000000888 ) ;
#15288=CARTESIAN_POINT ( 'NONE',  ( 148.9687500000000284, -2.485281374238585972, 6.000000000000005329 ) ) ;
#15289=CARTESIAN_POINT ( 'NONE',  ( 141.0000000000000284, -54.99999999999989342, 5.000000000000004441 ) ) ;
#15291=AXIS2_PLACEMENT_3D ( 'NONE', #23364, #19199, #23799 ) ;
#15294=VERTEX_POINT ( 'NONE', #16500 ) ;
#15295=CARTESIAN_POINT ( 'NONE',  ( 144.7500000000000568, -6.000000000000005329, 0.000000000000000000 ) ) ;
#15296=CARTESIAN_POINT ( 'NONE',  ( 161.2890952447136499, -5.450977163394726155, 1.974987045907475869 ) ) ;
#15297=STYLED_ITEM ( 'NONE', ( #27055 ), #23960 ) ;
#15303=ORIENTED_EDGE ( 'NONE', *, *, #27396, .F. ) ;
#15311=AXIS2_PLACEMENT_3D ( 'NONE', #27660, #1568, #20631 ) ;
#15313=CARTESIAN_POINT ( 'NONE',  ( 116.0000000000000142, 0.000000000000000000, 0.000000000000000000 ) ) ;
#15319=CARTESIAN_POINT ( 'NONE',  ( 124.9999999999999432, -70.00000000000000000, -7.500000000000007105 ) ) ;
#15320=AXIS2_PLACEMENT_3D ( 'NONE', #20600, #13880, #8927 ) ;
#15323=CARTESIAN_POINT ( 'NONE',  ( 137.3511751345948255, -3.889087296526011706, 3.889087296526011706 ) ) ;
#15327=FACE_OUTER_BOUND ( 'NONE', #2715, .T. ) ;
#15329=CARTESIAN_POINT ( 'NONE',  ( 135.7425748654052029, -2.278174593052352925, -5.499999999999671374 ) ) ;
#15330=VECTOR ( 'NONE', #24092, 1000.000000000000000 ) ;
#15332=CARTESIAN_POINT ( 'NONE',  ( 13.99999999999999822, 0.000000000000000000, 0.000000000000000000 ) ) ;
#15333=FACE_OUTER_BOUND ( 'NONE', #5651, .T. ) ;
#15339=DIRECTION ( 'NONE',  ( 0.000000000000000000, 0.000000000000000000, 1.000000000000000000 ) ) ;
#15346=AXIS2_PLACEMENT_3D ( 'NONE', #3049, #28249, #9987 ) ;
#15347=VERTEX_POINT ( 'NONE', #12783 ) ;
#15352=DIRECTION ( 'NONE',  ( 0.000000000000000000, 0.8787878787878786735, 0.4772125984249585562 ) ) ;
#15359=CARTESIAN_POINT ( 'NONE',  ( 155.4300748654052029, 2.278174593051818686, -5.500000000000204281 ) ) ;
#15367=CARTESIAN_POINT ( 'NONE',  ( 137.9136751345948539, 0.000000000000000000, -5.500000000000005329 ) ) ;
#15368=FACE_OUTER_BOUND ( 'NONE', #25947, .T. ) ;
#15370=CARTESIAN_POINT ( 'NONE',  ( 135.0000000000000284, -8.261054798780170572, 8.006597766721364806 ) ) ;
#15371=ORIENTED_EDGE ( 'NONE', *, *, #15602, .F. ) ;
#15373=DIRECTION ( 'NONE',  ( 0.000000000000000000, 0.000000000000000000, 1.000000000000000000 ) ) ;
#15378=ORIENTED_EDGE ( 'NONE', *, *, #19325, .F. ) ;
#15382=ORIENTED_EDGE ( 'NONE', *, *, #6846, .T. ) ;
#15383=CARTESIAN_POINT ( 'NONE',  ( 159.0000000000000284, 6.000000000000005329, 0.000000000000000000 ) ) ;
#15384=EDGE_CURVE ( 'NONE', #7800, #20811, #27936, .T. ) ;
#15389=ORIENTED_EDGE ( 'NONE', *, *, #22403, .T. ) ;
#15395=VERTEX_POINT ( 'NONE', #775 ) ;
#15399=CARTESIAN_POINT ( 'NONE',  ( 160.5164690628317317, -11.32153369091806461, -3.978831925134524106 ) ) ;
#15400=CARTESIAN_POINT ( 'NONE',  ( 135.0000000000000284, 0.000000000000000000, -12.00000000000000178 ) ) ;
#15405=DIRECTION ( 'NONE',  ( -0.000000000000000000, -0.000000000000000000, -1.000000000000000000 ) ) ;
#15406=CARTESIAN_POINT ( 'NONE',  ( 147.9449251345948539, -5.500000000000012434, 2.278174593052012309 ) ) ;
#15407=DIRECTION ( 'NONE',  ( -1.000000000000000000, 3.469446951953694061E-16, -0.000000000000000000 ) ) ;
#15409=AXIS2_PLACEMENT_3D ( 'NONE', #21842, #28876, #789 ) ;
#15411=CARTESIAN_POINT ( 'NONE',  ( 124.9999999999999432, -70.00000000000000000, 5.000000000000004441 ) ) ;
#15412=CARTESIAN_POINT ( 'NONE',  ( 160.5863248654052597, 0.000000000000000000, 5.500000000000005329 ) ) ;
#15415=CYLINDRICAL_SURFACE ( 'NONE', #250, 0.5000000000000004441 ) ;
#15417=VERTEX_POINT ( 'NONE', #17383 ) ;
#15424=DIRECTION ( 'NONE',  ( 0.000000000000000000, 0.000000000000000000, -1.000000000000000000 ) ) ;
#15425=CARTESIAN_POINT ( 'NONE',  ( 142.6875000000000284, 4.242640687119269671, 4.242640687119298093 ) ) ;
#15429=CARTESIAN_POINT ( 'NONE',  ( 135.8363248654052029, 0.000000000000000000, -5.500000000000005329 ) ) ;
#15431=CARTESIAN_POINT ( 'NONE',  ( 159.1011751345948255, 3.889087296526011706, -3.889087296526011706 ) ) ;
#15436=CARTESIAN_POINT ( 'NONE',  ( 148.5788997308104058, -4.999999999999989342, 2.071067811865468400 ) ) ;
#15437=DIRECTION ( 'NONE',  ( 0.000000000000000000, 0.7999999999999996003, -0.6000000000000006439 ) ) ;
#15438=CYLINDRICAL_SURFACE ( 'NONE', #20436, 5.500000000000000000 ) ;
#15439=CARTESIAN_POINT ( 'NONE',  ( 135.3652387094614085, -8.709367079857635474, 8.045772721957300533 ) ) ;
#15452=CARTESIAN_POINT ( 'NONE',  ( 148.4062500000000568, 6.000000000000005329, -2.485281374238556218 ) ) ;
#15454=EDGE_CURVE ( 'NONE', #26763, #27165, #27913, .T. ) ;
#15457=CARTESIAN_POINT ( 'NONE',  ( 145.5000000000000284, 6.000000000000005329, 0.000000000000000000 ) ) ;
#15458=DIRECTION ( 'NONE',  ( 0.000000000000000000, 0.000000000000000000, 1.000000000000000000 ) ) ;
#15459=ORIENTED_EDGE ( 'NONE', *, *, #5647, .T. ) ;
#15462=ORIENTED_EDGE ( 'NONE', *, *, #1470, .F. ) ;
#15465=VERTEX_POINT ( 'NONE', #14774 ) ;
#15469=DIRECTION ( 'NONE',  ( 1.000000000000000000, -0.000000000000000000, -0.000000000000000000 ) ) ;
#15470=CARTESIAN_POINT ( 'NONE',  ( 135.6335788417890740, -8.691129701112460637, -8.179621397165890428 ) ) ;
#15471=VECTOR ( 'NONE', #13475, 1000.000000000000000 ) ;
#15475=CARTESIAN_POINT ( 'NONE',  ( 136.9613248654052313, -5.500000000000005329, 0.000000000000000000 ) ) ;
#15476=CARTESIAN_POINT ( 'NONE',  ( 156.0863248654052597, 0.000000000000000000, 5.500000000000005329 ) ) ;
#15479=SURFACE_STYLE_FILL_AREA ( #3143 ) ;
#15482=CARTESIAN_POINT ( 'NONE',  ( 150.7648502691896510, 3.535533905932725318, 3.535533905932752852 ) ) ;
#15483=CARTESIAN_POINT ( 'NONE',  ( 150.0074251345948539, 2.278174593052043395, -5.499999999999981348 ) ) ;
#15487=EDGE_CURVE ( 'NONE', #12929, #12702, #2444, .T. ) ;
#15492=CARTESIAN_POINT ( 'NONE',  ( -10.00000000000000178, -19.99999999999998934, -4.000000000000003553 ) ) ;
#15494=CARTESIAN_POINT ( 'NONE',  ( 145.6011751345948539, 3.889087296526011706, -3.889087296526011706 ) ) ;
#15498=EDGE_CURVE ( 'NONE', #11567, #12257, #27042, .T. ) ;
#15499=VERTEX_POINT ( 'NONE', #28560 ) ;
#15511=FACE_OUTER_BOUND ( 'NONE', #17822, .T. ) ;
#15515=CARTESIAN_POINT ( 'NONE',  ( -0.5631067912581170232, -9.873786417483767508, 4.496381089953940702 ) ) ;
#15518=TOROIDAL_SURFACE ( 'NONE', #27236, 1.000000000000000000, 0.5000000000000000000 ) ;
#15519=TOROIDAL_SURFACE ( 'NONE', #7619, 10.49999999999999822, 0.5000000000000000000 ) ;
#15521=CARTESIAN_POINT ( 'NONE',  ( 141.3824251345948539, 5.500000000000012434, 2.278174593052012309 ) ) ;
#15526=EDGE_CURVE ( 'NONE', #476, #3609, #26415, .T. ) ;
#15532=CARTESIAN_POINT ( 'NONE',  ( 139.4925748654052313, 2.278174593052074925, 5.499999999999950262 ) ) ;
#15535=CARTESIAN_POINT ( 'NONE',  ( 156.8363248654052313, 0.000000000000000000, -5.500000000000005329 ) ) ;
#15539=ORIENTED_EDGE ( 'NONE', *, *, #16603, .T. ) ;
#15540=CARTESIAN_POINT ( 'NONE',  ( 154.5937500000000284, 6.000000000000005329, 2.485281374238585972 ) ) ;
#15543=ORIENTED_EDGE ( 'NONE', *, *, #9187, .F. ) ;
#15544=CARTESIAN_POINT ( 'NONE',  ( 151.0386751345948539, -5.500000000000005329, 0.000000000000000000 ) ) ;
#15547=MECHANICAL_DESIGN_GEOMETRIC_PRESENTATION_REPRESENTATION('',(#9128),#12599);
#15548=DIRECTION ( 'NONE',  ( 0.000000000000000000, 0.000000000000000000, -1.000000000000000000 ) ) ;
#15552=DIRECTION ( 'NONE',  ( -1.000000000000000000, -0.000000000000000000, -0.000000000000000000 ) ) ;
#15554=CARTESIAN_POINT ( 'NONE',  ( 159.5629673084600597, -11.38634829877173438, -3.839848799536992097 ) ) ;
#15556=CARTESIAN_POINT ( 'NONE',  ( 0.1053031288715573777, -15.23283975038563298, -8.619984219653423096 ) ) ;
#15559=TOROIDAL_SURFACE ( 'NONE', #15021, 12.50000000000000178, 0.5000000000000000000 ) ;
#15562=CARTESIAN_POINT ( 'NONE',  ( 140.0000000000000284, -8.500000000000007105, -7.500000000000007105 ) ) ;
#15563=DIRECTION ( 'NONE',  ( -0.000000000000000000, -0.000000000000000000, -1.000000000000000000 ) ) ;
#15571=EDGE_CURVE ( 'NONE', #12687, #28026, #5353, .T. ) ;
#15572=CARTESIAN_POINT ( 'NONE',  ( 138.7648502691896795, 3.535533905932725318, 3.535533905932752852 ) ) ;
#15573=ORIENTED_EDGE ( 'NONE', *, *, #17980, .T. ) ;
#15574=AXIS2_PLACEMENT_3D ( 'NONE', #20618, #29967, #2177 ) ;
#15576=SURFACE_STYLE_FILL_AREA ( #17558 ) ;
#15582=CARTESIAN_POINT ( 'NONE',  ( 138.4761751345948539, 3.889087296526011706, 3.889087296526011706 ) ) ;
#15583=CARTESIAN_POINT ( 'NONE',  ( 141.4687500000000568, -2.485281374238585972, 6.000000000000005329 ) ) ;
#15585=CARTESIAN_POINT ( 'NONE',  ( 161.0000000000000284, 0.000000000000000000, 0.000000000000000000 ) ) ;
#15589=FACE_OUTER_BOUND ( 'NONE', #26655, .T. ) ;
#15592=CARTESIAN_POINT ( 'NONE',  ( 147.5476497308104058, 0.000000000000000000, -5.000000000000004441 ) ) ;
#15595=DIRECTION ( 'NONE',  ( 0.000000000000000000, -0.000000000000000000, 1.000000000000000000 ) ) ;
#15596=FILL_AREA_STYLE ('',( #10661 ) ) ;
#15601=ORIENTED_EDGE ( 'NONE', *, *, #13847, .T. ) ;
#15602=EDGE_CURVE ( 'NONE', #23117, #2429, #1521, .T. ) ;
#15609=CARTESIAN_POINT ( 'NONE',  ( 148.7812500000000568, 2.485281374238585972, 6.000000000000005329 ) ) ;
#15610=CARTESIAN_POINT ( 'NONE',  ( 140.0000000000000284, -54.99999999999990763, 7.500000000000007105 ) ) ;
#15615=CARTESIAN_POINT ( 'NONE',  ( 135.8437500000000284, -6.000000000000005329, -2.485281374238555774 ) ) ;
#15616=CARTESIAN_POINT ( 'NONE',  ( -4.999999999999990230, -55.00000000000002132, -7.500000000000007105 ) ) ;
#15629=CYLINDRICAL_SURFACE ( 'NONE', #12657, 1.000000000000000000 ) ;
#15630=CARTESIAN_POINT ( 'NONE',  ( 135.8076776779767272, -8.774823127787460209, -8.164319474386353193 ) ) ;
#15635=FACE_OUTER_BOUND ( 'NONE', #7583, .T. ) ;
#15639=CARTESIAN_POINT ( 'NONE',  ( 152.3586002691896510, 2.071067811865468400, 4.999999999999989342 ) ) ;
#15648=CARTESIAN_POINT ( 'NONE',  ( 156.0000000000000284, 6.000000000000005329, 0.000000000000000000 ) ) ;
#15661=SHAPE_REPRESENTATION ( 'Fixed Jaw', ( #18805 ), #19755 ) ;
#15664=EDGE_CURVE ( 'NONE', #16115, #28288, #591, .T. ) ;
#15676=PRESENTATION_STYLE_ASSIGNMENT (( #15201 ) ) ;
#15677=CARTESIAN_POINT ( 'NONE',  ( -15.49999999999999289, -25.00000000000007816, -7.500000000000007105 ) ) ;
#15679=ORIENTED_EDGE ( 'NONE', *, *, #10185, .F. ) ;
#15692=CARTESIAN_POINT ( 'NONE',  ( 158.0625000000000284, -4.242640687119298093, 4.242640687119298093 ) ) ;
#15695=ORIENTED_EDGE ( 'NONE', *, *, #2646, .F. ) ;
#15700=CARTESIAN_POINT ( 'NONE',  ( 159.1354668258956053, -11.07692307937646348, 4.615384609496523183 ) ) ;
#15707=CARTESIAN_POINT ( 'NONE',  ( -4.999999999999990230, -55.00000000000002132, 8.000000000000007105 ) ) ;
#15715=FACE_OUTER_BOUND ( 'NONE', #27796, .T. ) ;
#15720=PLANE ( 'NONE',  #27407 ) ;
#15724=CARTESIAN_POINT ( 'NONE',  ( 137.9211002691896795, -4.999999999999989342, -2.071067811865468400 ) ) ;
#15728=SURFACE_STYLE_USAGE ( .BOTH. , #3991 ) ;
#15731=ORIENTED_EDGE ( 'NONE', *, *, #8784, .T. ) ;
#15733=CARTESIAN_POINT ( 'NONE',  ( 139.5000000000000284, 6.000000000000005329, 0.000000000000000000 ) ) ;
#15736=PRESENTATION_STYLE_ASSIGNMENT (( #29660 ) ) ;
#15738=ADVANCED_FACE ( 'NONE', ( #4990 ), #23757, .F. ) ;
#15742=DIRECTION ( 'NONE',  ( 1.000000000000000000, 0.000000000000000000, 0.000000000000000000 ) ) ;
#15744=TOROIDAL_SURFACE ( 'NONE', #11821, 16.00000000000000000, 1.000000000000000000 ) ;
#15745=CARTESIAN_POINT ( 'NONE',  ( 152.6101497308104058, 3.535533905932725318, 3.535533905932725318 ) ) ;
#15748=CIRCLE ( 'NONE', #24495, 1.000000000000000888 ) ;
#15749=LINE ( 'NONE', #4171, #7427 ) ;
#15752=EDGE_CURVE ( 'NONE', #7302, #14866, #6880, .T. ) ;
#15756=DIRECTION ( 'NONE',  ( 0.000000000000000000, 0.000000000000000000, -1.000000000000000000 ) ) ;
#15762=EDGE_LOOP ( 'NONE', ( #14311, #1165, #23314 ) ) ;
#15764=CARTESIAN_POINT ( 'NONE',  ( 143.1562500000000284, -6.000000000000005329, 2.485281374238556218 ) ) ;
#15765=CYLINDRICAL_SURFACE ( 'NONE', #22180, 1.000000000000000000 ) ;
#15767=COLOUR_RGB ( '', 0.40784314, 0.44705882, 0.49803922) ;
#15768=CARTESIAN_POINT ( 'NONE',  ( 140.2370868712064862, -11.61854343560322711, -4.230991509104584658 ) ) ;
#15770=CARTESIAN_POINT ( 'NONE',  ( 139.5000000000000284, 6.000000000000005329, 0.000000000000000000 ) ) ;
#15773=B_SPLINE_CURVE_WITH_KNOTS ( 'NONE', 3,
 ( #7585, #8344, #17597, #3416, #1121, #26617, #27226, #1430, #22186, #12842, #22498, #8501, #5723, #17442, #8036, #10519, #15296, #1590, #10842, #20195, #5877, #24464, #29545, #17750, #6198, #27075, #22649, #19872, #24784, #29218, #26913, #17908 ),
 .UNSPECIFIED., .F., .F.,
 ( 4, 2, 2, 2, 2, 2, 2, 2, 2, 2, 2, 2, 2, 2, 2, 4 ),
 ( 1.116565195435206273E-15, 0.001893041221572642650, 0.002839561832358405719, 0.003786082443144169005, 0.004732603053929931858, 0.005679123664715694277, 0.006625644275501457563, 0.007572164886287220849, 0.008518685497072985002, 0.009465206107858748288, 0.01041172671864451157, 0.01135824732943027313, 0.01230476794021603641, 0.01325128855100179970, 0.01419780916178756298, 0.01514432977257332627 ),
 .UNSPECIFIED. ) ;
#15777=ORIENTED_EDGE ( 'NONE', *, *, #14420, .F. ) ;
#15779=EDGE_CURVE ( 'NONE', #20769, #22758, #9777, .T. ) ;
#15786=( GEOMETRIC_REPRESENTATION_CONTEXT ( 3 ) GLOBAL_UNCERTAINTY_ASSIGNED_CONTEXT ( ( #25943 ) ) GLOBAL_UNIT_ASSIGNED_CONTEXT ( ( #4123, #23199, #22884 ) ) REPRESENTATION_CONTEXT ( 'NONE', 'WORKASPACE' ) );
#15788=AXIS2_PLACEMENT_3D ( 'NONE', #15157, #991, #8051 ) ;
#15790=CARTESIAN_POINT ( 'NONE',  ( 139.5000000000000284, -8.946933499675683521, -8.000000000000007105 ) ) ;
#15791=CARTESIAN_POINT ( 'NONE',  ( 156.1800748654052882, -2.278174593052098018, 5.499999999999928058 ) ) ;
#15796=CARTESIAN_POINT ( 'NONE',  ( 149.9136751345948539, 0.000000000000000000, -5.500000000000005329 ) ) ;
#15800=LINE ( 'NONE', #3444, #22969 ) ;
#15803=EDGE_LOOP ( 'NONE', ( #13651, #24245, #25341, #3843 ) ) ;
#15804=CARTESIAN_POINT ( 'NONE',  ( 157.9687500000000284, -2.485281374238585972, 6.000000000000005329 ) ) ;
#15807=VECTOR ( 'NONE', #692, 1000.000000000000000 ) ;
#15809=ORIENTED_EDGE ( 'NONE', *, *, #1059, .F. ) ;
#15811=AXIS2_PLACEMENT_3D ( 'NONE', #16889, #18736, #21628 ) ;
#15818=DIRECTION ( 'NONE',  ( -0.000000000000000000, -1.000000000000000000, -0.000000000000000000 ) ) ;
#15819=CARTESIAN_POINT ( 'NONE',  ( 140.5000000000000284, -9.599999999999997868, -7.200000000000011724 ) ) ;
#15820=CARTESIAN_POINT ( 'NONE',  ( 0.8631338372297875372, -15.37878787878788067, 8.351220472436777342 ) ) ;
#15822=( NAMED_UNIT ( * ) PLANE_ANGLE_UNIT ( ) SI_UNIT ( $, .RADIAN. ) );
#15824=PRESENTATION_STYLE_ASSIGNMENT (( #27424 ) ) ;
#15828=CARTESIAN_POINT ( 'NONE',  ( -0.05791364201276149454, -14.59225860131173924, 8.264570319127788167 ) ) ;
#15834=CARTESIAN_POINT ( 'NONE',  ( 159.8586002691896795, 2.071067811865468400, 4.999999999999989342 ) ) ;
#15836=CARTESIAN_POINT ( 'NONE',  ( 0.7579858402826514796, -15.51661825218675261, 8.092275262135514069 ) ) ;
#15844=AXIS2_PLACEMENT_3D ( 'NONE', #13099, #5981, #25016 ) ;
#15848=ORIENTED_EDGE ( 'NONE', *, *, #24279, .F. ) ;
#15849=CARTESIAN_POINT ( 'NONE',  ( 141.0000000000000284, -54.99999999999989342, -4.000000000000003553 ) ) ;
#15850=ORIENTED_EDGE ( 'NONE', *, *, #16432, .T. ) ;
#15851=CARTESIAN_POINT ( 'NONE',  ( 159.3750000000000568, 0.000000000000000000, 6.000000000000005329 ) ) ;
#15852=ORIENTED_EDGE ( 'NONE', *, *, #10363, .F. ) ;
#15860=FILL_AREA_STYLE_COLOUR ( '', #339 ) ;
#15861=CYLINDRICAL_SURFACE ( 'NONE', #27011, 5.500000000000000000 ) ;
#15866=DIRECTION ( 'NONE',  ( -0.000000000000000000, 1.000000000000000000, 0.000000000000000000 ) ) ;
#15867=CARTESIAN_POINT ( 'NONE',  ( 0.8353273635461547775, -15.41366153578293563, -8.287000568860444005 ) ) ;
#15874=DIRECTION ( 'NONE',  ( -1.000000000000000000, 0.000000000000000000, 0.000000000000000000 ) ) ;
#15881=CARTESIAN_POINT ( 'NONE',  ( 139.7961002691896510, 2.071067811865468400, -4.999999999999989342 ) ) ;
#15885=EDGE_CURVE ( 'NONE', #27983, #17415, #4285, .T. ) ;
#15889=ORIENTED_EDGE ( 'NONE', *, *, #4870, .T. ) ;
#15891=CARTESIAN_POINT ( 'NONE',  ( 159.5331181682643944, -12.11593836010622738, 3.856815297222582650 ) ) ;
#15892=CARTESIAN_POINT ( 'NONE',  ( 141.9375000000000284, -4.242640687119298093, -4.242640687119298093 ) ) ;
#15893=ADVANCED_FACE ( 'NONE', ( #21603 ), #24513, .F. ) ;
#15894=ORIENTED_EDGE ( 'NONE', *, *, #17955, .F. ) ;
#15898=( NAMED_UNIT ( * ) SI_UNIT ( $, .STERADIAN. ) SOLID_ANGLE_UNIT ( ) );
#15903=CARTESIAN_POINT ( 'NONE',  ( 135.1771402107443407, -8.419396982527448614, -8.000000000000007105 ) ) ;
#15904=AXIS2_PLACEMENT_3D ( 'NONE', #16557, #14253, #26024 ) ;
#15905=CARTESIAN_POINT ( 'NONE',  ( 152.5163997308104058, 4.999999999999989342, 2.071067811865468400 ) ) ;
#15906=CARTESIAN_POINT ( 'NONE',  ( 140.5000000000000284, -10.00000000000000888, 7.500000000000007105 ) ) ;
#15907=CARTESIAN_POINT ( 'NONE',  ( 141.0000000000000284, -8.500000000000007105, -5.000000000000004441 ) ) ;
#15909=CARTESIAN_POINT ( 'NONE',  ( -4.999999999999886313, -15.00000000000001421, 8.000000000000007105 ) ) ;
#15920=CARTESIAN_POINT ( 'NONE',  ( 146.3437500000000284, -6.000000000000005329, -2.485281374238556218 ) ) ;
#15921=CARTESIAN_POINT ( 'NONE',  ( 160.9487148452246572, -11.55421731372604377, -3.248622259074093854 ) ) ;
#15922=ADVANCED_FACE ( 'NONE', ( #2149 ), #20582, .F. ) ;
#15923=SURFACE_SIDE_STYLE ('',( #6499 ) ) ;
#15924=CARTESIAN_POINT ( 'NONE',  ( 137.3437500000000568, -6.000000000000005329, -2.485281374238555774 ) ) ;
#15925=CARTESIAN_POINT ( 'NONE',  ( -4.999999999999990230, -24.99999999999999289, -7.500000000000007105 ) ) ;
#15929=EDGE_LOOP ( 'NONE', ( #8608, #13851, #8298, #25443 ) ) ;
#15945=CARTESIAN_POINT ( 'NONE',  ( 149.0773502691896510, 5.000000000000004441, 0.000000000000000000 ) ) ;
#15948=FACE_OUTER_BOUND ( 'NONE', #28877, .T. ) ;
#15950=LINE ( 'NONE', #28015, #25149 ) ;
#15956=CARTESIAN_POINT ( 'NONE',  ( 153.8437500000000284, -6.000000000000005329, -2.485281374238555774 ) ) ;
#15961=VERTEX_POINT ( 'NONE', #17768 ) ;
#15966=( NAMED_UNIT ( * ) SI_UNIT ( $, .STERADIAN. ) SOLID_ANGLE_UNIT ( ) );
#15970=ORIENTED_EDGE ( 'NONE', *, *, #1820, .T. ) ;
#15972=CYLINDRICAL_SURFACE ( 'NONE', #22676, 1.000000000000000888 ) ;
#15973=CARTESIAN_POINT ( 'NONE',  ( 140.1537810142820604, -9.001257532780330806, 7.936737533466877714 ) ) ;
#15980=CARTESIAN_POINT ( 'NONE',  ( 160.0461002691896795, -2.071067811865468400, 4.999999999999989342 ) ) ;
#15982=CARTESIAN_POINT ( 'NONE',  ( -0.08076307744279384582, -15.22030785687954157, 7.625468407401369220 ) ) ;
#15989=DIRECTION ( 'NONE',  ( 0.000000000000000000, 0.000000000000000000, 1.000000000000000000 ) ) ;
#15993=AXIS2_PLACEMENT_3D ( 'NONE', #7666, #19372, #14620 ) ;
#15996=ORIENTED_EDGE ( 'NONE', *, *, #5279, .T. ) ;
#16000=CARTESIAN_POINT ( 'NONE',  ( 151.8750000000000284, 0.000000000000000000, 6.000000000000005329 ) ) ;
#16005=VERTEX_POINT ( 'NONE', #14845 ) ;
#16008=CARTESIAN_POINT ( 'NONE',  ( -0.5000000000000004441, -14.50000000000001243, 8.000000000000007105 ) ) ;
#16009=CARTESIAN_POINT ( 'NONE',  ( -20.99999999999998224, -25.00000000000010658, 5.000000000000004441 ) ) ;
#16010=VERTEX_POINT ( 'NONE', #27087 ) ;
#16028=EDGE_LOOP ( 'NONE', ( #25029, #6172, #10905, #22879 ) ) ;
#16032=CARTESIAN_POINT ( 'NONE',  ( 141.7648502691896510, 3.535533905932725318, 3.535533905932752852 ) ) ;
#16033=ADVANCED_FACE ( 'NONE', ( #3133 ), #15744, .F. ) ;
#16036=CARTESIAN_POINT ( 'NONE',  ( 151.4925748654052029, 2.278174593051965235, 5.500000000000058620 ) ) ;
#16043=CARTESIAN_POINT ( 'NONE',  ( 0.000000000000000000, 0.000000000000000000, 0.000000000000000000 ) ) ;
#16044=CARTESIAN_POINT ( 'NONE',  ( 142.4062500000000568, 6.000000000000005329, -2.485281374238555774 ) ) ;
#16046=EDGE_LOOP ( 'NONE', ( #8095, #22531, #29621, #26829 ) ) ;
#16048=VECTOR ( 'NONE', #4176, 1000.000000000000000 ) ;
#16051=CYLINDRICAL_SURFACE ( 'NONE', #446, 5.500000000000000000 ) ;
#16054=CARTESIAN_POINT ( 'NONE',  ( 141.7351497308104058, 3.535533905932725318, -3.535533905932725318 ) ) ;
#16056=CARTESIAN_POINT ( 'NONE',  ( 116.0000000000000142, 0.000000000000000000, -5.500000000000000000 ) ) ;
#16057=ADVANCED_FACE ( 'NONE', ( #17156 ), #19885, .F. ) ;
#16058=CARTESIAN_POINT ( 'NONE',  ( 125.0000000000000568, -55.00000000000000711, 8.000000000000007105 ) ) ;
#16061=( NAMED_UNIT ( * ) SI_UNIT ( $, .STERADIAN. ) SOLID_ANGLE_UNIT ( ) );
#16069=EDGE_CURVE ( 'NONE', #9311, #16823, #6385, .T. ) ;
#16071=LINE ( 'NONE', #11605, #1811 ) ;
#16074=CARTESIAN_POINT ( 'NONE',  ( 142.5937500000000568, 6.000000000000005329, 2.485281374238585972 ) ) ;
#16076=CARTESIAN_POINT ( 'NONE',  ( 139.9687500000000284, -2.485281374238585972, 6.000000000000005329 ) ) ;
#16085=EDGE_LOOP ( 'NONE', ( #22994, #164, #9081, #9383 ) ) ;
#16092=CARTESIAN_POINT ( 'NONE',  ( 139.8812274360932122, -9.071603356455097966, -7.858226389042775928 ) ) ;
#16094=CARTESIAN_POINT ( 'NONE',  ( -0.5000000000000009992, -10.00000000000000888, 5.000000000000004441 ) ) ;
#16097=STYLED_ITEM ( 'NONE', ( #18204 ), #4571 ) ;
#16103=CARTESIAN_POINT ( 'NONE',  ( 147.5773502691896795, 5.000000000000004441, 0.000000000000000000 ) ) ;
#16104=CARTESIAN_POINT ( 'NONE',  ( 160.9801477675673311, -5.500000000000006217, -0.4574064797147053274 ) ) ;
#16105=CARTESIAN_POINT ( 'NONE',  ( 158.2500000000000284, -6.000000000000005329, 0.000000000000000000 ) ) ;
#16112=CARTESIAN_POINT ( 'NONE',  ( 155.9062500000000853, 6.000000000000005329, -2.485281374238555774 ) ) ;
#16113=VECTOR ( 'NONE', #22443, 1000.000000000000000 ) ;
#16115=VERTEX_POINT ( 'NONE', #3887 ) ;
#16131=FACE_OUTER_BOUND ( 'NONE', #23639, .T. ) ;
#16135=CARTESIAN_POINT ( 'NONE',  ( 161.9211002691896510, -4.999999999999989342, -2.071067811865468400 ) ) ;
#16136=CARTESIAN_POINT ( 'NONE',  ( 0.7548346512657310159, -15.52549481223858407, 8.075233279249948382 ) ) ;
#16141=DIRECTION ( 'NONE',  ( 0.000000000000000000, -1.000000000000000000, 0.000000000000000000 ) ) ;
#16143=CYLINDRICAL_SURFACE ( 'NONE', #11064, 0.5000000000000004441 ) ;
#16149=AXIS2_PLACEMENT_3D ( 'NONE', #12580, #11993, #26207 ) ;
#16150=CARTESIAN_POINT ( 'NONE',  ( 151.7812500000000284, 2.485281374238585972, 6.000000000000005329 ) ) ;
#16156=SURFACE_STYLE_USAGE ( .BOTH. , #25930 ) ;
#16159=CARTESIAN_POINT ( 'NONE',  ( 159.2683792240647165, -11.08218540272183716, 4.602811073450635782 ) ) ;
#16169=CARTESIAN_POINT ( 'NONE',  ( 157.9613248654052029, -5.500000000000005329, 0.000000000000000000 ) ) ;
#16178=CARTESIAN_POINT ( 'NONE',  ( 135.0000000000000568, -8.936994204536771846, -7.963449837756274796 ) ) ;
#16182=DIRECTION ( 'NONE',  ( 0.000000000000000000, -1.000000000000000000, 0.000000000000000000 ) ) ;
#16186=CARTESIAN_POINT ( 'NONE',  ( 150.8363248654052029, 0.000000000000000000, -5.500000000000005329 ) ) ;
#16193=CARTESIAN_POINT ( 'NONE',  ( 135.7500000000000284, -6.000000000000005329, 0.000000000000000000 ) ) ;
#16194=ORIENTED_EDGE ( 'NONE', *, *, #601, .F. ) ;
#16196=DIRECTION ( 'NONE',  ( 1.734723475976824844E-16, -1.000000000000000000, 0.000000000000000000 ) ) ;
#16197=CARTESIAN_POINT ( 'NONE',  ( 143.1636751345948255, 0.000000000000000000, 5.500000000000005329 ) ) ;
#16199=CARTESIAN_POINT ( 'NONE',  ( -39.00000000000000000, -20.00000000000021316, 4.000000000000003553 ) ) ;
#16203=CARTESIAN_POINT ( 'NONE',  ( 141.5476497308104058, 0.000000000000000000, -5.000000000000004441 ) ) ;
#16206=DIRECTION ( 'NONE',  ( -1.000000000000000000, -0.000000000000000000, -0.000000000000000000 ) ) ;
#16208=PRESENTATION_STYLE_ASSIGNMENT (( #1722 ) ) ;
#16213=DIRECTION ( 'NONE',  ( -1.000000000000000000, 0.000000000000000000, 0.000000000000000000 ) ) ;
#16215=EDGE_LOOP ( 'NONE', ( #4383, #1348, #20959, #7479 ) ) ;
#16222=CARTESIAN_POINT ( 'NONE',  ( 142.4062500000000284, 6.000000000000005329, -2.485281374238556218 ) ) ;
#16225=CARTESIAN_POINT ( 'NONE',  ( 142.4136751345948539, 0.000000000000000000, -5.500000000000005329 ) ) ;
#16226=CARTESIAN_POINT ( 'NONE',  ( 139.3125000000000284, 4.242640687119298093, -4.242640687119298093 ) ) ;
#16229=CIRCLE ( 'NONE', #26938, 1.000000000000000888 ) ;
#16231=AXIS2_PLACEMENT_3D ( 'NONE', #13028, #20058, #29403 ) ;
#16236=AXIS2_PLACEMENT_3D ( 'NONE', #27355, #2339, #21232 ) ;
#16244=CARTESIAN_POINT ( 'NONE',  ( 139.9574378273420336, -9.627775814265145726, -7.738041920342903168 ) ) ;
#16250=( NAMED_UNIT ( * ) SI_UNIT ( $, .STERADIAN. ) SOLID_ANGLE_UNIT ( ) );
#16253=CARTESIAN_POINT ( 'NONE',  ( 147.4836002691896795, 4.999999999999989342, -2.071067811865468400 ) ) ;
#16255=DIRECTION ( 'NONE',  ( -1.000000000000000000, 0.000000000000000000, 0.000000000000000000 ) ) ;
#16256=CARTESIAN_POINT ( 'NONE',  ( 155.6250000000000284, 0.000000000000000000, -6.000000000000005329 ) ) ;
#16263=ORIENTED_EDGE ( 'NONE', *, *, #7201, .F. ) ;
#16264=CARTESIAN_POINT ( 'NONE',  ( 158.8125000000000284, 4.242640687119298093, -4.242640687119298093 ) ) ;
#16267=EDGE_CURVE ( 'NONE', #22758, #13173, #23585, .T. ) ;
#16273=CIRCLE ( 'NONE', #26014, 12.00000000000000178 ) ;
#16277=( GEOMETRIC_REPRESENTATION_CONTEXT ( 3 ) GLOBAL_UNCERTAINTY_ASSIGNED_CONTEXT ( ( #24802 ) ) GLOBAL_UNIT_ASSIGNED_CONTEXT ( ( #30165, #6349, #20348 ) ) REPRESENTATION_CONTEXT ( 'NONE', 'WORKASPACE' ) );
#16281=FACE_OUTER_BOUND ( 'NONE', #16028, .T. ) ;
#16291=CARTESIAN_POINT ( 'NONE',  ( 160.8898502691896510, 3.535533905932725318, -3.535533905932725318 ) ) ;
#16292=CARTESIAN_POINT ( 'NONE',  ( 0.1148185598142369424, -15.24995533668263370, 8.589789778559206113 ) ) ;
#16293=EDGE_LOOP ( 'NONE', ( #20527, #10073, #13681, #29725 ) ) ;
#16297=CIRCLE ( 'NONE', #24557, 0.5000000000000004441 ) ;
#16299=CARTESIAN_POINT ( 'NONE',  ( 158.1636751345948255, 0.000000000000000000, 5.500000000000005329 ) ) ;
#16303=EDGE_CURVE ( 'NONE', #7661, #10410, #6876, .T. ) ;
#16307=CARTESIAN_POINT ( 'NONE',  ( 147.6562500000000284, -6.000000000000005329, 2.485281374238555774 ) ) ;
#16321=CARTESIAN_POINT ( 'NONE',  ( 158.1488248654052029, -3.889087296526011706, -3.889087296526011706 ) ) ;
#16325=DIRECTION ( 'NONE',  ( 0.7071067811865555663, 0.000000000000000000, -0.7071067811865394681 ) ) ;
#16328=CARTESIAN_POINT ( 'NONE',  ( 135.4618877836824424, -8.932258562185509732, -8.000000000000047962 ) ) ;
#16330=ORIENTED_EDGE ( 'NONE', *, *, #10649, .F. ) ;
#16333=ORIENTED_EDGE ( 'NONE', *, *, #24041, .T. ) ;
#16334=CIRCLE ( 'NONE', #20221, 30.00000000000000355 ) ;
#16343=VERTEX_POINT ( 'NONE', #9385 ) ;
#16345=CARTESIAN_POINT ( 'NONE',  ( 152.0550748654052313, -5.500000000000012434, -2.278174593052012309 ) ) ;
#16346=CARTESIAN_POINT ( 'NONE',  ( 133.4062500000000568, 6.000000000000005329, -2.485281374238555774 ) ) ;
#16347=( BOUNDED_CURVE ( )  B_SPLINE_CURVE ( 2, ( #15796, #15483, #5747, #20511, #8528, #10714, #15161, #17933, #24493 ),
 .UNSPECIFIED., .F., .T. ) 
 B_SPLINE_CURVE_WITH_KNOTS ( ( 3, 2, 2, 2, 3 ),
 ( 0.5875000000000001332, 0.5937499999999998890, 0.5999999999999996447, 0.6062499999999992895, 0.6124999999999991562 ),
 .UNSPECIFIED. ) 
 CURVE ( )  GEOMETRIC_REPRESENTATION_ITEM ( )  RATIONAL_B_SPLINE_CURVE ( ( 0.9999999999999986677, 0.9238795325112880708, 1.000000000000000000, 0.9238795325112867385, 1.000000000000000000, 0.9238795325112867385, 1.000000000000000000, 0.9238795325112975076, 0.9999999999999892308 ) ) 
 REPRESENTATION_ITEM ( '' )  );
#16352=CARTESIAN_POINT ( 'NONE',  ( 8.673617379884035472E-16, -14.26964382489354399, 8.429284772777599244 ) ) ;
#16354=CARTESIAN_POINT ( 'NONE',  ( 142.7663997308104058, -4.999999999999989342, -2.071067811865468400 ) ) ;
#16355=CARTESIAN_POINT ( 'NONE',  ( 136.0000000000000284, 0.000000000000000000, -12.00000000000000178 ) ) ;
#16357=CARTESIAN_POINT ( 'NONE',  ( 156.4761751345948255, 3.889087296526011706, 3.889087296526011706 ) ) ;
#16362=PLANE ( 'NONE',  #28732 ) ;
#16369=CARTESIAN_POINT ( 'NONE',  ( 140.4375000000000284, -4.242640687119298093, -4.242640687119298093 ) ) ;
#16373=CARTESIAN_POINT ( 'NONE',  ( 161.0476497308104342, 0.000000000000000000, -5.000000000000004441 ) ) ;
#16375=ORIENTED_EDGE ( 'NONE', *, *, #8945, .F. ) ;
#16385=DIRECTION ( 'NONE',  ( 1.000000000000000000, 0.000000000000000000, 0.000000000000000000 ) ) ;
#16387=LINE ( 'NONE', #2072, #7182 ) ;
#16393=CARTESIAN_POINT ( 'NONE',  ( 124.9999999999999432, -70.00000000000000000, 7.500000000000007105 ) ) ;
#16400=CARTESIAN_POINT ( 'NONE',  ( 150.2023502691896510, 0.000000000000000000, -5.000000000000004441 ) ) ;
#16403=AXIS2_PLACEMENT_3D ( 'NONE', #25904, #252, #16434 ) ;
#16404=CARTESIAN_POINT ( 'NONE',  ( 157.3125000000000284, 4.242640687119298093, -4.242640687119298093 ) ) ;
#16407=CARTESIAN_POINT ( 'NONE',  ( 139.1324251345948824, -5.500000000000012434, -2.278174593052012309 ) ) ;
#16408=DIRECTION ( 'NONE',  ( 1.000000000000000000, 0.000000000000000000, 0.000000000000000000 ) ) ;
#16413=CARTESIAN_POINT ( 'NONE',  ( 147.9375000000000284, -4.242640687119298093, -4.242640687119298093 ) ) ;
#16418=ORIENTED_EDGE ( 'NONE', *, *, #7034, .T. ) ;
#16420=B_SPLINE_CURVE_WITH_KNOTS ( 'NONE', 3,
 ( #30066, #21027, #2568, #11991, #18733, #8888, #18276, #27589, #3150, #26497 ),
 .UNSPECIFIED., .F., .F.,
 ( 4, 2, 2, 2, 4 ),
 ( 0.01514432977257332627, 0.01608480558703491436, 0.01702528140149650246, 0.01796575721595809055, 0.01890623303041967865 ),
 .UNSPECIFIED. ) ;
#16424=CARTESIAN_POINT ( 'NONE',  ( 154.8601497308104058, -3.535533905932725318, -3.535533905932725318 ) ) ;
#16429=CARTESIAN_POINT ( 'NONE',  ( 147.6488248654052029, -3.889087296526011706, -3.889087296526011706 ) ) ;
#16432=EDGE_CURVE ( 'NONE', #26506, #20437, #10028, .T. ) ;
#16434=DIRECTION ( 'NONE',  ( 0.000000000000000000, 0.000000000000000000, -1.000000000000000000 ) ) ;
#16438=CARTESIAN_POINT ( 'NONE',  ( 160.5148502691896510, -3.535533905932725318, -3.535533905932725318 ) ) ;
#16446=CARTESIAN_POINT ( 'NONE',  ( 157.4136751345948539, 0.000000000000000000, -5.500000000000005329 ) ) ;
#16449=DIRECTION ( 'NONE',  ( 0.000000000000000000, 0.000000000000000000, -1.000000000000000000 ) ) ;
#16451=ORIENTED_EDGE ( 'NONE', *, *, #2285, .F. ) ;
#16453=CARTESIAN_POINT ( 'NONE',  ( 153.2812500000000568, 2.485281374238585972, 6.000000000000005329 ) ) ;
#16459=DIRECTION ( 'NONE',  ( 0.000000000000000000, -0.000000000000000000, -1.000000000000000000 ) ) ;
#16462=CARTESIAN_POINT ( 'NONE',  ( -1.000000000000000888, -9.000000000000007105, 4.000000000000003553 ) ) ;
#16468=CARTESIAN_POINT ( 'NONE',  ( -0.3085845443850022130, -9.691415455614869501, -4.244941038143118739 ) ) ;
#16471=CARTESIAN_POINT ( 'NONE',  ( 138.8363248654052029, 0.000000000000000000, -5.500000000000005329 ) ) ;
#16473=CARTESIAN_POINT ( 'NONE',  ( 135.0000000000000284, -8.265636665782029269, -8.005364441812183429 ) ) ;
#16474=CARTESIAN_POINT ( 'NONE',  ( 153.8363248654052029, 0.000000000000000000, -5.500000000000005329 ) ) ;
#16475=ORIENTED_EDGE ( 'NONE', *, *, #29029, .T. ) ;
#16477=CARTESIAN_POINT ( 'NONE',  ( 0.9171503098353951389, -15.89765342390441916, 7.324020193813952417 ) ) ;
#16483=LINE ( 'NONE', #7372, #18280 ) ;
#16489=CARTESIAN_POINT ( 'NONE',  ( 140.4300748654052029, 2.278174593051702335, -5.500000000000323297 ) ) ;
#16490=ORIENTED_EDGE ( 'NONE', *, *, #22049, .T. ) ;
#16491=ORIENTED_EDGE ( 'NONE', *, *, #18783, .F. ) ;
#16493=CARTESIAN_POINT ( 'NONE',  ( 136.1250000000000284, 0.000000000000000000, -6.000000000000005329 ) ) ;
#16494=ORIENTED_EDGE ( 'NONE', *, *, #24516, .F. ) ;
#16500=CARTESIAN_POINT ( 'NONE',  ( 1.000000000000000888, -16.43939393939394833, 5.999693900976793337 ) ) ;
#16502=CARTESIAN_POINT ( 'NONE',  ( 147.0788997308104342, -4.999999999999989342, 2.071067811865468400 ) ) ;
#16505=DIRECTION ( 'NONE',  ( 1.000000000000000000, 0.000000000000000000, 0.000000000000000000 ) ) ;
#16506=CIRCLE ( 'NONE', #21856, 0.5000000000000000000 ) ;
#16512=SURFACE_STYLE_USAGE ( .BOTH. , #7093 ) ;
#16514=ORIENTED_EDGE ( 'NONE', *, *, #2046, .F. ) ;
#16523=CARTESIAN_POINT ( 'NONE',  ( 141.5625000000000284, -4.242640687119298093, 4.242640687119298093 ) ) ;
#16527=CARTESIAN_POINT ( 'NONE',  ( 159.5476497308104342, 0.000000000000000000, -5.000000000000004441 ) ) ;
#16530=ORIENTED_EDGE ( 'NONE', *, *, #3720, .T. ) ;
#16531=ORIENTED_EDGE ( 'NONE', *, *, #9815, .F. ) ;
#16534=CARTESIAN_POINT ( 'NONE',  ( 116.0000000000000142, 6.735557395310442023E-16, 5.500000000000000000 ) ) ;
#16536=CARTESIAN_POINT ( 'NONE',  ( 154.9761751345948255, 3.889087296526011706, 3.889087296526011706 ) ) ;
#16537=VECTOR ( 'NONE', #18102, 1000.000000000000000 ) ;
#16540=EDGE_CURVE ( 'NONE', #1653, #19367, #27491, .T. ) ;
#16543=AXIS2_PLACEMENT_3D ( 'NONE', #3282, #12708, #12859 ) ;
#16550=AXIS2_PLACEMENT_3D ( 'NONE', #22251, #22562, #11049 ) ;
#16554=CARTESIAN_POINT ( 'NONE',  ( 155.9062500000000568, 6.000000000000005329, -2.485281374238556218 ) ) ;
#16555=( NAMED_UNIT ( * ) SI_UNIT ( $, .STERADIAN. ) SOLID_ANGLE_UNIT ( ) );
#16557=CARTESIAN_POINT ( 'NONE',  ( 116.0000000000000142, 0.000000000000000000, 0.000000000000000000 ) ) ;
#16558=AXIS2_PLACEMENT_3D ( 'NONE', #14825, #3255, #5713 ) ;
#16561=CARTESIAN_POINT ( 'NONE',  ( 151.1250000000000284, 0.000000000000000000, -6.000000000000005329 ) ) ;
#16563=ORIENTED_EDGE ( 'NONE', *, *, #28029, .T. ) ;
#16570=CARTESIAN_POINT ( 'NONE',  ( 157.9538997308104058, -2.071067811865468400, -4.999999999999989342 ) ) ;
#16572=CARTESIAN_POINT ( 'NONE',  ( 159.1800748654052029, -2.278174593052116670, 5.499999999999908518 ) ) ;
#16574=AXIS2_PLACEMENT_3D ( 'NONE', #12096, #16408, #9302 ) ;
#16589=CIRCLE ( 'NONE', #29776, 0.5000000000000006661 ) ;
#16595=ORIENTED_EDGE ( 'NONE', *, *, #4699, .T. ) ;
#16600=ORIENTED_EDGE ( 'NONE', *, *, #25087, .F. ) ;
#16601=CARTESIAN_POINT ( 'NONE',  ( 150.0937500000000284, 6.000000000000005329, 2.485281374238585972 ) ) ;
#16603=EDGE_CURVE ( 'NONE', #20340, #22119, #7058, .T. ) ;
#16606=( BOUNDED_CURVE ( )  B_SPLINE_CURVE ( 2, ( #6369, #23299, #20990, #18693, #6988, #16407, #11170, #8694, #20518 ),
 .UNSPECIFIED., .F., .F. ) 
 B_SPLINE_CURVE_WITH_KNOTS ( ( 3, 2, 2, 2, 3 ),
 ( 0.2124999999999988010, 0.2187499999999990008, 0.2249999999999992006, 0.2312499999999994282, 0.2374999999999997391 ),
 .UNSPECIFIED. ) 
 CURVE ( )  GEOMETRIC_REPRESENTATION_ITEM ( )  RATIONAL_B_SPLINE_CURVE ( ( 1.000000000000014877, 0.9238795325112718615, 1.000000000000000000, 0.9238795325112867385, 1.000000000000000000, 0.9238795325112867385, 1.000000000000000000, 0.9238795325112904022, 0.9999999999999963363 ) ) 
 REPRESENTATION_ITEM ( '' )  );
#16608=ORIENTED_EDGE ( 'NONE', *, *, #17566, .F. ) ;
#16613=ORIENTED_EDGE ( 'NONE', *, *, #1051, .F. ) ;
#16614=( BOUNDED_SURFACE ( )  B_SPLINE_SURFACE ( 1, 2, ( 
 ( #25133, #6720, #2119, #30367, #18418, #18269, #21169, #16135, #18574, #27895, #18876, #111, #11522, #30059, #28198, #6868, #4098, #25441, #16291, #13521, #21018, #30214, #16438, #25763, #9493, #4709, #25611, #15980, #8882, #15834, #14142, #22861, #1798, #11204, #20550, #29902, #4564, #9029, #1960, #13830, #27581, #13990, #4251, #20864, #9177, #13673, #19317, #28639, #21472, #7173, #14711, #21314, #12277, #12420, #23913, #708, #26490, #19465, #26349, #21620, #14435, #23627, #257, #16733, #25909, #26200, #7610, #14285, #14566, #2560, #11984, #19032, #5298, #28349, #7325, #26057, #2702, #400, #19167, #28501, #16880, #5151, #15000, #24949, #24651, #3902, #20222, #22365, #3598, #7908, #22671, #29093, #13027, #29572, #17322, #8053, #6069, #8527, #26638, #17783, #26943, #12872, #5598, #24340, #17932, #8373, #10545, #22211, #27249, #15639, #15160, #26782, #24492, #19902, #1300, #3295, #1614, #12722, #10713, #3439, #3757, #19747, #29243, #8206, #17622, #20057, #15482, #11639, #13793, #30332, #27860, #20510, #16400, #6523, #18083, #13952, #25569, #13481, #20985, #25725, #1762, #11163, #27398, #6827, #15945, #22980, #22821, #4058, #9295, #25245, #8688, #6363, #25102, #4216, #2237, #4527, #11326, #20672, #30025, #18383, #16103, #16253, #2083, #25405, #11487, #24021, #16698, #2965, #364, #14827, #21581, #513, #19434, #16843, #24171, #26019, #12387, #9907, #28759, #19283, #11791, #14402, #14676, #23735, #28463, #21733, #69, #217, #26165, #9753, #12243, #5115, #26460, #5416, #7294, #672, #10058, #21132, #14535, #28163, #7133, #11951, #21277, #23875, #14249, #4824, #7575, #23587, #2524, #9603, #18993, #2820, #28604, #6302, #29949, #20300, #22021, #29646, #6156, #817, #7876, #17290, #16032, #3113, #20440, #19575, #8461, #11095, #24887, #8612, #18020, #12536, #27477, #22607, #6453, #6610, #22905, #13266, #22756, #24308, #20601, #14968, #18163, #15881, #29495, #1848, #27632, #11251, #25180, #20148, #13410, #21879, #10947, #957, #15572, #5565, #10213, #1697, #17868, #27337, #4144, #28910, #10358, #15724, #1542, #3988, #25033, #8928, #26610, #27185, #13567, #18319, #3257, #29799, #12688, #3838, #8776, #4305, #23065, #25330, #13724, #2006, #11415, #10295, #12188, #15061, #12775, #24108, #17228, #10449, #764, #2908, #10149, #17076, #21529, #19220, #28551, #26840, #14486, #898, #454, #19373, #21965, #5357, #19521, #28853, #23820, #7966, #3056, #17374, #17526, #3346, #12479, #3197, #5207, #1057, #26256, #28999, #26690, #9997, #22116 ),
 ( #9842, #12622, #24249, #14621, #19803, #609, #7519, #5653, #19660, #16930, #24405, #29148, #23971, #12328, #21674, #8106, #28695, #7667, #26405, #14765, #2760, #21818, #7812, #26553, #5499, #14909, #18131, #11063, #15851, #29459, #27446, #22420, #15383, #3956, #8583, #13088, #5802, #6417, #10768, #25151, #27155, #8896, #15692, #25002, #13535, #10921, #18287, #20116, #4113, #13382, #22875, #22725, #15218, #8431, #20408, #1358, #3500, #29769, #8746, #29308, #1815, #11221, #17677, #27000, #12930, #1668, #17838, #6125, #8263, #19955, #20569, #24708, #29919, #24550, #22267, #1196, #10602, #5963, #3652, #15540, #24858, #3806, #13235, #22579, #17987, #1509, #20272, #29618, #27303, #6272, #18586, #273, #7040, #16453, #4871, #2288, #9655, #2135, #9510, #25779, #14302, #4727, #27598, #11535, #2436, #20876, #4578, #125, #16000, #16150, #11693, #25630, #28064, #14004, #23642, #21331, #23190, #28217, #21185, #6577, #23346, #18897, #25300, #27754, #6731, #30383, #30075, #16601, #23493, #11382, #11848, #4271, #7191, #25924, #6881, #9351, #2575, #21038, #25456, #18743, #30230, #13692, #1975, #20726, #23031, #9044, #14156, #18434, #9193, #11997, #27906, #4422, #13850, #16307, #21926, #26365, #858, #1008, #7922, #5314, #24210, #9801, #15019, #413, #3159, #28961, #14578, #24361, #19046, #3309, #14446, #2867, #23780, #2714, #21779, #26211, #722, #21487, #12142, #12288, #10106, #1399, #18331, #8623, #29509, #13275, #3693, #29346, #29811, #11105, #10808, #27644, #17879, #8308, #25191, #6466, #24754, #22918, #6622, #13125, #22463, #17717, #18176, #27195, #24896, #20159, #15425, #1859, #8471, #16044, #11264, #25342, #4316, #13578, #15892, #20614, #3845, #29960, #6171, #15583, #8789, #4001, #22618, #1237, #8941, #1555, #13734, #10961, #10645, #20452, #27488, #19994, #6310, #27041, #20310, #6008, #4155, #29656, #18032, #27348, #15733, #25043, #13420, #22765, #1708, #11427, #11576, #7079, #21074, #23531, #9389, #311, #16789, #18626, #23679, #16642, #5055, #18782, #14339, #23079, #23234, #2175, #25819, #25502, #12033, #18939, #6774, #28257, #20772, #2615, #21374, #2330, #4767, #19082, #28104, #20922, #16493, #25666, #30119, #27798, #16193, #2019, #9083, #9547, #18478, #27947, #167, #14045, #14194, #2473, #4468, #25963, #11731, #4911, #26111, #9699, #4, #11889, #13894, #28404, #30271, #7234, #7382, #6921, #9233, #16346, #4615, #23383, #21225, #5356, #21528, #26255, #7811, #23970, #9841, #21817, #12478, #16929, #10148, #17227, #5206 ) ),
 .UNSPECIFIED., .F., .F., .T. ) 
 B_SPLINE_SURFACE_WITH_KNOTS ( ( 2, 2 ),
 ( 3, 2, 2, 2, 2, 2, 2, 2, 2, 2, 2, 2, 2, 2, 2, 2, 2, 2, 2, 2, 2, 2, 2, 2, 2, 2, 2, 2, 2, 2, 2, 2, 2, 2, 2, 2, 2, 2, 2, 2, 2, 2, 2, 2, 2, 2, 2, 2, 2, 2, 2, 2, 2, 2, 2, 2, 2, 2, 2, 2, 2, 2, 2, 2, 2, 2, 2, 2, 2, 2, 2, 2, 2, 2, 2, 2, 2, 2, 2, 2, 2, 2, 2, 2, 2, 2, 2, 2, 2, 2, 2, 2, 2, 2, 2, 2, 2, 2, 2, 2, 2, 2, 2, 2, 2, 2, 2, 2, 2, 2, 2, 2, 2, 2, 2, 2, 2, 2, 2, 2, 2, 2, 2, 2, 2, 2, 2, 2, 2, 2, 2, 2, 2, 2, 2, 2, 2, 2, 2, 2, 2, 2, 2, 2, 2, 2, 2, 2, 2, 2, 2, 2, 2, 2, 2, 2, 2, 2, 2, 2, 3 ),
 ( 0.000000000000000000, 1.000000000000000000 ),
 ( 0.000000000000000000, 0.006250000000000000347, 0.01250000000000000069, 0.01874999999999999931, 0.02500000000000000139, 0.03125000000000000000, 0.03749999999999999861, 0.04374999999999999722, 0.05000000000000000278, 0.05625000000000000139, 0.06250000000000000000, 0.06875000000000000555, 0.07499999999999999722, 0.08125000000000000278, 0.08749999999999999445, 0.09375000000000000000, 0.1000000000000000056, 0.1062499999999999972, 0.1125000000000000028, 0.1187499999999999944, 0.1250000000000000000, 0.1312500000000000056, 0.1375000000000000111, 0.1437499999999999889, 0.1499999999999999944, 0.1562500000000000000, 0.1625000000000000056, 0.1687500000000000111, 0.1749999999999999889, 0.1812499999999999944, 0.1875000000000000000, 0.1937500000000000056, 0.2000000000000000111, 0.2062499999999999889, 0.2124999999999999944, 0.2187500000000000000, 0.2250000000000000056, 0.2312500000000000111, 0.2374999999999999889, 0.2437499999999999944, 0.2500000000000000000, 0.2562499999999999778, 0.2625000000000000111, 0.2687499999999999889, 0.2750000000000000222, 0.2812500000000000000, 0.2874999999999999778, 0.2937500000000000111, 0.2999999999999999889, 0.3062500000000000222, 0.3125000000000000000, 0.3187499999999999778, 0.3250000000000000111, 0.3312499999999999889, 0.3375000000000000222, 0.3437500000000000000, 0.3499999999999999778, 0.3562500000000000111, 0.3624999999999999889, 0.3687500000000000222, 0.3750000000000000000, 0.3812499999999999778, 0.3875000000000000111, 0.3937499999999999889, 0.4000000000000000222, 0.4062500000000000000, 0.4124999999999999778, 0.4187500000000000111, 0.4249999999999999889, 0.4312500000000000222, 0.4375000000000000000, 0.4437499999999999778, 0.4500000000000000111, 0.4562499999999999889, 0.4625000000000000222, 0.4687500000000000000, 0.4749999999999999778, 0.4812500000000000111, 0.4874999999999999889, 0.4937500000000000222, 0.5000000000000000000, 0.5062499999999999778, 0.5124999999999999556, 0.5187500000000000444, 0.5250000000000000222, 0.5312500000000000000, 0.5374999999999999778, 0.5437499999999999556, 0.5500000000000000444, 0.5562500000000000222, 0.5625000000000000000, 0.5687499999999999778, 0.5749999999999999556, 0.5812500000000000444, 0.5875000000000000222, 0.5937500000000000000, 0.5999999999999999778, 0.6062499999999999556, 0.6125000000000000444, 0.6187500000000000222, 0.6250000000000000000, 0.6312499999999999778, 0.6374999999999999556, 0.6437500000000000444, 0.6500000000000000222, 0.6562500000000000000, 0.6624999999999999778, 0.6687499999999999556, 0.6750000000000000444, 0.6812500000000000222, 0.6875000000000000000, 0.6937499999999999778, 0.6999999999999999556, 0.7062500000000000444, 0.7125000000000000222, 0.7187500000000000000, 0.7249999999999999778, 0.7312499999999999556, 0.7375000000000000444, 0.7437500000000000222, 0.7500000000000000000, 0.7562499999999999778, 0.7624999999999999556, 0.7687500000000000444, 0.7750000000000000222, 0.7812500000000000000, 0.7874999999999999778, 0.7937499999999999556, 0.8000000000000000444, 0.8062500000000000222, 0.8125000000000000000, 0.8187499999999999778, 0.8249999999999999556, 0.8312500000000000444, 0.8375000000000000222, 0.8437500000000000000, 0.8499999999999999778, 0.8562499999999999556, 0.8625000000000000444, 0.8687500000000000222, 0.8750000000000000000, 0.8812499999999999778, 0.8874999999999999556, 0.8937500000000000444, 0.9000000000000000222, 0.9062500000000000000, 0.9124999999999999778, 0.9187499999999999556, 0.9250000000000000444, 0.9312500000000000222, 0.9375000000000000000, 0.9437499999999999778, 0.9499999999999999556, 0.9562500000000000444, 0.9625000000000000222, 0.9687500000000000000, 0.9749999999999999778, 0.9812499999999999556, 0.9875000000000000444, 0.9937500000000000222, 1.000000000000000000 ),
 .UNSPECIFIED. ) 
 GEOMETRIC_REPRESENTATION_ITEM ( )  RATIONAL_B_SPLINE_SURFACE ( (
 ( 1.000000000000000000, 0.9238795325112867385, 1.000000000000000000, 0.9238795325112867385, 1.000000000000000000, 0.9238795325112867385, 1.000000000000000000, 0.9238795325112867385, 1.000000000000000000, 0.9238795325112867385, 1.000000000000000000, 0.9238795325112867385, 1.000000000000000000, 0.9238795325112867385, 1.000000000000000000, 0.9238795325112867385, 1.000000000000000000, 0.9238795325112867385, 1.000000000000000000, 0.9238795325112867385, 1.000000000000000000, 0.9238795325112867385, 1.000000000000000000, 0.9238795325112867385, 1.000000000000000000, 0.9238795325112867385, 1.000000000000000000, 0.9238795325112867385, 1.000000000000000000, 0.9238795325112867385, 1.000000000000000000, 0.9238795325112867385, 1.000000000000000000, 0.9238795325112867385, 1.000000000000000000, 0.9238795325112867385, 1.000000000000000000, 0.9238795325112867385, 1.000000000000000000, 0.9238795325112867385, 1.000000000000000000, 0.9238795325112867385, 1.000000000000000000, 0.9238795325112867385, 1.000000000000000000, 0.9238795325112867385, 1.000000000000000000, 0.9238795325112867385, 1.000000000000000000, 0.9238795325112867385, 1.000000000000000000, 0.9238795325112867385, 1.000000000000000000, 0.9238795325112867385, 1.000000000000000000, 0.9238795325112867385, 1.000000000000000000, 0.9238795325112867385, 1.000000000000000000, 0.9238795325112867385, 1.000000000000000000, 0.9238795325112867385, 1.000000000000000000, 0.9238795325112867385, 1.000000000000000000, 0.9238795325112867385, 1.000000000000000000, 0.9238795325112867385, 1.000000000000000000, 0.9238795325112867385, 1.000000000000000000, 0.9238795325112867385, 1.000000000000000000, 0.9238795325112867385, 1.000000000000000000, 0.9238795325112867385, 1.000000000000000000, 0.9238795325112867385, 1.000000000000000000, 0.9238795325112867385, 1.000000000000000000, 0.9238795325112867385, 1.000000000000000000, 0.9238795325112867385, 1.000000000000000000, 0.9238795325112867385, 1.000000000000000000, 0.9238795325112867385, 1.000000000000000000, 0.9238795325112867385, 1.000000000000000000, 0.9238795325112867385, 1.000000000000000000, 0.9238795325112867385, 1.000000000000000000, 0.9238795325112867385, 1.000000000000000000, 0.9238795325112867385, 1.000000000000000000, 0.9238795325112867385, 1.000000000000000000, 0.9238795325112867385, 1.000000000000000000, 0.9238795325112867385, 1.000000000000000000, 0.9238795325112867385, 1.000000000000000000, 0.9238795325112867385, 1.000000000000000000, 0.9238795325112867385, 1.000000000000000000, 0.9238795325112867385, 1.000000000000000000, 0.9238795325112867385, 1.000000000000000000, 0.9238795325112867385, 1.000000000000000000, 0.9238795325112867385, 1.000000000000000000, 0.9238795325112867385, 1.000000000000000000, 0.9238795325112867385, 1.000000000000000000, 0.9238795325112867385, 1.000000000000000000, 0.9238795325112867385, 1.000000000000000000, 0.9238795325112867385, 1.000000000000000000, 0.9238795325112867385, 1.000000000000000000, 0.9238795325112867385, 1.000000000000000000, 0.9238795325112867385, 1.000000000000000000, 0.9238795325112867385, 1.000000000000000000, 0.9238795325112867385, 1.000000000000000000, 0.9238795325112867385, 1.000000000000000000, 0.9238795325112867385, 1.000000000000000000, 0.9238795325112867385, 1.000000000000000000, 0.9238795325112867385, 1.000000000000000000, 0.9238795325112867385, 1.000000000000000000, 0.9238795325112867385, 1.000000000000000000, 0.9238795325112867385, 1.000000000000000000, 0.9238795325112867385, 1.000000000000000000, 0.9238795325112867385, 1.000000000000000000, 0.9238795325112867385, 1.000000000000000000, 0.9238795325112867385, 1.000000000000000000, 0.9238795325112867385, 1.000000000000000000, 0.9238795325112867385, 1.000000000000000000, 0.9238795325112867385, 1.000000000000000000, 0.9238795325112867385, 1.000000000000000000, 0.9238795325112867385, 1.000000000000000000, 0.9238795325112867385, 1.000000000000000000, 0.9238795325112867385, 1.000000000000000000, 0.9238795325112867385, 1.000000000000000000, 0.9238795325112867385, 1.000000000000000000, 0.9238795325112867385, 1.000000000000000000, 0.9238795325112867385, 1.000000000000000000, 0.9238795325112867385, 1.000000000000000000, 0.9238795325112867385, 1.000000000000000000, 0.9238795325112867385, 1.000000000000000000, 0.9238795325112867385, 1.000000000000000000, 0.9238795325112867385, 1.000000000000000000, 0.9238795325112867385, 1.000000000000000000, 0.9238795325112867385, 1.000000000000000000, 0.9238795325112867385, 1.000000000000000000, 0.9238795325112867385, 1.000000000000000000, 0.9238795325112867385, 1.000000000000000000, 0.9238795325112867385, 1.000000000000000000, 0.9238795325112867385, 1.000000000000000000, 0.9238795325112867385, 1.000000000000000000, 0.9238795325112867385, 1.000000000000000000, 0.9238795325112867385, 1.000000000000000000, 0.9238795325112867385, 1.000000000000000000, 0.9238795325112867385, 1.000000000000000000, 0.9238795325112867385, 1.000000000000000000, 0.9238795325112867385, 1.000000000000000000, 0.9238795325112867385, 1.000000000000000000, 0.9238795325112867385, 1.000000000000000000, 0.9238795325112867385, 1.000000000000000000, 0.9238795325112867385, 1.000000000000000000, 0.9238795325112867385, 1.000000000000000000, 0.9238795325112867385, 1.000000000000000000, 0.9238795325112867385, 1.000000000000000000, 0.9238795325112867385, 1.000000000000000000, 0.9238795325112867385, 1.000000000000000000, 0.9238795325112867385, 1.000000000000000000, 0.9238795325112867385, 1.000000000000000000, 0.9238795325112867385, 1.000000000000000000, 0.9238795325112867385, 1.000000000000000000, 0.9238795325112867385, 1.000000000000000000, 0.9238795325112867385, 1.000000000000000000, 0.9238795325112867385, 1.000000000000000000, 0.9238795325112867385, 1.000000000000000000, 0.9238795325112867385, 1.000000000000000000, 0.9238795325112867385, 1.000000000000000000, 0.9238795325112867385, 1.000000000000000000, 0.9238795325112867385, 1.000000000000000000, 0.9238795325112867385, 1.000000000000000000, 0.9238795325112867385, 1.000000000000000000, 0.9238795325112867385, 1.000000000000000000, 0.9238795325112867385, 1.000000000000000000, 0.9238795325112867385, 1.000000000000000000, 0.9238795325112867385, 1.000000000000000000, 0.9238795325112867385, 1.000000000000000000, 0.9238795325112867385, 1.000000000000000000, 0.9238795325112867385, 1.000000000000000000, 0.9238795325112867385, 1.000000000000000000, 0.9238795325112867385, 1.000000000000000000, 0.9238795325112867385, 1.000000000000000000, 0.9238795325112867385, 1.000000000000000000, 0.9238795325112867385, 1.000000000000000000, 0.9238795325112867385, 1.000000000000000000, 0.9238795325112867385, 1.000000000000000000, 0.9238795325112867385, 1.000000000000000000, 0.9238795325112867385, 1.000000000000000000, 0.9238795325112867385, 1.000000000000000000, 0.9238795325112867385, 1.000000000000000000, 0.9238795325112867385, 1.000000000000000000, 0.9238795325112867385, 1.000000000000000000, 0.9238795325112867385, 1.000000000000000000, 0.9238795325112867385, 1.000000000000000000, 0.9238795325112867385, 1.000000000000000000, 0.9238795325112867385, 1.000000000000000000, 0.9238795325112867385, 1.000000000000000000, 0.9238795325112867385, 1.000000000000000000, 0.9238795325112867385, 1.000000000000000000),
 ( 1.000000000000000000, 0.9238795325112867385, 1.000000000000000000, 0.9238795325112867385, 1.000000000000000000, 0.9238795325112867385, 1.000000000000000000, 0.9238795325112867385, 1.000000000000000000, 0.9238795325112867385, 1.000000000000000000, 0.9238795325112867385, 1.000000000000000000, 0.9238795325112867385, 1.000000000000000000, 0.9238795325112867385, 1.000000000000000000, 0.9238795325112867385, 1.000000000000000000, 0.9238795325112867385, 1.000000000000000000, 0.9238795325112867385, 1.000000000000000000, 0.9238795325112867385, 1.000000000000000000, 0.9238795325112867385, 1.000000000000000000, 0.9238795325112867385, 1.000000000000000000, 0.9238795325112867385, 1.000000000000000000, 0.9238795325112867385, 1.000000000000000000, 0.9238795325112867385, 1.000000000000000000, 0.9238795325112867385, 1.000000000000000000, 0.9238795325112867385, 1.000000000000000000, 0.9238795325112867385, 1.000000000000000000, 0.9238795325112867385, 1.000000000000000000, 0.9238795325112867385, 1.000000000000000000, 0.9238795325112867385, 1.000000000000000000, 0.9238795325112867385, 1.000000000000000000, 0.9238795325112867385, 1.000000000000000000, 0.9238795325112867385, 1.000000000000000000, 0.9238795325112867385, 1.000000000000000000, 0.9238795325112867385, 1.000000000000000000, 0.9238795325112867385, 1.000000000000000000, 0.9238795325112867385, 1.000000000000000000, 0.9238795325112867385, 1.000000000000000000, 0.9238795325112867385, 1.000000000000000000, 0.9238795325112867385, 1.000000000000000000, 0.9238795325112867385, 1.000000000000000000, 0.9238795325112867385, 1.000000000000000000, 0.9238795325112867385, 1.000000000000000000, 0.9238795325112867385, 1.000000000000000000, 0.9238795325112867385, 1.000000000000000000, 0.9238795325112867385, 1.000000000000000000, 0.9238795325112867385, 1.000000000000000000, 0.9238795325112867385, 1.000000000000000000, 0.9238795325112867385, 1.000000000000000000, 0.9238795325112867385, 1.000000000000000000, 0.9238795325112867385, 1.000000000000000000, 0.9238795325112867385, 1.000000000000000000, 0.9238795325112867385, 1.000000000000000000, 0.9238795325112867385, 1.000000000000000000, 0.9238795325112867385, 1.000000000000000000, 0.9238795325112867385, 1.000000000000000000, 0.9238795325112867385, 1.000000000000000000, 0.9238795325112867385, 1.000000000000000000, 0.9238795325112867385, 1.000000000000000000, 0.9238795325112867385, 1.000000000000000000, 0.9238795325112867385, 1.000000000000000000, 0.9238795325112867385, 1.000000000000000000, 0.9238795325112867385, 1.000000000000000000, 0.9238795325112867385, 1.000000000000000000, 0.9238795325112867385, 1.000000000000000000, 0.9238795325112867385, 1.000000000000000000, 0.9238795325112867385, 1.000000000000000000, 0.9238795325112867385, 1.000000000000000000, 0.9238795325112867385, 1.000000000000000000, 0.9238795325112867385, 1.000000000000000000, 0.9238795325112867385, 1.000000000000000000, 0.9238795325112867385, 1.000000000000000000, 0.9238795325112867385, 1.000000000000000000, 0.9238795325112867385, 1.000000000000000000, 0.9238795325112867385, 1.000000000000000000, 0.9238795325112867385, 1.000000000000000000, 0.9238795325112867385, 1.000000000000000000, 0.9238795325112867385, 1.000000000000000000, 0.9238795325112867385, 1.000000000000000000, 0.9238795325112867385, 1.000000000000000000, 0.9238795325112867385, 1.000000000000000000, 0.9238795325112867385, 1.000000000000000000, 0.9238795325112867385, 1.000000000000000000, 0.9238795325112867385, 1.000000000000000000, 0.9238795325112867385, 1.000000000000000000, 0.9238795325112867385, 1.000000000000000000, 0.9238795325112867385, 1.000000000000000000, 0.9238795325112867385, 1.000000000000000000, 0.9238795325112867385, 1.000000000000000000, 0.9238795325112867385, 1.000000000000000000, 0.9238795325112867385, 1.000000000000000000, 0.9238795325112867385, 1.000000000000000000, 0.9238795325112867385, 1.000000000000000000, 0.9238795325112867385, 1.000000000000000000, 0.9238795325112867385, 1.000000000000000000, 0.9238795325112867385, 1.000000000000000000, 0.9238795325112867385, 1.000000000000000000, 0.9238795325112867385, 1.000000000000000000, 0.9238795325112867385, 1.000000000000000000, 0.9238795325112867385, 1.000000000000000000, 0.9238795325112867385, 1.000000000000000000, 0.9238795325112867385, 1.000000000000000000, 0.9238795325112867385, 1.000000000000000000, 0.9238795325112867385, 1.000000000000000000, 0.9238795325112867385, 1.000000000000000000, 0.9238795325112867385, 1.000000000000000000, 0.9238795325112867385, 1.000000000000000000, 0.9238795325112867385, 1.000000000000000000, 0.9238795325112867385, 1.000000000000000000, 0.9238795325112867385, 1.000000000000000000, 0.9238795325112867385, 1.000000000000000000, 0.9238795325112867385, 1.000000000000000000, 0.9238795325112867385, 1.000000000000000000, 0.9238795325112867385, 1.000000000000000000, 0.9238795325112867385, 1.000000000000000000, 0.9238795325112867385, 1.000000000000000000, 0.9238795325112867385, 1.000000000000000000, 0.9238795325112867385, 1.000000000000000000, 0.9238795325112867385, 1.000000000000000000, 0.9238795325112867385, 1.000000000000000000, 0.9238795325112867385, 1.000000000000000000, 0.9238795325112867385, 1.000000000000000000, 0.9238795325112867385, 1.000000000000000000, 0.9238795325112867385, 1.000000000000000000, 0.9238795325112867385, 1.000000000000000000, 0.9238795325112867385, 1.000000000000000000, 0.9238795325112867385, 1.000000000000000000, 0.9238795325112867385, 1.000000000000000000, 0.9238795325112867385, 1.000000000000000000, 0.9238795325112867385, 1.000000000000000000, 0.9238795325112867385, 1.000000000000000000, 0.9238795325112867385, 1.000000000000000000, 0.9238795325112867385, 1.000000000000000000, 0.9238795325112867385, 1.000000000000000000, 0.9238795325112867385, 1.000000000000000000, 0.9238795325112867385, 1.000000000000000000, 0.9238795325112867385, 1.000000000000000000, 0.9238795325112867385, 1.000000000000000000, 0.9238795325112867385, 1.000000000000000000, 0.9238795325112867385, 1.000000000000000000, 0.9238795325112867385, 1.000000000000000000, 0.9238795325112867385, 1.000000000000000000, 0.9238795325112867385, 1.000000000000000000, 0.9238795325112867385, 1.000000000000000000, 0.9238795325112867385, 1.000000000000000000, 0.9238795325112867385, 1.000000000000000000, 0.9238795325112867385, 1.000000000000000000, 0.9238795325112867385, 1.000000000000000000, 0.9238795325112867385, 1.000000000000000000, 0.9238795325112867385, 1.000000000000000000, 0.9238795325112867385, 1.000000000000000000, 0.9238795325112867385, 1.000000000000000000, 0.9238795325112867385, 1.000000000000000000, 0.9238795325112867385, 1.000000000000000000, 0.9238795325112867385, 1.000000000000000000, 0.9238795325112867385, 1.000000000000000000, 0.9238795325112867385, 1.000000000000000000, 0.9238795325112867385, 1.000000000000000000, 0.9238795325112867385, 1.000000000000000000, 0.9238795325112867385, 1.000000000000000000, 0.9238795325112867385, 1.000000000000000000, 0.9238795325112867385, 1.000000000000000000, 0.9238795325112867385, 1.000000000000000000, 0.9238795325112867385, 1.000000000000000000, 0.9238795325112867385, 1.000000000000000000, 0.9238795325112867385, 1.000000000000000000, 0.9238795325112867385, 1.000000000000000000) ) ) 
 REPRESENTATION_ITEM ( '' )  SURFACE ( )  );
#16620=CARTESIAN_POINT ( 'NONE',  ( -20.99999999999998224, -25.00000000000010658, -5.000000000000004441 ) ) ;
#16633=CIRCLE ( 'NONE', #7271, 12.00000000000000178 ) ;
#16636=ORIENTED_EDGE ( 'NONE', *, *, #1535, .T. ) ;
#16642=CARTESIAN_POINT ( 'NONE',  ( 138.0937500000000284, 6.000000000000005329, 2.485281374238585972 ) ) ;
#16643=ADVANCED_FACE ( 'NONE', ( #14707 ), #3942, .T. ) ;
#16645=FACE_OUTER_BOUND ( 'NONE', #25301, .T. ) ;
#16646=DIRECTION ( 'NONE',  ( 0.000000000000000000, 0.000000000000000000, -1.000000000000000000 ) ) ;
#16650=CARTESIAN_POINT ( 'NONE',  ( -0.04562205425659145164, -14.50000000000004619, 8.291335958003871909 ) ) ;
#16651=ADVANCED_FACE ( 'NONE', ( #16731 ), #23622, .F. ) ;
#16653=CARTESIAN_POINT ( 'NONE',  ( 146.2351497308104342, 3.535533905932725318, -3.535533905932725318 ) ) ;
#16669=CARTESIAN_POINT ( 'NONE',  ( 139.7812500000000284, 2.485281374238585972, 6.000000000000005329 ) ) ;
#16671=CARTESIAN_POINT ( 'NONE',  ( 138.2738248654052313, -3.889087296526011706, 3.889087296526011706 ) ) ;
#16672=CARTESIAN_POINT ( 'NONE',  ( 159.1726497308104058, -5.000000000000004441, 0.000000000000000000 ) ) ;
#16674=ADVANCED_FACE ( 'NONE', ( #26055 ), #397, .T. ) ;
#16679=TOROIDAL_SURFACE ( 'NONE', #10794, 29.00000000000000000, 1.000000000000000000 ) ;
#16681=DIRECTION ( 'NONE',  ( 1.000000000000000000, 0.000000000000000000, 0.000000000000000000 ) ) ;
#16684=CARTESIAN_POINT ( 'NONE',  ( 152.2574251345947971, -2.278174593051795149, 5.500000000000228262 ) ) ;
#16689=CARTESIAN_POINT ( 'NONE',  ( 140.2041261978397984, -9.046524830661697436, 7.884417203574004773 ) ) ;
#16691=DIRECTION ( 'NONE',  ( 1.000000000000000000, 6.938893903907221278E-15, 0.000000000000000000 ) ) ;
#16697=CARTESIAN_POINT ( 'NONE',  ( 139.8596287541092522, -9.431323395269577858, 7.852286093092132546 ) ) ;
#16698=CARTESIAN_POINT ( 'NONE',  ( 147.0148502691896510, -3.535533905932725318, -3.535533905932725318 ) ) ;
#16699=CARTESIAN_POINT ( 'NONE',  ( 161.0625000000000284, -4.242640687119298093, 4.242640687119298093 ) ) ;
#16701=( NAMED_UNIT ( * ) PLANE_ANGLE_UNIT ( ) SI_UNIT ( $, .RADIAN. ) );
#16702=CIRCLE ( 'NONE', #6358, 0.5000000000000004441 ) ;
#16707=CARTESIAN_POINT ( 'NONE',  ( 150.7500000000000284, -6.000000000000005329, 0.000000000000000000 ) ) ;
#16714=ORIENTED_EDGE ( 'NONE', *, *, #7414, .T. ) ;
#16717=ORIENTED_EDGE ( 'NONE', *, *, #6051, .F. ) ;
#16719=CARTESIAN_POINT ( 'NONE',  ( 154.2038997308104342, 2.071067811865468400, 4.999999999999989342 ) ) ;
#16724=CARTESIAN_POINT ( 'NONE',  ( 146.3363248654052029, 0.000000000000000000, -5.500000000000005329 ) ) ;
#16729=CARTESIAN_POINT ( 'NONE',  ( 141.0000000000000284, -12.00000000000001066, 4.000000000000003553 ) ) ;
#16731=FACE_OUTER_BOUND ( 'NONE', #5689, .T. ) ;
#16733=CARTESIAN_POINT ( 'NONE',  ( 156.6711002691896510, 4.999999999999989342, 2.071067811865468400 ) ) ;
#16736=UNCERTAINTY_MEASURE_WITH_UNIT (LENGTH_MEASURE( 1.000000000000000082E-05 ), #21866, 'distance_accuracy_value', 'NONE');
#16741=VERTEX_POINT ( 'NONE', #12126 ) ;
#16743=CARTESIAN_POINT ( 'NONE',  ( 140.1636751345948255, 0.000000000000000000, 5.500000000000005329 ) ) ;
#16752=UNCERTAINTY_MEASURE_WITH_UNIT (LENGTH_MEASURE( 1.000000000000000082E-05 ), #17509, 'distance_accuracy_value', 'NONE');
#16755=CARTESIAN_POINT ( 'NONE',  ( 158.7113248654052313, 5.500000000000005329, 0.000000000000000000 ) ) ;
#16759=CARTESIAN_POINT ( 'NONE',  ( 0.7576871283314742245, -15.57034058591134063, -7.988420828365927484 ) ) ;
#16761=DIRECTION ( 'NONE',  ( 0.000000000000000000, 0.000000000000000000, -1.000000000000000000 ) ) ;
#16766=CARTESIAN_POINT ( 'NONE',  ( 0.000000000000000000, 9.000000000000007105, 5.000000000000004441 ) ) ;
#16770=UNCERTAINTY_MEASURE_WITH_UNIT (LENGTH_MEASURE( 1.000000000000000082E-05 ), #4619, 'distance_accuracy_value', 'NONE');
#16776=ADVANCED_FACE ( 'NONE', ( #26780 ), #5899, .F. ) ;
#16782=EDGE_LOOP ( 'NONE', ( #13758, #3799, #25582, #20413 ) ) ;
#16783=DIRECTION ( 'NONE',  ( -1.734723475976824844E-16, 1.000000000000000000, -0.000000000000000000 ) ) ;
#16784=( BOUNDED_SURFACE ( )  B_SPLINE_SURFACE ( 3, 2, ( 
 ( #30166, #22965, #4204 ),
 ( #13619, #27997, #9130 ),
 ( #20661, #27846, #6815 ),
 ( #25553, #24158, #23721 ),
 ( #662, #12372, #12080 ),
 ( #7562, #19421, #18980 ),
 ( #24011, #2657, #350 ),
 ( #21266, #7718, #5257 ) ),
 .UNSPECIFIED., .F., .F., .F. ) 
 B_SPLINE_SURFACE_WITH_KNOTS ( ( 4, 2, 2, 4 ),
 ( 3, 3 ),
 ( 3.536383773289560661, 3.830385075063342804, 4.124386376837125390, 4.712388980384689674 ),
 ( 0.000000000000000000, 1.000000000000000000 ),
 .UNSPECIFIED. ) 
 GEOMETRIC_REPRESENTATION_ITEM ( )  RATIONAL_B_SPLINE_SURFACE ( (
 ( 1.000000000000000000, 0.7576044462920088485, 1.000000000000000000),
 ( 1.000000000000000000, 0.7805842023125117990, 1.000000000000000000),
 ( 1.000000000000000000, 0.8091552864627948871, 1.000000000000000000),
 ( 1.000000000000000000, 0.8665500556586516190, 1.000000000000000000),
 ( 1.000000000000000000, 0.8952806170300977584, 1.000000000000000000),
 ( 1.000000000000000000, 0.9690373989632083962, 1.000000000000000000),
 ( 1.000000000000000000, 1.000817594376246511, 1.000000000000000000),
 ( 1.000000000000000000, 1.000000000000000000, 1.000000000000000000) ) ) 
 REPRESENTATION_ITEM ( '' )  SURFACE ( )  );
#16787=ORIENTED_EDGE ( 'NONE', *, *, #12614, .F. ) ;
#16789=CARTESIAN_POINT ( 'NONE',  ( 138.3750000000000284, 0.000000000000000000, 6.000000000000005329 ) ) ;
#16794=VECTOR ( 'NONE', #24010, 1000.000000000000000 ) ;
#16795=CIRCLE ( 'NONE', #3487, 1.000000000000000000 ) ;
#16802=CARTESIAN_POINT ( 'NONE',  ( 135.8288997308104058, 4.999999999999989342, -2.071067811865468400 ) ) ;
#16808=CARTESIAN_POINT ( 'NONE',  ( 137.9136751345948539, 0.000000000000000000, -5.500000000000005329 ) ) ;
#16809=ORIENTED_EDGE ( 'NONE', *, *, #24839, .T. ) ;
#16810=ADVANCED_FACE ( 'NONE', ( #5745 ), #26487, .F. ) ;
#16818=ADVANCED_FACE ( 'NONE', ( #15327 ), #24338, .T. ) ;
#16819=CARTESIAN_POINT ( 'NONE',  ( 134.3437500000000568, -6.000000000000005329, -2.485281374238555774 ) ) ;
#16823=VERTEX_POINT ( 'NONE', #1143 ) ;
#16827=CARTESIAN_POINT ( 'NONE',  ( 116.0000000000000142, 6.735557395310442023E-16, 5.500000000000000000 ) ) ;
#16832=DIRECTION ( 'NONE',  ( 0.000000000000000000, 0.000000000000000000, -1.000000000000000000 ) ) ;
#16842=( LENGTH_UNIT ( ) NAMED_UNIT ( * ) SI_UNIT ( .MILLI., .METRE. ) );
#16843=CARTESIAN_POINT ( 'NONE',  ( 146.3586002691896510, 2.071067811865468400, 4.999999999999989342 ) ) ;
#16844=CARTESIAN_POINT ( 'NONE',  ( 150.8437500000000284, -6.000000000000005329, -2.485281374238556218 ) ) ;
#16850=CARTESIAN_POINT ( 'NONE',  ( 150.0000000000000284, 6.000000000000005329, 0.000000000000000000 ) ) ;
#16852=CARTESIAN_POINT ( 'NONE',  ( 153.8363248654052029, 0.000000000000000000, -5.500000000000005329 ) ) ;
#16853=UNCERTAINTY_MEASURE_WITH_UNIT (LENGTH_MEASURE( 1.000000000000000082E-05 ), #16924, 'distance_accuracy_value', 'NONE');
#16855=( GEOMETRIC_REPRESENTATION_CONTEXT ( 3 ) GLOBAL_UNCERTAINTY_ASSIGNED_CONTEXT ( ( #5036 ) ) GLOBAL_UNIT_ASSIGNED_CONTEXT ( ( #25270, #18105, #8716 ) ) REPRESENTATION_CONTEXT ( 'NONE', 'WORKASPACE' ) );
#16863=SURFACE_STYLE_FILL_AREA ( #27765 ) ;
#16864=DIRECTION ( 'NONE',  ( -0.000000000000000000, -0.000000000000000000, -1.000000000000000000 ) ) ;
#16867=CARTESIAN_POINT ( 'NONE',  ( 140.0256844536734206, -11.04862469602420916, 4.684420475250495208 ) ) ;
#16871=CARTESIAN_POINT ( 'NONE',  ( 161.0000000000000284, 3.467572205841706889, 4.269185284954735593 ) ) ;
#16880=CARTESIAN_POINT ( 'NONE',  ( 155.0773502691896510, 5.000000000000004441, 0.000000000000000000 ) ) ;
#16885=DIRECTION ( 'NONE',  ( 0.000000000000000000, 0.000000000000000000, -1.000000000000000000 ) ) ;
#16887=ORIENTED_EDGE ( 'NONE', *, *, #14049, .T. ) ;
#16889=CARTESIAN_POINT ( 'NONE',  ( 135.0000000000000284, -9.165151389911669000, -8.500000000000007105 ) ) ;
#16892=EDGE_LOOP ( 'NONE', ( #13502, #12835, #18328, #25960 ) ) ;
#16900=CARTESIAN_POINT ( 'NONE',  ( 136.0000000000000284, 0.000000000000000000, 0.000000000000000000 ) ) ;
#16901=ORIENTED_EDGE ( 'NONE', *, *, #25044, .T. ) ;
#16902=CARTESIAN_POINT ( 'NONE',  ( -0.08066462393745461867, -15.01489640285979910, -8.018075067159342595 ) ) ;
#16904=CARTESIAN_POINT ( 'NONE',  ( -4.999999999999886313, -69.50000000000001421, -8.000000000000007105 ) ) ;
#16907=CYLINDRICAL_SURFACE ( 'NONE', #7834, 17.50000000000000355 ) ;
#16909=CARTESIAN_POINT ( 'NONE',  ( 13.99999999999999822, 2.020667218593133494E-15, 16.50000000000000355 ) ) ;
#16911=DIRECTION ( 'NONE',  ( 0.000000000000000000, 0.000000000000000000, -1.000000000000000000 ) ) ;
#16915=DIRECTION ( 'NONE',  ( 0.000000000000000000, 0.000000000000000000, -1.000000000000000000 ) ) ;
#16916=ORIENTED_EDGE ( 'NONE', *, *, #4031, .F. ) ;
#16919=CARTESIAN_POINT ( 'NONE',  ( 1.000000004086045946, -16.31569083567854150, 6.338645202004363988 ) ) ;
#16924=( LENGTH_UNIT ( ) NAMED_UNIT ( * ) SI_UNIT ( .MILLI., .METRE. ) );
#16929=CARTESIAN_POINT ( 'NONE',  ( 132.2812500000000000, 2.485281374238585972, 6.000000000000005329 ) ) ;
#16930=CARTESIAN_POINT ( 'NONE',  ( 161.1562500000000284, -6.000000000000005329, 2.485281374238555774 ) ) ;
#16931=ORIENTED_EDGE ( 'NONE', *, *, #11372, .F. ) ;
#16940=CARTESIAN_POINT ( 'NONE',  ( 138.6413997308104342, 2.071067811865468400, -4.999999999999989342 ) ) ;
#16943=CARTESIAN_POINT ( 'NONE',  ( 1.000000000000000888, 0.000000000000000000, 17.50000000000000355 ) ) ;
#16946=EDGE_CURVE ( 'NONE', #22830, #26206, #3168, .T. ) ;
#16948=DIRECTION ( 'NONE',  ( 1.000000000000000000, 0.000000000000000000, 0.000000000000000000 ) ) ;
#16949=CARTESIAN_POINT ( 'NONE',  ( 154.0386751345948539, -5.500000000000005329, 0.000000000000000000 ) ) ;
#16955=VERTEX_POINT ( 'NONE', #6520 ) ;
#16957=CARTESIAN_POINT ( 'NONE',  ( 135.5625000000000284, -4.242640687119298093, 4.242640687119298093 ) ) ;
#16962=AXIS2_PLACEMENT_3D ( 'NONE', #21330, #18740, #25922 ) ;
#16963=CARTESIAN_POINT ( 'NONE',  ( 140.5384615384615756, -11.07692307692308908, 4.615384615384614975 ) ) ;
#16966=EDGE_CURVE ( 'NONE', #6311, #278, #12069, .T. ) ;
#16967=ORIENTED_EDGE ( 'NONE', *, *, #1470, .T. ) ;
#16968=B_SPLINE_CURVE_WITH_KNOTS ( 'NONE', 3,
 ( #15212, #5797, #22719, #10598 ),
 .UNSPECIFIED., .F., .F.,
 ( 4, 4 ),
 ( 1.734723475976789761E-18, 0.0005141325497624451386 ),
 .UNSPECIFIED. ) ;
#16970=AXIS2_PLACEMENT_3D ( 'NONE', #14718, #28646, #5157 ) ;
#16986=DIRECTION ( 'NONE',  ( 0.000000000000000000, 0.000000000000000000, -1.000000000000000000 ) ) ;
#16989=CARTESIAN_POINT ( 'NONE',  ( 154.7812500000000568, 2.485281374238585972, 6.000000000000005329 ) ) ;
#16990=CARTESIAN_POINT ( 'NONE',  ( 135.0000000000000000, -7.800730961597594160, -7.983509344454088108 ) ) ;
#16996=CARTESIAN_POINT ( 'NONE',  ( 149.2500000000000284, -6.000000000000005329, 0.000000000000000000 ) ) ;
#17002=VECTOR ( 'NONE', #18253, 1000.000000000000000 ) ;
#17004=ADVANCED_FACE ( 'NONE', ( #22817 ), #1916, .T. ) ;
#17009=CARTESIAN_POINT ( 'NONE',  ( 140.0000000000000284, -11.45643923738959202, 5.000000000000004441 ) ) ;
#17013=CARTESIAN_POINT ( 'NONE',  ( 143.5238248654052029, 3.889087296526011706, -3.889087296526011706 ) ) ;
#17019=CARTESIAN_POINT ( 'NONE',  ( -10.00000000000000178, -19.99999999999998934, 4.000000000000003553 ) ) ;
#17026=CARTESIAN_POINT ( 'NONE',  ( -4.999999999999886313, -70.00000000000001421, -7.500000000000007105 ) ) ;
#17031=MECHANICAL_DESIGN_GEOMETRIC_PRESENTATION_REPRESENTATION('',(#8174),#14152);
#17033=ADVANCED_FACE ( 'NONE', ( #8992 ), #4055, .F. ) ;
#17035=VECTOR ( 'NONE', #13917, 1000.000000000000000 ) ;
#17037=( BOUNDED_CURVE ( )  B_SPLINE_CURVE ( 2, ( #8423, #15532, #26831, #19948, #3800, #24543, #15050, #3494, #29142 ),
 .UNSPECIFIED., .F., .T. ) 
 B_SPLINE_CURVE_WITH_KNOTS ( ( 3, 2, 2, 2, 3 ),
 ( 0.7375000000000002665, 0.7437500000000004663, 0.7500000000000006661, 0.7562500000000009770, 0.7625000000000011768 ),
 .UNSPECIFIED. ) 
 CURVE ( )  GEOMETRIC_REPRESENTATION_ITEM ( )  RATIONAL_B_SPLINE_CURVE ( ( 0.9999999999999973355, 0.9238795325112894030, 1.000000000000000000, 0.9238795325112867385, 1.000000000000000000, 0.9238795325112867385, 1.000000000000000000, 0.9238795325112718615, 1.000000000000014877 ) ) 
 REPRESENTATION_ITEM ( '' )  );
#17049=FACE_OUTER_BOUND ( 'NONE', #2740, .T. ) ;
#17050=VECTOR ( 'NONE', #26030, 1000.000000000000000 ) ;
#17056=PRESENTATION_STYLE_ASSIGNMENT (( #14466 ) ) ;
#17058=SURFACE_STYLE_FILL_AREA ( #7649 ) ;
#17064=CARTESIAN_POINT ( 'NONE',  ( 0.1286836220987009893, -16.20672030812517761, 6.611306774490117277 ) ) ;
#17069=DIRECTION ( 'NONE',  ( 0.000000000000000000, 0.000000000000000000, -1.000000000000000000 ) ) ;
#17070=EDGE_LOOP ( 'NONE', ( #28998, #6691, #8828, #26995, #1679, #10779 ) ) ;
#17072=CIRCLE ( 'NONE', #28326, 1.000000000000000888 ) ;
#17074=EDGE_LOOP ( 'NONE', ( #7819, #8581, #25326, #1481 ) ) ;
#17076=CARTESIAN_POINT ( 'NONE',  ( 135.1086002691896795, -2.071067811865468400, -4.999999999999989342 ) ) ;
#17081=( NAMED_UNIT ( * ) SI_UNIT ( $, .STERADIAN. ) SOLID_ANGLE_UNIT ( ) );
#17084=ORIENTED_EDGE ( 'NONE', *, *, #7409, .F. ) ;
#17085=VECTOR ( 'NONE', #29761, 1000.000000000000000 ) ;
#17087=CARTESIAN_POINT ( 'NONE',  ( -0.004400386472629622125, -15.41927558935930875, -6.289782602405238343 ) ) ;
#17088=CARTESIAN_POINT ( 'NONE',  ( 149.7261751345948539, -3.889087296526011706, -3.889087296526011706 ) ) ;
#17089=CARTESIAN_POINT ( 'NONE',  ( 137.6101497308104342, 3.535533905932725318, 3.535533905932725318 ) ) ;
#17092=LINE ( 'NONE', #21833, #20943 ) ;
#17102=ORIENTED_EDGE ( 'NONE', *, *, #7638, .T. ) ;
#17104=AXIS2_PLACEMENT_3D ( 'NONE', #23099, #30142, #6645 ) ;
#17115=ORIENTED_EDGE ( 'NONE', *, *, #27984, .T. ) ;
#17118=B_SPLINE_CURVE_WITH_KNOTS ( 'NONE', 3,
 ( #29425, #3617, #24675, #8395, #19629, #13052, #1323, #24219, #7932, #28816, #3024, #24514 ),
 .UNSPECIFIED., .F., .F.,
 ( 4, 2, 2, 2, 2, 4 ),
 ( 0.000000000000000000, 0.0005856679266213420500, 0.001171335853242684100, 0.001757003779864027343, 0.002049837743174697663, 0.002342671706485368634 ),
 .UNSPECIFIED. ) ;
#17119=DIRECTION ( 'NONE',  ( 0.000000000000000000, 0.000000000000000000, 1.000000000000000000 ) ) ;
#17120=SURFACE_STYLE_USAGE ( .BOTH. , #30353 ) ;
#17124=CARTESIAN_POINT ( 'NONE',  ( -19.99999999999998224, -25.00000000000010658, 7.500000000000007105 ) ) ;
#17129=CARTESIAN_POINT ( 'NONE',  ( 139.8284140731593652, -9.384860798393967585, 7.878476001700652098 ) ) ;
#17131=CARTESIAN_POINT ( 'NONE',  ( 139.5074251345948255, 2.278174593051927044, -5.500000000000096811 ) ) ;
#17136=CARTESIAN_POINT ( 'NONE',  ( 153.2812500000000000, 2.485281374238585972, 6.000000000000005329 ) ) ;
#17137=CARTESIAN_POINT ( 'NONE',  ( 135.0000000000000568, -7.637934915400436786, -8.088409639717225375 ) ) ;
#17142=ORIENTED_EDGE ( 'NONE', *, *, #6959, .F. ) ;
#17143=CARTESIAN_POINT ( 'NONE',  ( 142.7812500000000568, 2.485281374238585972, 6.000000000000005329 ) ) ;
#17145=CARTESIAN_POINT ( 'NONE',  ( 135.0863248654052313, 0.000000000000000000, 5.500000000000005329 ) ) ;
#17146=EDGE_CURVE ( 'NONE', #18703, #5354, #16633, .T. ) ;
#17150=ORIENTED_EDGE ( 'NONE', *, *, #9715, .F. ) ;
#17156=FACE_OUTER_BOUND ( 'NONE', #26537, .T. ) ;
#17158=CARTESIAN_POINT ( 'NONE',  ( 140.5000000328705028, -11.02580175850465238, 4.736714422037595185 ) ) ;
#17162=DIRECTION ( 'NONE',  ( 1.000000000000000000, 0.000000000000000000, 0.000000000000000000 ) ) ;
#17163=VECTOR ( 'NONE', #9737, 1000.000000000000000 ) ;
#17165=CARTESIAN_POINT ( 'NONE',  ( 142.3988248654052313, 3.889087296526011706, 3.889087296526011706 ) ) ;
#17170=MECHANICAL_DESIGN_GEOMETRIC_PRESENTATION_REPRESENTATION('',(#9330),#6863);
#17174=CARTESIAN_POINT ( 'NONE',  ( -9.999999999999772626, -89.00000000000001421, 3.000000000000002665 ) ) ;
#17177=SURFACE_STYLE_USAGE ( .BOTH. , #15012 ) ;
#17179=CARTESIAN_POINT ( 'NONE',  ( 145.7886751345948539, 5.500000000000005329, 0.000000000000000000 ) ) ;
#17181=AXIS2_PLACEMENT_3D ( 'NONE', #22485, #3864, #15756 ) ;
#17185=ORIENTED_EDGE ( 'NONE', *, *, #12104, .F. ) ;
#17188=VECTOR ( 'NONE', #872, 1000.000000000000000 ) ;
#17194=CARTESIAN_POINT ( 'NONE',  ( 125.0000000000000568, -55.00000000000000711, 7.500000000000007105 ) ) ;
#17197=ORIENTED_EDGE ( 'NONE', *, *, #5614, .T. ) ;
#17198=CARTESIAN_POINT ( 'NONE',  ( -0.05026617339078452013, -14.53485816245738960, -8.281223121639204265 ) ) ;
#17199=CARTESIAN_POINT ( 'NONE',  ( 158.9136751345948539, 0.000000000000000000, -5.500000000000005329 ) ) ;
#17211=DIRECTION ( 'NONE',  ( 0.000000000000000000, 1.000000000000000000, -0.000000000000000000 ) ) ;
#17215=VERTEX_POINT ( 'NONE', #25176 ) ;
#17216=DIRECTION ( 'NONE',  ( 0.000000000000000000, -1.000000000000000000, 0.000000000000000000 ) ) ;
#17217=CARTESIAN_POINT ( 'NONE',  ( -1.000000000000000888, 11.00000000000001066, 3.000000000000002665 ) ) ;
#17218=AXIS2_PLACEMENT_3D ( 'NONE', #10468, #13109, #24880 ) ;
#17222=EDGE_CURVE ( 'NONE', #15499, #7376, #12222, .T. ) ;
#17227=CARTESIAN_POINT ( 'NONE',  ( 132.0937500000000568, 6.000000000000005329, 2.485281374238585972 ) ) ;
#17228=CARTESIAN_POINT ( 'NONE',  ( 135.5773502691896510, 5.000000000000004441, 0.000000000000000000 ) ) ;
#17233=ORIENTED_EDGE ( 'NONE', *, *, #15384, .F. ) ;
#17235=CARTESIAN_POINT ( 'NONE',  ( 125.0000000000000568, -55.00000000000000711, -8.000000000000007105 ) ) ;
#17236=DIRECTION ( 'NONE',  ( 1.000000000000000000, 0.000000000000000000, 0.000000000000000000 ) ) ;
#17238=STYLED_ITEM ( 'NONE', ( #26636 ), #16776 ) ;
#17239=CARTESIAN_POINT ( 'NONE',  ( 140.1413997308104058, 2.071067811865468400, -4.999999999999989342 ) ) ;
#17245=DIRECTION ( 'NONE',  ( 1.000000000000000000, -3.469446951953694061E-16, 0.000000000000000000 ) ) ;
#17248=VERTEX_POINT ( 'NONE', #1082 ) ;
#17249=EDGE_CURVE ( 'NONE', #25966, #5920, #10473, .T. ) ;
#17251=CARTESIAN_POINT ( 'NONE',  ( -9.999999999999980460, -60.00000000000001421, 4.000000000000003553 ) ) ;
#17257=CARTESIAN_POINT ( 'NONE',  ( 135.4687500000000853, -2.485281374238585972, 6.000000000000005329 ) ) ;
#17259=CIRCLE ( 'NONE', #26062, 0.5000000000000004441 ) ;
#17261=CARTESIAN_POINT ( 'NONE',  ( 162.0000000000000284, 1.408343819019456176E-15, 11.00000000000000355 ) ) ;
#17265=ORIENTED_EDGE ( 'NONE', *, *, #25113, .T. ) ;
#17266=ORIENTED_EDGE ( 'NONE', *, *, #20481, .T. ) ;
#17274=CARTESIAN_POINT ( 'NONE',  ( 153.5476497308104342, 0.000000000000000000, -5.000000000000004441 ) ) ;
#17277=CARTESIAN_POINT ( 'NONE',  ( 116.0000000000000142, 0.000000000000000000, 0.000000000000000000 ) ) ;
#17278=CIRCLE ( 'NONE', #10898, 15.99999999999998579 ) ;
#17284=CARTESIAN_POINT ( 'NONE',  ( -4.999999999999886313, -10.00000000000000888, -7.500000000000007105 ) ) ;
#17288=CARTESIAN_POINT ( 'NONE',  ( -10.00000000000000178, 9.000000000000007105, 3.000000000000002665 ) ) ;
#17289=ORIENTED_EDGE ( 'NONE', *, *, #21777, .T. ) ;
#17290=CARTESIAN_POINT ( 'NONE',  ( 141.8586002691896510, 2.071067811865468400, 4.999999999999989342 ) ) ;
#17291=CARTESIAN_POINT ( 'NONE',  ( 152.7187500000000284, 2.485281374238556218, -6.000000000000005329 ) ) ;
#17294=CARTESIAN_POINT ( 'NONE',  ( 157.5863248654052597, 0.000000000000000000, 5.500000000000005329 ) ) ;
#17295=CARTESIAN_POINT ( 'NONE',  ( 145.9687500000000568, -2.485281374238585972, 6.000000000000005329 ) ) ;
#17296=CARTESIAN_POINT ( 'NONE',  ( 143.3363248654052029, 0.000000000000000000, -5.500000000000005329 ) ) ;
#17299=CARTESIAN_POINT ( 'NONE',  ( -0.5000000000000004441, -10.00000000000000888, 5.000000000000004441 ) ) ;
#17303=( LENGTH_UNIT ( ) NAMED_UNIT ( * ) SI_UNIT ( .MILLI., .METRE. ) );
#17306=( BOUNDED_CURVE ( )  B_SPLINE_CURVE ( 2, ( #19780, #30018, #23132, #24384, #26671, #5631, #15037, #8088, #17502 ),
 .UNSPECIFIED., .F., .T. ) 
 B_SPLINE_CURVE_WITH_KNOTS ( ( 3, 2, 2, 2, 3 ),
 ( 0.2125000000000006883, 0.2187500000000004441, 0.2250000000000002276, 0.2312500000000000111, 0.2374999999999997391 ),
 .UNSPECIFIED. ) 
 CURVE ( )  GEOMETRIC_REPRESENTATION_ITEM ( )  RATIONAL_B_SPLINE_CURVE ( ( 0.9999999999999915623, 0.9238795325112951762, 1.000000000000000000, 0.9238795325112867385, 1.000000000000000000, 0.9238795325112867385, 1.000000000000000000, 0.9238795325112897361, 0.9999999999999970024 ) ) 
 REPRESENTATION_ITEM ( '' )  );
#17310=EDGE_CURVE ( 'NONE', #15465, #17671, #29500, .T. ) ;
#17312=DIRECTION ( 'NONE',  ( 1.000000000000000000, 0.000000000000000000, 0.000000000000000000 ) ) ;
#17317=CARTESIAN_POINT ( 'NONE',  ( 134.9999999999999147, 5.939731808376970790, 0.5826989768619842414 ) ) ;
#17322=CARTESIAN_POINT ( 'NONE',  ( 153.7648502691896510, 3.535533905932725318, 3.535533905932752852 ) ) ;
#17324=CARTESIAN_POINT ( 'NONE',  ( 151.8824251345948255, 5.500000000000012434, 2.278174593052012309 ) ) ;
#17327=DIRECTION ( 'NONE',  ( 1.000000000000000000, 0.000000000000000000, 0.000000000000000000 ) ) ;
#17329=ORIENTED_EDGE ( 'NONE', *, *, #3831, .F. ) ;
#17330=CARTESIAN_POINT ( 'NONE',  ( 159.5625000000000284, -4.242640687119298093, 4.242640687119298093 ) ) ;
#17344=CARTESIAN_POINT ( 'NONE',  ( 147.1949251345948539, 5.500000000000012434, -2.278174593052012309 ) ) ;
#17347=ORIENTED_EDGE ( 'NONE', *, *, #11296, .F. ) ;
#17351=DIRECTION ( 'NONE',  ( 1.000000000000000000, 0.000000000000000000, 0.000000000000000000 ) ) ;
#17358=CARTESIAN_POINT ( 'NONE',  ( 135.0124371858787526, -7.358334781654392920, 8.428837531783013759 ) ) ;
#17363=EDGE_CURVE ( 'NONE', #11174, #8510, #20005, .T. ) ;
#17366=CARTESIAN_POINT ( 'NONE',  ( 135.1659834729329930, -8.213724325835228157, -8.175323444973551901 ) ) ;
#17370=ORIENTED_EDGE ( 'NONE', *, *, #29691, .F. ) ;
#17372=VERTEX_POINT ( 'NONE', #27480 ) ;
#17374=CARTESIAN_POINT ( 'NONE',  ( 133.6086002691896510, -2.071067811865468400, -4.999999999999989342 ) ) ;
#17377=( NAMED_UNIT ( * ) SI_UNIT ( $, .STERADIAN. ) SOLID_ANGLE_UNIT ( ) );
#17378=CARTESIAN_POINT ( 'NONE',  ( 136.0000000000000284, -9.165151389911695645, -8.000000000000007105 ) ) ;
#17379=FACE_OUTER_BOUND ( 'NONE', #10472, .T. ) ;
#17383=CARTESIAN_POINT ( 'NONE',  ( 15.00000000000000000, 2.081899558550500674E-15, 16.50000000000000355 ) ) ;
#17384=CARTESIAN_POINT ( 'NONE',  ( 135.0788997308104342, -4.999999999999989342, 2.071067811865468400 ) ) ;
#17389=DIRECTION ( 'NONE',  ( 0.000000000000000000, 0.000000000000000000, -1.000000000000000000 ) ) ;
#17401=CARTESIAN_POINT ( 'NONE',  ( 1.000000000000000888, -16.43939393939394833, 5.999693900976793337 ) ) ;
#17403=CARTESIAN_POINT ( 'NONE',  ( 162.0000000000000284, 0.000000000000000000, -6.499999999999977796 ) ) ;
#17404=ORIENTED_EDGE ( 'NONE', *, *, #22224, .F. ) ;
#17411=DIRECTION ( 'NONE',  ( 0.000000000000000000, 0.000000000000000000, 1.000000000000000000 ) ) ;
#17412=CARTESIAN_POINT ( 'NONE',  ( 140.1656963055991127, -11.58284815279920110, 4.440052304730676802 ) ) ;
#17413=AXIS2_PLACEMENT_3D ( 'NONE', #1184, #4219, #12613 ) ;
#17415=VERTEX_POINT ( 'NONE', #25621 ) ;
#17423=CARTESIAN_POINT ( 'NONE',  ( 158.4226497308104058, 5.000000000000004441, 0.000000000000000000 ) ) ;
#17424=DIRECTION ( 'NONE',  ( -0.000000000000000000, -1.000000000000000000, -0.000000000000000000 ) ) ;
#17433=DIRECTION ( 'NONE',  ( 0.000000000000000000, 0.000000000000000000, -1.000000000000000000 ) ) ;
#17435=CARTESIAN_POINT ( 'NONE',  ( 153.7500000000000284, -6.000000000000005329, 0.000000000000000000 ) ) ;
#17440=EDGE_LOOP ( 'NONE', ( #12401, #1014, #26718, #28570 ) ) ;
#17441=CARTESIAN_POINT ( 'NONE',  ( 145.2187500000000000, 2.485281374238555774, -6.000000000000005329 ) ) ;
#17442=CARTESIAN_POINT ( 'NONE',  ( 161.3226222142385495, -5.782726518792725479, 0.7502167045361700648 ) ) ;
#17443=AXIS2_PLACEMENT_3D ( 'NONE', #9342, #23183, #15989 ) ;
#17444=( BOUNDED_CURVE ( )  B_SPLINE_CURVE ( 2, ( #27450, #8750, #29464, #25306, #15544, #5969, #29622, #22730, #8266 ),
 .UNSPECIFIED., .F., .F. ) 
 B_SPLINE_CURVE_WITH_KNOTS ( ( 3, 2, 2, 2, 3 ),
 ( 0.6124999999999991562, 0.6187499999999994671, 0.6249999999999996669, 0.6312499999999998668, 0.6375000000000001776 ),
 .UNSPECIFIED. ) 
 CURVE ( )  GEOMETRIC_REPRESENTATION_ITEM ( )  RATIONAL_B_SPLINE_CURVE ( ( 1.000000000000010880, 0.9238795325112759693, 1.000000000000000000, 0.9238795325112867385, 1.000000000000000000, 0.9238795325112867385, 1.000000000000000000, 0.9238795325112840739, 1.000000000000002665 ) ) 
 REPRESENTATION_ITEM ( '' )  );
#17451=EDGE_CURVE ( 'NONE', #2002, #1706, #19327, .T. ) ;
#17455=CIRCLE ( 'NONE', #9596, 1.000000000000000888 ) ;
#17458=CARTESIAN_POINT ( 'NONE',  ( 135.5572654074498757, -8.633464121020763216, -8.190187016698715183 ) ) ;
#17459=CARTESIAN_POINT ( 'NONE',  ( 135.0583403565103993, -7.808325495672431948, 8.343593232207838994 ) ) ;
#17469=CARTESIAN_POINT ( 'NONE',  ( 151.9761751345948255, 3.889087296526011706, 3.889087296526011706 ) ) ;
#17480=VECTOR ( 'NONE', #4550, 1000.000000000000000 ) ;
#17482=ORIENTED_EDGE ( 'NONE', *, *, #6477, .T. ) ;
#17484=ORIENTED_EDGE ( 'NONE', *, *, #4238, .F. ) ;
#17492=FACE_OUTER_BOUND ( 'NONE', #16085, .T. ) ;
#17493=CARTESIAN_POINT ( 'NONE',  ( 147.4761751345948255, 3.889087296526011706, 3.889087296526011706 ) ) ;
#17497=DIRECTION ( 'NONE',  ( -0.000000000000000000, -0.000000000000000000, -1.000000000000000000 ) ) ;
#17500=( LENGTH_UNIT ( ) NAMED_UNIT ( * ) SI_UNIT ( .MILLI., .METRE. ) );
#17502=CARTESIAN_POINT ( 'NONE',  ( 154.5863248654052313, 0.000000000000000000, 5.500000000000005329 ) ) ;
#17505=CARTESIAN_POINT ( 'NONE',  ( 135.3537157487436673, -8.430252226432825680, 8.227605494166098765 ) ) ;
#17506=CIRCLE ( 'NONE', #18002, 0.5000000000000004441 ) ;
#17509=( LENGTH_UNIT ( ) NAMED_UNIT ( * ) SI_UNIT ( .MILLI., .METRE. ) );
#17511=ORIENTED_EDGE ( 'NONE', *, *, #26950, .F. ) ;
#17514=DIRECTION ( 'NONE',  ( 0.000000000000000000, -1.000000000000000000, 0.000000000000000000 ) ) ;
#17523=AXIS2_PLACEMENT_3D ( 'NONE', #6313, #8473, #6777 ) ;
#17526=CARTESIAN_POINT ( 'NONE',  ( 133.5148502691896510, -3.535533905932725318, -3.535533905932725318 ) ) ;
#17534=ORIENTED_EDGE ( 'NONE', *, *, #15526, .F. ) ;
#17537=SURFACE_STYLE_USAGE ( .BOTH. , #12492 ) ;
#17542=LINE ( 'NONE', #5989, #8209 ) ;
#17543=FACE_OUTER_BOUND ( 'NONE', #16892, .T. ) ;
#17548=STYLED_ITEM ( 'NONE', ( #1309 ), #7074 ) ;
#17554=CARTESIAN_POINT ( 'NONE',  ( 0.9172842643931518047, -15.89806073124487540, 7.323133569090728656 ) ) ;
#17555=VERTEX_POINT ( 'NONE', #21481 ) ;
#17556=AXIS2_PLACEMENT_3D ( 'NONE', #28174, #7144, #23599 ) ;
#17558=FILL_AREA_STYLE ('',( #19988 ) ) ;
#17559=EDGE_CURVE ( 'NONE', #3582, #5384, #7476, .T. ) ;
#17564=CARTESIAN_POINT ( 'NONE',  ( 140.1944936379391322, -11.19449363793818542, 4.371599137206779062 ) ) ;
#17565=COLOUR_RGB ( '', 0.08235294, 0.09019608, 0.10196078) ;
#17566=EDGE_CURVE ( 'NONE', #13568, #22235, #18086, .T. ) ;
#17573=CARTESIAN_POINT ( 'NONE',  ( 148.2038997308104342, 2.071067811865468400, 4.999999999999989342 ) ) ;
#17575=TOROIDAL_SURFACE ( 'NONE', #27818, 14.49999999999999822, 0.5000000000000000000 ) ;
#17579=( BOUNDED_SURFACE ( )  B_SPLINE_SURFACE ( 3, 2, ( 
 ( #30085, #8439, #27609 ),
 ( #15700, #20125, #18445 ),
 ( #16159, #25309, #6425 ),
 ( #13095, #22429, #27313 ),
 ( #18295, #1367, #3964 ),
 ( #10777, #17844, #6586 ),
 ( #13391, #27164, #22734 ),
 ( #20578, #1677, #24866 ),
 ( #8754, #4122, #13544 ),
 ( #22883, #11545, #13858 ),
 ( #4432, #25468, #2145 ),
 ( #23198, #10561, #17638 ) ),
 .UNSPECIFIED., .F., .F., .T. ) 
 B_SPLINE_SURFACE_WITH_KNOTS ( ( 4, 2, 2, 2, 2, 4 ),
 ( 3, 3 ),
 ( 0.001274372683696326294, 0.001674986756246988479, 0.002075600828797650663, 0.002876828973898974597, 0.003678057119000298532, 0.004479285264101622900 ),
 ( 0.000000000000000000, 1.000000000000000000 ),
 .UNSPECIFIED. ) 
 GEOMETRIC_REPRESENTATION_ITEM ( )  RATIONAL_B_SPLINE_SURFACE ( (
 ( 1.000000000000000000, 0.8320502943378437211, 1.000000000000000000),
 ( 1.000000000000000000, 0.8320475279104844191, 1.000000000000000000),
 ( 1.000000000000000000, 0.8309444048799978777, 1.000000000000000000),
 ( 1.000000000000000000, 0.8266812726961745295, 1.000000000000000000),
 ( 1.000000000000000000, 0.8234657432881781203, 1.000000000000000000),
 ( 1.000000000000000000, 0.8113071453214155682, 1.000000000000000000),
 ( 1.000000000000000000, 0.7996314351500605211, 1.000000000000000000),
 ( 1.000000000000000000, 0.7734282707767409226, 1.000000000000000000),
 ( 1.000000000000000000, 0.7587203540637079691, 1.000000000000000000),
 ( 1.000000000000000000, 0.7309429981451178726, 1.000000000000000000),
 ( 1.000000000000000000, 0.7175754434900719625, 1.000000000000000000),
 ( 1.000000000000000000, 0.7071067811865474617, 1.000000000000000000) ) ) 
 REPRESENTATION_ITEM ( '' )  SURFACE ( )  );
#17583=COLOUR_RGB ( '', 0.72549020, 0.75294118, 0.79215686) ;
#17589=CARTESIAN_POINT ( 'NONE',  ( 144.9375000000000284, -4.242640687119298093, -4.242640687119298093 ) ) ;
#17596=CARTESIAN_POINT ( 'NONE',  ( 144.9375000000000284, -4.242640687119298093, -4.242640687119298093 ) ) ;
#17597=CARTESIAN_POINT ( 'NONE',  ( 161.4683586609244799, -4.012149146953796652, -4.464357517409463405 ) ) ;
#17598=ORIENTED_EDGE ( 'NONE', *, *, #13407, .T. ) ;
#17603=EDGE_LOOP ( 'NONE', ( #17265, #16490, #19135, #16714 ) ) ;
#17611=CARTESIAN_POINT ( 'NONE',  ( 140.0255071013316410, -11.51275355066580453, -4.738782956804194590 ) ) ;
#17614=CARTESIAN_POINT ( 'NONE',  ( -4.999999999999990230, -24.99999999999999289, 5.000000000000004441 ) ) ;
#17616=CARTESIAN_POINT ( 'NONE',  ( 134.9999999999999716, 5.403404080199650572, 2.230070723382028053 ) ) ;
#17622=CARTESIAN_POINT ( 'NONE',  ( 150.9523502691896510, 0.000000000000000000, 5.000000000000004441 ) ) ;
#17624=CARTESIAN_POINT ( 'NONE',  ( 150.8363248654052029, 0.000000000000000000, -5.500000000000005329 ) ) ;
#17625=CARTESIAN_POINT ( 'NONE',  ( 144.8363248654052029, 0.000000000000000000, -5.500000000000005329 ) ) ;
#17626=DIRECTION ( 'NONE',  ( 1.000000000000000000, 0.000000000000000000, 0.000000000000000000 ) ) ;
#17627=EDGE_CURVE ( 'NONE', #15465, #13349, #10244, .T. ) ;
#17628=DIRECTION ( 'NONE',  ( 0.000000000000000000, 0.000000000000000000, -1.000000000000000000 ) ) ;
#17632=CARTESIAN_POINT ( 'NONE',  ( 160.8750000000000568, 0.000000000000000000, 6.000000000000005329 ) ) ;
#17638=CARTESIAN_POINT ( 'NONE',  ( 160.0000000000000284, -12.64911064067352164, 3.000000000000002220 ) ) ;
#17644=AXIS2_PLACEMENT_3D ( 'NONE', #23354, #16459, #2722 ) ;
#17645=ORIENTED_EDGE ( 'NONE', *, *, #5555, .F. ) ;
#17647=CARTESIAN_POINT ( 'NONE',  ( 146.1636751345948255, 0.000000000000000000, 5.500000000000005329 ) ) ;
#17648=CARTESIAN_POINT ( 'NONE',  ( 141.1800748654052029, -2.278174593051950136, 5.500000000000074607 ) ) ;
#17659=CARTESIAN_POINT ( 'NONE',  ( 135.0000000000000284, -9.047800747817552391, 7.500000000000007105 ) ) ;
#17662=FACE_OUTER_BOUND ( 'NONE', #20536, .T. ) ;
#17663=CARTESIAN_POINT ( 'NONE',  ( 161.3437500000000568, -6.000000000000005329, -2.485281374238556218 ) ) ;
#17666=EDGE_CURVE ( 'NONE', #6328, #7272, #26813, .T. ) ;
#17667=VERTEX_POINT ( 'NONE', #8699 ) ;
#17671=VERTEX_POINT ( 'NONE', #15013 ) ;
#17674=( GEOMETRIC_REPRESENTATION_CONTEXT ( 3 ) GLOBAL_UNCERTAINTY_ASSIGNED_CONTEXT ( ( #26936 ) ) GLOBAL_UNIT_ASSIGNED_CONTEXT ( ( #17500, #27429, #10897 ) ) REPRESENTATION_CONTEXT ( 'NONE', 'WORKASPACE' ) );
#17675=EDGE_LOOP ( 'NONE', ( #21696, #3955, #19045, #2827 ) ) ;
#17677=CARTESIAN_POINT ( 'NONE',  ( 156.1875000000000284, 4.242640687119269671, 4.242640687119298093 ) ) ;
#17688=CARTESIAN_POINT ( 'NONE',  ( -0.07769256095284111929, -15.23231281889970390, -7.499999999999977796 ) ) ;
#17692=CARTESIAN_POINT ( 'NONE',  ( 0.7560530053056007116, -15.51661680578449598, -8.092351268349677440 ) ) ;
#17696=EDGE_CURVE ( 'NONE', #22958, #5354, #16589, .T. ) ;
#17699=CARTESIAN_POINT ( 'NONE',  ( -4.999999999999886313, -70.00000000000001421, 8.000000000000007105 ) ) ;
#17706=CARTESIAN_POINT ( 'NONE',  ( 0.000000000000000000, -10.50000000000000888, 8.500000000000007105 ) ) ;
#17707=EDGE_CURVE ( 'NONE', #13841, #19367, #3272, .T. ) ;
#17714=UNCERTAINTY_MEASURE_WITH_UNIT (LENGTH_MEASURE( 1.000000000000000082E-05 ), #17303, 'distance_accuracy_value', 'NONE');
#17717=CARTESIAN_POINT ( 'NONE',  ( 143.1562500000000284, -6.000000000000005329, 2.485281374238555774 ) ) ;
#17719=ORIENTED_EDGE ( 'NONE', *, *, #7803, .F. ) ;
#17722=CARTESIAN_POINT ( 'NONE',  ( 140.9136751345948539, 0.000000000000000000, -5.500000000000005329 ) ) ;
#17728=CARTESIAN_POINT ( 'NONE',  ( 150.0788997308104058, -4.999999999999989342, 2.071067811865468400 ) ) ;
#17742=VERTEX_POINT ( 'NONE', #13804 ) ;
#17744=CARTESIAN_POINT ( 'NONE',  ( 147.9375000000000284, -4.242640687119298093, -4.242640687119298093 ) ) ;
#17748=ORIENTED_EDGE ( 'NONE', *, *, #25996, .T. ) ;
#17749=CARTESIAN_POINT ( 'NONE',  ( 142.6875000000000284, 4.242640687119269671, 4.242640687119298093 ) ) ;
#17750=CARTESIAN_POINT ( 'NONE',  ( 161.1978354363685924, -3.302530014113373102, 4.653882225248398896 ) ) ;
#17751=AXIS2_PLACEMENT_3D ( 'NONE', #17277, #26738, #22319 ) ;
#17768=CARTESIAN_POINT ( 'NONE',  ( -1.000000000000000888, 9.000000000000007105, -4.000000000000003553 ) ) ;
#17774=CARTESIAN_POINT ( 'NONE',  ( 137.2425748654051461, -2.278174593052383567, -5.499999999999640288 ) ) ;
#17777=UNCERTAINTY_MEASURE_WITH_UNIT (LENGTH_MEASURE( 1.000000000000000082E-05 ), #11908, 'distance_accuracy_value', 'NONE');
#17779=CARTESIAN_POINT ( 'NONE',  ( -4.999999999999886313, -10.50000000000000888, -7.500000000000007105 ) ) ;
#17783=CARTESIAN_POINT ( 'NONE',  ( 153.2961002691896795, 2.071067811865468400, -4.999999999999989342 ) ) ;
#17785=CARTESIAN_POINT ( 'NONE',  ( 140.0000000000000853, -9.835711086345112264, -7.609525942436604851 ) ) ;
#17786=CYLINDRICAL_SURFACE ( 'NONE', #13352, 0.5000000000000004441 ) ;
#17791=VERTEX_POINT ( 'NONE', #22990 ) ;
#17792=CARTESIAN_POINT ( 'NONE',  ( 160.0312500000000284, -2.485281374238555774, -6.000000000000005329 ) ) ;
#17802=DIRECTION ( 'NONE',  ( 1.000000000000000000, -0.000000000000000000, -0.000000000000000000 ) ) ;
#17807=ADVANCED_FACE ( 'NONE', ( #2093 ), #23305, .T. ) ;
#17810=DIRECTION ( 'NONE',  ( -0.000000000000000000, -0.000000000000000000, -1.000000000000000000 ) ) ;
#17815=CARTESIAN_POINT ( 'NONE',  ( -0.1262135825162392089, -9.436893208741910399, 4.496381089953947807 ) ) ;
#17821=CARTESIAN_POINT ( 'NONE',  ( 135.0000000000000284, -7.893250067244766299, 8.123627818918411236 ) ) ;
#17822=EDGE_LOOP ( 'NONE', ( #22449, #14693, #27782, #25041 ) ) ;
#17832=CARTESIAN_POINT ( 'NONE',  ( 149.7113248654052313, 5.500000000000005329, 0.000000000000000000 ) ) ;
#17837=ORIENTED_EDGE ( 'NONE', *, *, #23285, .T. ) ;
#17838=CARTESIAN_POINT ( 'NONE',  ( 155.8125000000000284, 4.242640687119298093, -4.242640687119298093 ) ) ;
#17844=CARTESIAN_POINT ( 'NONE',  ( 159.6387256973390834, -11.39945094249770108, 3.799649049763677233 ) ) ;
#17851=CARTESIAN_POINT ( 'NONE',  ( 160.0185456724816220, -11.17912010889672381, -4.362636621731123654 ) ) ;
#17852=DIRECTION ( 'NONE',  ( -1.000000000000000000, 0.000000000000000000, 0.000000000000000000 ) ) ;
#17853=DIRECTION ( 'NONE',  ( 1.000000000000000000, 0.000000000000000000, 0.000000000000000000 ) ) ;
#17860=( BOUNDED_CURVE ( )  B_SPLINE_CURVE ( 2, ( #6079, #29414, #15494, #8384, #17179, #27111, #5607, #24355, #15014 ),
 .UNSPECIFIED., .F., .T. ) 
 B_SPLINE_CURVE_WITH_KNOTS ( ( 3, 2, 2, 2, 3 ),
 ( 0.4374999999999999445, 0.4437499999999997002, 0.4499999999999994005, 0.4562499999999992673, 0.4624999999999990230 ),
 .UNSPECIFIED. ) 
 CURVE ( )  GEOMETRIC_REPRESENTATION_ITEM ( )  RATIONAL_B_SPLINE_CURVE ( ( 1.000000000000000666, 0.9238795325112860723, 1.000000000000000000, 0.9238795325112867385, 1.000000000000000000, 0.9238795325112867385, 1.000000000000000000, 0.9238795325112989509, 0.9999999999999877875 ) ) 
 REPRESENTATION_ITEM ( '' )  );
#17864=ORIENTED_EDGE ( 'NONE', *, *, #2159, .F. ) ;
#17868=CARTESIAN_POINT ( 'NONE',  ( 138.3898502691896510, 3.535533905932725318, -3.535533905932725318 ) ) ;
#17869=ORIENTED_EDGE ( 'NONE', *, *, #19013, .F. ) ;
#17874=CARTESIAN_POINT ( 'NONE',  ( 140.5000000328705028, -11.02580175850478383, -4.736714422037297645 ) ) ;
#17877=CARTESIAN_POINT ( 'NONE',  ( -4.999999999999913847, -65.50000000000001421, 8.000000000000007105 ) ) ;
#17879=CARTESIAN_POINT ( 'NONE',  ( 144.0000000000000284, 6.000000000000005329, 0.000000000000000000 ) ) ;
#17880=ORIENTED_EDGE ( 'NONE', *, *, #15526, .T. ) ;
#17881=AXIS2_PLACEMENT_3D ( 'NONE', #5078, #2781, #2931 ) ;
#17885=CARTESIAN_POINT ( 'NONE',  ( 135.9449251345948539, -5.500000000000012434, 2.278174593052012309 ) ) ;
#17889=CARTESIAN_POINT ( 'NONE',  ( 152.9851497308104058, -3.535533905932725318, 3.535533905932725318 ) ) ;
#17896=ORIENTED_EDGE ( 'NONE', *, *, #18471, .F. ) ;
#17898=DIRECTION ( 'NONE',  ( 1.000000000000000000, 1.734723475976807094E-15, 0.000000000000000000 ) ) ;
#17902=CARTESIAN_POINT ( 'NONE',  ( 143.8125000000000284, 4.242640687119298093, -4.242640687119298093 ) ) ;
#17905=DIRECTION ( 'NONE',  ( 0.000000000000000000, 0.000000000000000000, -1.000000000000000000 ) ) ;
#17906=ORIENTED_EDGE ( 'NONE', *, *, #4286, .F. ) ;
#17907=CARTESIAN_POINT ( 'NONE',  ( 136.1250000000000284, 0.000000000000000000, -6.000000000000005329 ) ) ;
#17908=CARTESIAN_POINT ( 'NONE',  ( 161.1037658773653050, -2.857005778783127844E-13, 5.603765877365280090 ) ) ;
#17909=EDGE_CURVE ( 'NONE', #15017, #17667, #825, .T. ) ;
#17911=EDGE_CURVE ( 'NONE', #1653, #15017, #15091, .T. ) ;
#17913=B_SPLINE_CURVE_WITH_KNOTS ( 'NONE', 3,
 ( #26153, #11938, #4812, #12232 ),
 .UNSPECIFIED., .F., .F.,
 ( 4, 4 ),
 ( 0.000000000000000000, 0.0002043583609089620558 ),
 .UNSPECIFIED. ) ;
#17922=CARTESIAN_POINT ( 'NONE',  ( 148.1175748654052313, 5.500000000000012434, -2.278174593052012309 ) ) ;
#17932=CARTESIAN_POINT ( 'NONE',  ( 152.8273502691896510, -5.000000000000004441, 0.000000000000000000 ) ) ;
#17933=CARTESIAN_POINT ( 'NONE',  ( 150.5699251345948255, 2.278174593052259667, 5.499999999999763745 ) ) ;
#17934=CARTESIAN_POINT ( 'NONE',  ( 161.0874653000716989, -5.321804761115118687, -1.753823027392139577 ) ) ;
#17936=TOROIDAL_SURFACE ( 'NONE', #1195, 29.00000000000000000, 1.000000000000000000 ) ;
#17942=CARTESIAN_POINT ( 'NONE',  ( 154.6875000000000284, 4.242640687119269671, 4.242640687119298093 ) ) ;
#17944=LINE ( 'NONE', #3766, #10359 ) ;
#17946=EDGE_CURVE ( 'NONE', #16741, #25006, #15773, .T. ) ;
#17947=ORIENTED_EDGE ( 'NONE', *, *, #17946, .F. ) ;
#17955=EDGE_CURVE ( 'NONE', #17415, #5531, #20967, .T. ) ;
#17956=EDGE_LOOP ( 'NONE', ( #13703, #12181, #18582, #14689 ) ) ;
#17957=DIRECTION ( 'NONE',  ( 0.000000000000000000, 0.000000000000000000, 1.000000000000000000 ) ) ;
#17969=DIRECTION ( 'NONE',  ( -0.000000000000000000, 0.000000000000000000, -1.000000000000000000 ) ) ;
#17970=DIRECTION ( 'NONE',  ( 0.000000000000000000, 0.000000000000000000, -1.000000000000000000 ) ) ;
#17978=DIRECTION ( 'NONE',  ( 0.000000000000000000, 0.000000000000000000, -1.000000000000000000 ) ) ;
#17980=EDGE_CURVE ( 'NONE', #2648, #8247, #26853, .T. ) ;
#17987=CARTESIAN_POINT ( 'NONE',  ( 154.1250000000000284, 0.000000000000000000, -6.000000000000005329 ) ) ;
#17999=VERTEX_POINT ( 'NONE', #966 ) ;
#18002=AXIS2_PLACEMENT_3D ( 'NONE', #4515, #18825, #11312 ) ;
#18003=CARTESIAN_POINT ( 'NONE',  ( 159.9311390374854227, -11.50936040660355353, -3.430377613042744578 ) ) ;
#18009=CARTESIAN_POINT ( 'NONE',  ( -4.999999999999879208, -9.000000000000007105, -5.000000000000004441 ) ) ;
#18011=CARTESIAN_POINT ( 'NONE',  ( 148.1324251345948255, -5.500000000000012434, -2.278174593052012309 ) ) ;
#18016=STYLED_ITEM ( 'NONE', ( #16208 ), #24129 ) ;
#18020=CARTESIAN_POINT ( 'NONE',  ( 141.0148502691896510, -3.535533905932725318, -3.535533905932725318 ) ) ;
#18027=CARTESIAN_POINT ( 'NONE',  ( 140.0000000000000284, -10.99818166789400919, -4.800000000000004263 ) ) ;
#18032=CARTESIAN_POINT ( 'NONE',  ( 139.6875000000000284, 4.242640687119269671, 4.242640687119298093 ) ) ;
#18033=VERTEX_POINT ( 'NONE', #18512 ) ;
#18037=AXIS2_PLACEMENT_3D ( 'NONE', #18614, #23219, #4303 ) ;
#18039=( BOUNDED_CURVE ( )  B_SPLINE_CURVE ( 2, ( #20792, #1139, #15323, #19894, #13436, #22783, #11122, #20470, #16808 ),
 .UNSPECIFIED., .F., .T. ) 
 B_SPLINE_CURVE_WITH_KNOTS ( ( 3, 2, 2, 2, 3 ),
 ( 0.1624999999999987566, 0.1687499999999989564, 0.1749999999999992673, 0.1812499999999994948, 0.1874999999999996947 ),
 .UNSPECIFIED. ) 
 CURVE ( )  GEOMETRIC_REPRESENTATION_ITEM ( )  RATIONAL_B_SPLINE_CURVE ( ( 1.000000000000014877, 0.9238795325112718615, 1.000000000000000000, 0.9238795325112867385, 1.000000000000000000, 0.9238795325112867385, 1.000000000000000000, 0.9238795325112904022, 0.9999999999999963363 ) ) 
 REPRESENTATION_ITEM ( '' )  );
#18040=CARTESIAN_POINT ( 'NONE',  ( 149.7976497308104058, 0.000000000000000000, 5.000000000000004441 ) ) ;
#18042=CYLINDRICAL_SURFACE ( 'NONE', #24343, 0.5000000000000004441 ) ;
#18049=ORIENTED_EDGE ( 'NONE', *, *, #4729, .T. ) ;
#18052=DIRECTION ( 'NONE',  ( 1.000000000000000000, 1.734723475976843579E-16, -0.000000000000000000 ) ) ;
#18054=AXIS2_PLACEMENT_3D ( 'NONE', #28932, #17312, #695 ) ;
#18056=CARTESIAN_POINT ( 'NONE',  ( 146.8125000000000284, 4.242640687119298093, -4.242640687119298093 ) ) ;
#18058=CARTESIAN_POINT ( 'NONE',  ( 116.0000000000000142, 0.000000000000000000, 0.000000000000000000 ) ) ;
#18060=ORIENTED_EDGE ( 'NONE', *, *, #27593, .F. ) ;
#18061=CARTESIAN_POINT ( 'NONE',  ( 140.6250000000000284, 0.000000000000000000, -6.000000000000005329 ) ) ;
#18069=ORIENTED_EDGE ( 'NONE', *, *, #11907, .F. ) ;
#18071=CARTESIAN_POINT ( 'NONE',  ( 135.5000000000000284, -54.99999999999993605, -7.500000000000007105 ) ) ;
#18074=CIRCLE ( 'NONE', #25890, 16.50000000000000355 ) ;
#18081=DIRECTION ( 'NONE',  ( 0.000000000000000000, 0.000000000000000000, 1.000000000000000000 ) ) ;
#18083=CARTESIAN_POINT ( 'NONE',  ( 150.0148502691896510, -3.535533905932725318, -3.535533905932725318 ) ) ;
#18085=CARTESIAN_POINT ( 'NONE',  ( 159.0000000000000284, -12.00000000000001066, 4.000000000000003553 ) ) ;
#18086=CIRCLE ( 'NONE', #16149, 0.9999999999999993339 ) ;
#18088=CARTESIAN_POINT ( 'NONE',  ( 116.0000000000000142, 0.000000000000000000, 0.000000000000000000 ) ) ;
#18092=CARTESIAN_POINT ( 'NONE',  ( 156.0937500000000000, 6.000000000000005329, 2.485281374238585972 ) ) ;
#18093=DIRECTION ( 'NONE',  ( 1.000000000000000000, 0.000000000000000000, 0.000000000000000000 ) ) ;
#18096=ORIENTED_EDGE ( 'NONE', *, *, #29029, .F. ) ;
#18101=CARTESIAN_POINT ( 'NONE',  ( -19.49999999999998224, -54.99999999999990763, -7.500000000000007105 ) ) ;
#18102=DIRECTION ( 'NONE',  ( -1.000000000000000000, -1.067522139062651904E-16, 0.000000000000000000 ) ) ;
#18105=( NAMED_UNIT ( * ) PLANE_ANGLE_UNIT ( ) SI_UNIT ( $, .RADIAN. ) );
#18116=ORIENTED_EDGE ( 'NONE', *, *, #18509, .T. ) ;
#18120=EDGE_CURVE ( 'NONE', #25268, #16010, #21939, .T. ) ;
#18122=( BOUNDED_SURFACE ( )  B_SPLINE_SURFACE ( 3, 2, ( 
 ( #8783, #20306, #27483 ),
 ( #1704, #29503, #19990 ),
 ( #17874, #29651, #8618 ),
 ( #11258, #18027, #13121 ) ),
 .UNSPECIFIED., .F., .F., .T. ) 
 B_SPLINE_SURFACE_WITH_KNOTS ( ( 4, 4 ),
 ( 3, 3 ),
 ( -1.355252715606880543E-18, 0.0002125775066526909465 ),
 ( 0.000000000000000000, 1.000000000000000000 ),
 .UNSPECIFIED. ) 
 GEOMETRIC_REPRESENTATION_ITEM ( )  RATIONAL_B_SPLINE_SURFACE ( (
 ( 1.000000000000000000, 0.7576044462920076272, 1.000000000000000000),
 ( 1.000000000000000000, 0.7424605758826383628, 1.000000000000000000),
 ( 1.000000000000000000, 0.7257758655053253571, 1.000000000000000000),
 ( 1.000000000000000000, 0.7071067811865475727, 1.000000000000000000) ) ) 
 REPRESENTATION_ITEM ( '' )  SURFACE ( )  );
#18124=DIRECTION ( 'NONE',  ( -6.938893903907221278E-15, 1.000000000000000000, 0.000000000000000000 ) ) ;
#18131=CARTESIAN_POINT ( 'NONE',  ( 159.5625000000000284, -4.242640687119298093, 4.242640687119298093 ) ) ;
#18133=CIRCLE ( 'NONE', #5349, 0.5000000000000004441 ) ;
#18137=STYLED_ITEM ( 'NONE', ( #24131 ), #14454 ) ;
#18141=CARTESIAN_POINT ( 'NONE',  ( 152.9136751345948539, 0.000000000000000000, -5.500000000000005329 ) ) ;
#18147=CARTESIAN_POINT ( 'NONE',  ( 157.8675748654052313, -5.500000000000012434, 2.278174593052012309 ) ) ;
#18153=CARTESIAN_POINT ( 'NONE',  ( 148.4136751345948539, 0.000000000000000000, -5.500000000000005329 ) ) ;
#18155=CARTESIAN_POINT ( 'NONE',  ( -14.99999999999999289, -54.99999999999990763, 7.500000000000007105 ) ) ;
#18162=ADVANCED_FACE ( 'NONE', ( #25696 ), #4034, .F. ) ;
#18163=CARTESIAN_POINT ( 'NONE',  ( 139.8898502691896510, 3.535533905932725318, -3.535533905932725318 ) ) ;
#18166=EDGE_LOOP ( 'NONE', ( #16451, #27109, #9019, #22510 ) ) ;
#18168=CARTESIAN_POINT ( 'NONE',  ( 116.0000000000000142, 0.000000000000000000, 0.000000000000000000 ) ) ;
#18170=COLOUR_RGB ( '', 0.72549020, 0.75294118, 0.79215686) ;
#18175=CARTESIAN_POINT ( 'NONE',  ( 138.3824251345948255, 5.500000000000012434, 2.278174593052012309 ) ) ;
#18176=CARTESIAN_POINT ( 'NONE',  ( 143.0625000000000284, -4.242640687119298093, 4.242640687119298093 ) ) ;
#18180=VECTOR ( 'NONE', #5139, 1000.000000000000000 ) ;
#18184=CARTESIAN_POINT ( 'NONE',  ( 149.5163997308103774, 4.999999999999989342, 2.071067811865468400 ) ) ;
#18189=FILL_AREA_STYLE_COLOUR ( '', #15051 ) ;
#18190=ADVANCED_FACE ( 'NONE', ( #23416 ), #17575, .T. ) ;
#18191=CARTESIAN_POINT ( 'NONE',  ( 116.0000000000000142, 0.000000000000000000, -5.500000000000000000 ) ) ;
#18194=LINE ( 'NONE', #29363, #16048 ) ;
#18202=CARTESIAN_POINT ( 'NONE',  ( 147.2812500000000284, 2.485281374238585972, 6.000000000000005329 ) ) ;
#18204=PRESENTATION_STYLE_ASSIGNMENT (( #24780 ) ) ;
#18205=CARTESIAN_POINT ( 'NONE',  ( 138.2812500000000284, 2.485281374238585972, 6.000000000000005329 ) ) ;
#18210=ORIENTED_EDGE ( 'NONE', *, *, #27531, .T. ) ;
#18218=CARTESIAN_POINT ( 'NONE',  ( 135.0000000000000284, -54.99999999999993605, 7.500000000000007105 ) ) ;
#18220=CARTESIAN_POINT ( 'NONE',  ( 161.0000000000000284, 0.000000000000000000, -5.500000000000000000 ) ) ;
#18225=CARTESIAN_POINT ( 'NONE',  ( -0.04562205425674009662, -14.50000000000001243, -8.291335958003937634 ) ) ;
#18232=CARTESIAN_POINT ( 'NONE',  ( 147.8363248654052029, 0.000000000000000000, -5.500000000000005329 ) ) ;
#18235=CARTESIAN_POINT ( 'NONE',  ( -4.999999999999886313, -10.00000000000000888, -7.500000000000007105 ) ) ;
#18238=CARTESIAN_POINT ( 'NONE',  ( 154.3125000000000284, 4.242640687119298093, -4.242640687119298093 ) ) ;
#18246=EDGE_CURVE ( 'NONE', #18033, #8327, #12792, .T. ) ;
#18251=CARTESIAN_POINT ( 'NONE',  ( 140.3905920374922403, -9.244723267345564821, -7.652122629818983057 ) ) ;
#18253=DIRECTION ( 'NONE',  ( -0.000000000000000000, -1.000000000000000000, -0.000000000000000000 ) ) ;
#18256=CARTESIAN_POINT ( 'NONE',  ( -0.5000000000000004441, -15.00000000000001421, -7.500000000000007105 ) ) ;
#18257=EDGE_LOOP ( 'NONE', ( #7958, #294, #2796, #27885 ) ) ;
#18259=DIRECTION ( 'NONE',  ( 1.000000000000000000, 0.000000000000000000, 0.000000000000000000 ) ) ;
#18260=EDGE_CURVE ( 'NONE', #16823, #23494, #10788, .T. ) ;
#18261=CARTESIAN_POINT ( 'NONE',  ( 147.7425748654052313, -2.278174593052259667, -5.499999999999763745 ) ) ;
#18262=AXIS2_PLACEMENT_3D ( 'NONE', #25762, #21471, #4708 ) ;
#18266=CARTESIAN_POINT ( 'NONE',  ( 160.3199251345948539, -2.278174593051888408, -5.500000000000135891 ) ) ;
#18269=CARTESIAN_POINT ( 'NONE',  ( 162.1086002691896795, -2.071067811865468400, -4.999999999999989342 ) ) ;
#18271=CARTESIAN_POINT ( 'NONE',  ( 0.7522378546890716722, -15.54348611246722633, 8.040548560309273896 ) ) ;
#18276=CARTESIAN_POINT ( 'NONE',  ( 161.0349825973430313, 2.426008766636172265, 4.985030962988786563 ) ) ;
#18280=VECTOR ( 'NONE', #25952, 1000.000000000000000 ) ;
#18287=CARTESIAN_POINT ( 'NONE',  ( 157.6875000000000284, 4.242640687119269671, 4.242640687119298093 ) ) ;
#18288=EDGE_CURVE ( 'NONE', #11814, #25843, #17542, .T. ) ;
#18295=CARTESIAN_POINT ( 'NONE',  ( 159.6587023700971031, -11.11766146451058113, 4.516663148717062981 ) ) ;
#18299=EDGE_CURVE ( 'NONE', #15465, #15294, #25364, .T. ) ;
#18311=DIRECTION ( 'NONE',  ( 1.000000000000000000, 0.000000000000000000, 0.000000000000000000 ) ) ;
#18314=DIRECTION ( 'NONE',  ( -1.000000000000000000, 0.000000000000000000, 0.000000000000000000 ) ) ;
#18318=CARTESIAN_POINT ( 'NONE',  ( 1.000000000000000888, 0.000000000000000000, 0.000000000000000000 ) ) ;
#18319=CARTESIAN_POINT ( 'NONE',  ( 137.1711002691896795, 4.999999999999989342, 2.071067811865468400 ) ) ;
#18328=ORIENTED_EDGE ( 'NONE', *, *, #5580, .T. ) ;
#18331=CARTESIAN_POINT ( 'NONE',  ( 144.9375000000000284, -4.242640687119298093, -4.242640687119298093 ) ) ;
#18332=EDGE_CURVE ( 'NONE', #16343, #5531, #3520, .T. ) ;
#18334=ORIENTED_EDGE ( 'NONE', *, *, #10438, .F. ) ;
#18335=CARTESIAN_POINT ( 'NONE',  ( -38.99999999999998579, -59.99999999999980105, 4.000000000000003553 ) ) ;
#18337=EDGE_CURVE ( 'NONE', #5051, #16955, #26322, .T. ) ;
#18338=CARTESIAN_POINT ( 'NONE',  ( 124.9999999999999432, -69.50000000000000000, 7.500000000000007105 ) ) ;
#18342=CARTESIAN_POINT ( 'NONE',  ( 143.1413997308104342, 2.071067811865468400, -4.999999999999989342 ) ) ;
#18343=DIRECTION ( 'NONE',  ( 0.000000000000000000, 0.000000000000000000, 1.000000000000000000 ) ) ;
#18346=SURFACE_STYLE_FILL_AREA ( #8640 ) ;
#18351=ORIENTED_EDGE ( 'NONE', *, *, #21571, .T. ) ;
#18356=ORIENTED_EDGE ( 'NONE', *, *, #26976, .F. ) ;
#18358=CARTESIAN_POINT ( 'NONE',  ( 138.5625000000000284, -4.242640687119298093, 4.242640687119298093 ) ) ;
#18359=CARTESIAN_POINT ( 'NONE',  ( 140.5835741348633690, -11.79178706743166494, -4.000000000000005329 ) ) ;
#18360=CARTESIAN_POINT ( 'NONE',  ( 137.8125000000000284, 4.242640687119298093, -4.242640687119298093 ) ) ;
#18362=CIRCLE ( 'NONE', #12971, 15.00000000000000000 ) ;
#18363=ADVANCED_FACE ( 'NONE', ( #24571 ), #13402, .F. ) ;
#18367=ORIENTED_EDGE ( 'NONE', *, *, #2585, .T. ) ;
#18374=CARTESIAN_POINT ( 'NONE',  ( 140.0000000000000284, -54.99999999999990763, -5.000000000000004441 ) ) ;
#18378=CARTESIAN_POINT ( 'NONE',  ( -0.2114713642193710996, -9.788528635780624043, 4.341247053692733004 ) ) ;
#18381=FILL_AREA_STYLE ('',( #13329 ) ) ;
#18383=CARTESIAN_POINT ( 'NONE',  ( 147.6711002691896510, 4.999999999999989342, 2.071067811865468400 ) ) ;
#18385=DIRECTION ( 'NONE',  ( 0.000000000000000000, 0.000000000000000000, -1.000000000000000000 ) ) ;
#18393=ORIENTED_EDGE ( 'NONE', *, *, #25628, .F. ) ;
#18394=CARTESIAN_POINT ( 'NONE',  ( 159.0000000000000284, 6.000000000000005329, 0.000000000000000000 ) ) ;
#18399=ORIENTED_EDGE ( 'NONE', *, *, #22087, .F. ) ;
#18401=ADVANCED_FACE ( 'NONE', ( #11707 ), #25337, .F. ) ;
#18402=EDGE_LOOP ( 'NONE', ( #6268, #28653, #4087, #6845, #16330 ) ) ;
#18410=CARTESIAN_POINT ( 'NONE',  ( 161.0000000000000284, 0.000000000000000000, -12.00000000000000178 ) ) ;
#18415=( LENGTH_UNIT ( ) NAMED_UNIT ( * ) SI_UNIT ( .MILLI., .METRE. ) );
#18418=CARTESIAN_POINT ( 'NONE',  ( 162.2023502691896795, 0.000000000000000000, -5.000000000000004441 ) ) ;
#18419=CARTESIAN_POINT ( 'NONE',  ( -0.07939152865813971227, -15.22963250115830292, 7.558609509503281032 ) ) ;
#18424=DIRECTION ( 'NONE',  ( 0.000000000000000000, 1.000000000000000000, -0.000000000000000000 ) ) ;
#18425=ORIENTED_EDGE ( 'NONE', *, *, #23147, .T. ) ;
#18429=VERTEX_POINT ( 'NONE', #27623 ) ;
#18431=EDGE_CURVE ( 'NONE', #2429, #278, #19055, .T. ) ;
#18434=CARTESIAN_POINT ( 'NONE',  ( 148.2187500000000568, 2.485281374238555774, -6.000000000000005329 ) ) ;
#18436=CIRCLE ( 'NONE', #5146, 9.999999999999998224 ) ;
#18445=CARTESIAN_POINT ( 'NONE',  ( 159.0677334129669873, -12.00000000265806754, 4.000000000000004441 ) ) ;
#18447=ORIENTED_EDGE ( 'NONE', *, *, #17696, .F. ) ;
#18449=DIRECTION ( 'NONE',  ( -0.000000000000000000, -1.000000000000000000, 0.000000000000000000 ) ) ;
#18461=VERTEX_POINT ( 'NONE', #21052 ) ;
#18471=EDGE_CURVE ( 'NONE', #26763, #4156, #4136, .T. ) ;
#18472=EDGE_CURVE ( 'NONE', #20769, #7022, #25644, .T. ) ;
#18478=CARTESIAN_POINT ( 'NONE',  ( 135.3750000000000284, 0.000000000000000000, 6.000000000000005329 ) ) ;
#18483=CARTESIAN_POINT ( 'NONE',  ( 124.9999999999999432, -70.00000000000000000, 8.000000000000007105 ) ) ;
#18489=CARTESIAN_POINT ( 'NONE',  ( 146.1413997308104058, 2.071067811865468400, -4.999999999999989342 ) ) ;
#18491=DIRECTION ( 'NONE',  ( -1.000000000000000000, 0.000000000000000000, 0.000000000000000000 ) ) ;
#18492=LINE ( 'NONE', #23246, #10970 ) ;
#18493=CARTESIAN_POINT ( 'NONE',  ( 156.0074251345948824, 2.278174593052074925, -5.499999999999950262 ) ) ;
#18499=CARTESIAN_POINT ( 'NONE',  ( 0.000000000000000000, 0.000000000000000000, 0.000000000000000000 ) ) ;
#18503=DIRECTION ( 'NONE',  ( -1.000000000000000000, -0.000000000000000000, -0.000000000000000000 ) ) ;
#18505=EDGE_LOOP ( 'NONE', ( #28255, #20184, #3345, #3926 ) ) ;
#18507=CARTESIAN_POINT ( 'NONE',  ( 138.1875000000000284, 4.242640687119269671, 4.242640687119298093 ) ) ;
#18509=EDGE_CURVE ( 'NONE', #15347, #11375, #24403, .T. ) ;
#18510=EDGE_CURVE ( 'NONE', #6339, #10447, #12454, .T. ) ;
#18511=CARTESIAN_POINT ( 'NONE',  ( 138.5625000000000284, -4.242640687119298093, 4.242640687119298093 ) ) ;
#18512=CARTESIAN_POINT ( 'NONE',  ( 141.0000000000000284, -12.00000000000001066, -4.000000000000003553 ) ) ;
#18517=ORIENTED_EDGE ( 'NONE', *, *, #2292, .T. ) ;
#18520=CARTESIAN_POINT ( 'NONE',  ( 140.0769230769231228, -11.53846153846155254, 4.615384615384604317 ) ) ;
#18535=DIRECTION ( 'NONE',  ( 0.000000000000000000, -1.000000000000000000, 0.000000000000000000 ) ) ;
#18537=CARTESIAN_POINT ( 'NONE',  ( 156.3750000000000284, 0.000000000000000000, 6.000000000000005329 ) ) ;
#18543=ADVANCED_FACE ( 'NONE', ( #14888 ), #4888, .F. ) ;
#18546=CARTESIAN_POINT ( 'NONE',  ( 154.8750000000000284, 0.000000000000000000, 6.000000000000005329 ) ) ;
#18550=ORIENTED_EDGE ( 'NONE', *, *, #8515, .T. ) ;
#18557=DIRECTION ( 'NONE',  ( 0.000000000000000000, 0.5151515151515151381, -0.8570991287109668288 ) ) ;
#18560=ORIENTED_EDGE ( 'NONE', *, *, #22645, .T. ) ;
#18561=DIRECTION ( 'NONE',  ( 0.000000000000000000, 1.224646799147351482E-16, 1.000000000000000000 ) ) ;
#18562=CARTESIAN_POINT ( 'NONE',  ( 148.5863248654052313, 0.000000000000000000, 5.500000000000005329 ) ) ;
#18569=FILL_AREA_STYLE ('',( #14280 ) ) ;
#18571=ADVANCED_FACE ( 'NONE', ( #26529 ), #2888, .F. ) ;
#18574=CARTESIAN_POINT ( 'NONE',  ( 161.8273502691896510, -5.000000000000004441, 0.000000000000000000 ) ) ;
#18575=CARTESIAN_POINT ( 'NONE',  ( -0.08067167272386344123, -15.01514411294037110, 8.017838343683242996 ) ) ;
#18576=VERTEX_POINT ( 'NONE', #3037 ) ;
#18581=CYLINDRICAL_SURFACE ( 'NONE', #17443, 1.000000000000000000 ) ;
#18582=ORIENTED_EDGE ( 'NONE', *, *, #18332, .F. ) ;
#18586=CARTESIAN_POINT ( 'NONE',  ( 153.5625000000000568, -4.242640687119298093, 4.242640687119298093 ) ) ;
#18590=ORIENTED_EDGE ( 'NONE', *, *, #12965, .F. ) ;
#18594=CARTESIAN_POINT ( 'NONE',  ( 124.9999999999999432, -65.00000000000000000, 7.500000000000007105 ) ) ;
#18597=SURFACE_SIDE_STYLE ('',( #13861 ) ) ;
#18598=AXIS2_PLACEMENT_3D ( 'NONE', #9869, #25682, #4633 ) ;
#18601=CARTESIAN_POINT ( 'NONE',  ( -4.999999999999984013, -10.50000000000000888, 7.500000000000007105 ) ) ;
#18606=DIRECTION ( 'NONE',  ( 0.000000000000000000, 0.000000000000000000, -1.000000000000000000 ) ) ;
#18608=CARTESIAN_POINT ( 'NONE',  ( 159.5177518860653265, -11.09692667050913428, -4.568096268470709376 ) ) ;
#18614=CARTESIAN_POINT ( 'NONE',  ( -4.999999999999990230, -24.99999999999999289, 8.000000000000007105 ) ) ;
#18617=CARTESIAN_POINT ( 'NONE',  ( -19.99999999999998224, -25.00000000000010658, 7.500000000000007105 ) ) ;
#18620=FACE_OUTER_BOUND ( 'NONE', #22767, .T. ) ;
#18624=ORIENTED_EDGE ( 'NONE', *, *, #18337, .T. ) ;
#18626=CARTESIAN_POINT ( 'NONE',  ( 138.2812500000000284, 2.485281374238585972, 6.000000000000005329 ) ) ;
#18627=VERTEX_POINT ( 'NONE', #23658 ) ;
#18631=SURFACE_STYLE_USAGE ( .BOTH. , #6473 ) ;
#18635=CARTESIAN_POINT ( 'NONE',  ( 134.4977709871273248, -7.448582144714649189, -8.000000000000007105 ) ) ;
#18636=CARTESIAN_POINT ( 'NONE',  ( 144.9226497308104342, 5.000000000000004441, 0.000000000000000000 ) ) ;
#18643=DIRECTION ( 'NONE',  ( 0.000000000000000000, 1.000000000000000000, -0.000000000000000000 ) ) ;
#18644=( GEOMETRIC_REPRESENTATION_CONTEXT ( 3 ) GLOBAL_UNCERTAINTY_ASSIGNED_CONTEXT ( ( #21351 ) ) GLOBAL_UNIT_ASSIGNED_CONTEXT ( ( #29969, #22626, #1562 ) ) REPRESENTATION_CONTEXT ( 'NONE', 'WORKASPACE' ) );
#18645=EDGE_CURVE ( 'NONE', #20381, #15417, #6248, .T. ) ;
#18647=VECTOR ( 'NONE', #14632, 1000.000000000000000 ) ;
#18649=SURFACE_STYLE_FILL_AREA ( #4928 ) ;
#18658=CARTESIAN_POINT ( 'NONE',  ( 142.2187500000000284, 2.485281374238556218, -6.000000000000005329 ) ) ;
#18660=CARTESIAN_POINT ( 'NONE',  ( 142.7886751345948539, 5.500000000000005329, 0.000000000000000000 ) ) ;
#18662=CARTESIAN_POINT ( 'NONE',  ( 132.3750000000000284, 0.000000000000000000, 6.000000000000005329 ) ) ;
#18667=ORIENTED_EDGE ( 'NONE', *, *, #20481, .F. ) ;
#18668=STYLED_ITEM ( 'NONE', ( #26477 ), #979 ) ;
#18671=CARTESIAN_POINT ( 'NONE',  ( 125.0000000000000568, -55.00000000000000711, 7.500000000000007105 ) ) ;
#18675=FACE_OUTER_BOUND ( 'NONE', #18886, .T. ) ;
#18677=ADVANCED_FACE ( 'NONE', ( #27695 ), #1197, .F. ) ;
#18685=CARTESIAN_POINT ( 'NONE',  ( 140.5000000000000284, 0.000000000000000000, 0.000000000000000000 ) ) ;
#18690=CARTESIAN_POINT ( 'NONE',  ( 159.1875000000000284, 4.242640687119269671, 4.242640687119298093 ) ) ;
#18692=VECTOR ( 'NONE', #23212, 1000.000000000000000 ) ;
#18693=CARTESIAN_POINT ( 'NONE',  ( 138.9449251345948824, -5.500000000000012434, 2.278174593052012309 ) ) ;
#18697=VERTEX_POINT ( 'NONE', #20092 ) ;
#18698=CARTESIAN_POINT ( 'NONE',  ( 149.7187500000000568, 2.485281374238555774, -6.000000000000005329 ) ) ;
#18703=VERTEX_POINT ( 'NONE', #26817 ) ;
#18710=PRESENTATION_STYLE_ASSIGNMENT (( #17120 ) ) ;
#18711=CARTESIAN_POINT ( 'NONE',  ( 158.8913997308104058, -2.071067811865468400, 4.999999999999989342 ) ) ;
#18715=EDGE_CURVE ( 'NONE', #3655, #10447, #17306, .T. ) ;
#18725=PRESENTATION_STYLE_ASSIGNMENT (( #23329 ) ) ;
#18726=CARTESIAN_POINT ( 'NONE',  ( 0.1878980370099003760, -15.40048167581654681, 8.313448362010671389 ) ) ;
#18727=VERTEX_POINT ( 'NONE', #16393 ) ;
#18733=CARTESIAN_POINT ( 'NONE',  ( 161.0614794248616590, 1.551837106343485706, 5.349811464556154306 ) ) ;
#18736=DIRECTION ( 'NONE',  ( 1.000000000000000000, 0.000000000000000000, 0.000000000000000000 ) ) ;
#18737=VECTOR ( 'NONE', #19042, 1000.000000000000000 ) ;
#18740=DIRECTION ( 'NONE',  ( 0.000000000000000000, 0.000000000000000000, 1.000000000000000000 ) ) ;
#18741=MECHANICAL_DESIGN_GEOMETRIC_PRESENTATION_REPRESENTATION('',(#28011),#9404);
#18742=EDGE_LOOP ( 'NONE', ( #535, #527, #3028, #20450 ) ) ;
#18743=CARTESIAN_POINT ( 'NONE',  ( 148.9687500000000284, -2.485281374238585972, 6.000000000000005329 ) ) ;
#18744=EDGE_CURVE ( 'NONE', #28218, #6311, #17072, .T. ) ;
#18753=( BOUNDED_CURVE ( )  B_SPLINE_CURVE ( 3, ( #16462, #731, #26083, #14590 ),
 .UNSPECIFIED., .F., .T. ) 
 B_SPLINE_CURVE_WITH_KNOTS ( ( 4, 4 ),
 ( 4.712388980384689674, 6.283185307179586232 ),
 .UNSPECIFIED. ) 
 CURVE ( )  GEOMETRIC_REPRESENTATION_ITEM ( )  RATIONAL_B_SPLINE_CURVE ( ( 1.000000000000000000, 0.8047378541243649375, 0.8047378541243649375, 1.000000000000000000 ) ) 
 REPRESENTATION_ITEM ( '' )  );
#18755=CARTESIAN_POINT ( 'NONE',  ( -0.5000000000000004441, -9.500000000000008882, 8.000000000000007105 ) ) ;
#18761=DIRECTION ( 'NONE',  ( -0.000000000000000000, 1.000000000000000000, 0.000000000000000000 ) ) ;
#18762=CARTESIAN_POINT ( 'NONE',  ( 136.0000000000000284, -9.165151389911669000, 8.000000000000007105 ) ) ;
#18764=CARTESIAN_POINT ( 'NONE',  ( 134.9999999911586883, -7.162772570454863263, -8.424744567432407294 ) ) ;
#18766=ORIENTED_EDGE ( 'NONE', *, *, #23074, .T. ) ;
#18770=CARTESIAN_POINT ( 'NONE',  ( 135.0000000000000284, 0.000000000000000000, -5.500000000000000000 ) ) ;
#18773=VECTOR ( 'NONE', #10095, 1000.000000000000000 ) ;
#18782=CARTESIAN_POINT ( 'NONE',  ( 137.9062500000000568, 6.000000000000005329, -2.485281374238555774 ) ) ;
#18783=EDGE_CURVE ( 'NONE', #8182, #7800, #4522, .T. ) ;
#18786=CYLINDRICAL_SURFACE ( 'NONE', #25026, 5.500000000000000000 ) ;
#18790=CARTESIAN_POINT ( 'NONE',  ( 1.000000000000000888, -14.99923475244192339, 9.015151515151522688 ) ) ;
#18792=CARTESIAN_POINT ( 'NONE',  ( 143.0476497308104058, 0.000000000000000000, -5.000000000000004441 ) ) ;
#18795=LINE ( 'NONE', #8953, #25654 ) ;
#18798=FILL_AREA_STYLE_COLOUR ( '', #23505 ) ;
#18799=DIRECTION ( 'NONE',  ( -1.000000000000000000, -6.938893903907221278E-15, 0.000000000000000000 ) ) ;
#18805=AXIS2_PLACEMENT_3D ( 'NONE', #20700, #11038, #18259 ) ;
#18809=CARTESIAN_POINT ( 'NONE',  ( 141.0937500000000284, 6.000000000000005329, 2.485281374238585972 ) ) ;
#18812=CARTESIAN_POINT ( 'NONE',  ( 159.7351497308104058, 3.535533905932725318, -3.535533905932725318 ) ) ;
#18815=AXIS2_PLACEMENT_3D ( 'NONE', #5516, #27170, #17853 ) ;
#18817=CARTESIAN_POINT ( 'NONE',  ( 135.0000000000000284, 0.000000000000000000, -11.00000000000000355 ) ) ;
#18825=DIRECTION ( 'NONE',  ( 6.938893903907221278E-15, -1.000000000000000000, 0.000000000000000000 ) ) ;
#18828=CARTESIAN_POINT ( 'NONE',  ( 140.0000000000000000, -10.00000000000000888, 7.500000000000000888 ) ) ;
#18836=AXIS2_PLACEMENT_3D ( 'NONE', #26578, #12646, #15088 ) ;
#18838=DIRECTION ( 'NONE',  ( -0.000000000000000000, -0.000000000000000000, -1.000000000000000000 ) ) ;
#18839=( GEOMETRIC_REPRESENTATION_CONTEXT ( 3 ) GLOBAL_UNCERTAINTY_ASSIGNED_CONTEXT ( ( #9661 ) ) GLOBAL_UNIT_ASSIGNED_CONTEXT ( ( #29131, #8091, #24232 ) ) REPRESENTATION_CONTEXT ( 'NONE', 'WORKASPACE' ) );
#18840=CARTESIAN_POINT ( 'NONE',  ( 159.7500000000000284, -6.000000000000005329, 0.000000000000000000 ) ) ;
#18841=DIRECTION ( 'NONE',  ( 0.000000000000000000, 0.000000000000000000, -1.000000000000000000 ) ) ;
#18848=ORIENTED_EDGE ( 'NONE', *, *, #18961, .T. ) ;
#18849=CARTESIAN_POINT ( 'NONE',  ( 149.0625000000000284, -4.242640687119298093, 4.242640687119298093 ) ) ;
#18853=LINE ( 'NONE', #12102, #9209 ) ;
#18861=AXIS2_PLACEMENT_3D ( 'NONE', #9107, #8964, #28 ) ;
#18862=CARTESIAN_POINT ( 'NONE',  ( 154.2976497308104342, 0.000000000000000000, 5.000000000000004441 ) ) ;
#18867=CARTESIAN_POINT ( 'NONE',  ( 147.2738248654052313, -3.889087296526011706, 3.889087296526011706 ) ) ;
#18876=CARTESIAN_POINT ( 'NONE',  ( 161.6398502691896510, -3.535533905932752852, 3.535533905932725318 ) ) ;
#18877=CARTESIAN_POINT ( 'NONE',  ( 135.0000000000000284, -7.635558407351254573, 8.089926835396470395 ) ) ;
#18880=UNCERTAINTY_MEASURE_WITH_UNIT (LENGTH_MEASURE( 1.000000000000000082E-05 ), #2670, 'distance_accuracy_value', 'NONE');
#18886=EDGE_LOOP ( 'NONE', ( #25625, #619, #25064 ) ) ;
#18893=EDGE_CURVE ( 'NONE', #16955, #20809, #26605, .T. ) ;
#18897=CARTESIAN_POINT ( 'NONE',  ( 150.6562500000000284, -6.000000000000005329, 2.485281374238555774 ) ) ;
#18898=EDGE_LOOP ( 'NONE', ( #26555, #22291, #17482, #2008 ) ) ;
#18903=ORIENTED_EDGE ( 'NONE', *, *, #11013, .T. ) ;
#18904=DIRECTION ( 'NONE',  ( 1.000000000000000000, 0.000000000000000000, 0.000000000000000000 ) ) ;
#18909=LINE ( 'NONE', #27614, #20721 ) ;
#18910=CARTESIAN_POINT ( 'NONE',  ( 135.5000000000000000, -24.99999999999999289, 7.500000000000007105 ) ) ;
#18916=UNCERTAINTY_MEASURE_WITH_UNIT (LENGTH_MEASURE( 1.000000000000000082E-05 ), #19637, 'distance_accuracy_value', 'NONE');
#18918=CARTESIAN_POINT ( 'NONE',  ( 135.2061204155054099, -8.336295798213267716, -8.142448489966165326 ) ) ;
#18926=DIRECTION ( 'NONE',  ( 0.000000000000000000, 0.000000000000000000, -1.000000000000000000 ) ) ;
#18936=ORIENTED_EDGE ( 'NONE', *, *, #12182, .T. ) ;
#18938=CARTESIAN_POINT ( 'NONE',  ( 151.5863248654052313, 0.000000000000000000, 5.500000000000005329 ) ) ;
#18939=CARTESIAN_POINT ( 'NONE',  ( 137.1562500000000284, -6.000000000000005329, 2.485281374238555774 ) ) ;
#18943=FILL_AREA_STYLE_COLOUR ( '', #21605 ) ;
#18945=DIRECTION ( 'NONE',  ( 0.000000000000000000, 0.000000000000000000, -1.000000000000000000 ) ) ;
#18947=CARTESIAN_POINT ( 'NONE',  ( 142.5788997308104058, -4.999999999999989342, 2.071067811865468400 ) ) ;
#18949=DIRECTION ( 'NONE',  ( -0.000000000000000000, -1.000000000000000000, 0.000000000000000000 ) ) ;
#18951=CIRCLE ( 'NONE', #25265, 17.50000000000000355 ) ;
#18957=ORIENTED_EDGE ( 'NONE', *, *, #12342, .T. ) ;
#18958=EDGE_CURVE ( 'NONE', #21900, #7029, #30224, .T. ) ;
#18960=LINE ( 'NONE', #27973, #3089 ) ;
#18961=EDGE_CURVE ( 'NONE', #24855, #12501, #23408, .T. ) ;
#18963=AXIS2_PLACEMENT_3D ( 'NONE', #17614, #8519, #26932 ) ;
#18966=CARTESIAN_POINT ( 'NONE',  ( 139.4062500000000284, 6.000000000000005329, -2.485281374238556218 ) ) ;
#18970=CARTESIAN_POINT ( 'NONE',  ( 132.6562500000000284, -6.000000000000005329, 2.485281374238555774 ) ) ;
#18972=( GEOMETRIC_REPRESENTATION_CONTEXT ( 3 ) GLOBAL_UNCERTAINTY_ASSIGNED_CONTEXT ( ( #23770 ) ) GLOBAL_UNIT_ASSIGNED_CONTEXT ( ( #25367, #6943, #14360 ) ) REPRESENTATION_CONTEXT ( 'NONE', 'WORKASPACE' ) );
#18980=CARTESIAN_POINT ( 'NONE',  ( 140.8041911596568241, -11.60838231931462339, -4.059228028635601504 ) ) ;
#18983=AXIS2_PLACEMENT_3D ( 'NONE', #14093, #53, #13780 ) ;
#18986=DIRECTION ( 'NONE',  ( -1.000000000000000000, -1.067522139062651411E-16, 0.000000000000000000 ) ) ;
#18993=CARTESIAN_POINT ( 'NONE',  ( 142.8898502691896510, 3.535533905932725318, -3.535533905932725318 ) ) ;
#18995=CARTESIAN_POINT ( 'NONE',  ( 159.6562500000000568, -6.000000000000005329, 2.485281374238556218 ) ) ;
#18998=CARTESIAN_POINT ( 'NONE',  ( -0.5000000000000004441, -10.50000000000000888, -8.000000000000007105 ) ) ;
#19001=ORIENTED_EDGE ( 'NONE', *, *, #27883, .T. ) ;
#19002=CARTESIAN_POINT ( 'NONE',  ( 151.5937500000000284, 6.000000000000005329, 2.485281374238585972 ) ) ;
#19005=FACE_OUTER_BOUND ( 'NONE', #29676, .T. ) ;
#19012=CARTESIAN_POINT ( 'NONE',  ( 153.9226497308104058, 5.000000000000004441, 0.000000000000000000 ) ) ;
#19013=EDGE_CURVE ( 'NONE', #11662, #379, #12828, .T. ) ;
#19018=B_SPLINE_CURVE_WITH_KNOTS ( 'NONE', 3,
 ( #19735, #29083, #17611, #20209 ),
 .UNSPECIFIED., .F., .F.,
 ( 4, 4 ),
 ( 0.000000000000000000, 0.0004007166227139782183 ),
 .UNSPECIFIED. ) ;
#19022=CARTESIAN_POINT ( 'NONE',  ( 160.7886751345948255, 5.500000000000005329, 0.000000000000000000 ) ) ;
#19024=VECTOR ( 'NONE', #8305, 1000.000000000000000 ) ;
#19032=CARTESIAN_POINT ( 'NONE',  ( 155.9211002691896510, -4.999999999999989342, -2.071067811865468400 ) ) ;
#19033=CARTESIAN_POINT ( 'NONE',  ( -9.999999999999765521, -90.00000000000001421, -3.000000000000002665 ) ) ;
#19034=VERTEX_POINT ( 'NONE', #20471 ) ;
#19037=DIRECTION ( 'NONE',  ( 0.000000000000000000, 0.000000000000000000, -1.000000000000000000 ) ) ;
#19042=DIRECTION ( 'NONE',  ( 1.000000000000000000, -3.469446951953694061E-16, -0.000000000000000000 ) ) ;
#19043=VECTOR ( 'NONE', #8225, 1000.000000000000000 ) ;
#19045=ORIENTED_EDGE ( 'NONE', *, *, #9883, .T. ) ;
#19046=CARTESIAN_POINT ( 'NONE',  ( 146.2500000000000568, -6.000000000000005329, 0.000000000000000000 ) ) ;
#19055=CIRCLE ( 'NONE', #12184, 1.000000000000000000 ) ;
#19057=ORIENTED_EDGE ( 'NONE', *, *, #28272, .T. ) ;
#19059=SURFACE_STYLE_FILL_AREA ( #23946 ) ;
#19065=VECTOR ( 'NONE', #29872, 1000.000000000000000 ) ;
#19067=EDGE_CURVE ( 'NONE', #15961, #2390, #18194, .T. ) ;
#19079=CARTESIAN_POINT ( 'NONE',  ( 157.3199251345948824, -2.278174593051950136, -5.500000000000074607 ) ) ;
#19082=CARTESIAN_POINT ( 'NONE',  ( 136.4062500000000568, 6.000000000000005329, -2.485281374238555774 ) ) ;
#19085=DIRECTION ( 'NONE',  ( 1.000000000000000000, -0.000000000000000000, -0.000000000000000000 ) ) ;
#19090=CARTESIAN_POINT ( 'NONE',  ( 8.673617379884035472E-16, -14.99923475244192339, 9.015151515151522688 ) ) ;
#19091=CARTESIAN_POINT ( 'NONE',  ( 136.3913997308104058, -2.071067811865468400, 4.999999999999989342 ) ) ;
#19100=DIRECTION ( 'NONE',  ( 0.000000000000000000, 1.000000000000000000, -1.224646799147353207E-16 ) ) ;
#19103=ORIENTED_EDGE ( 'NONE', *, *, #15498, .T. ) ;
#19105=CARTESIAN_POINT ( 'NONE',  ( 137.0625000000000284, -4.242640687119298093, 4.242640687119298093 ) ) ;
#19107=CARTESIAN_POINT ( 'NONE',  ( 138.4613248654052313, -5.500000000000005329, 0.000000000000000000 ) ) ;
#19109=CARTESIAN_POINT ( 'NONE',  ( 134.6250000000000284, 0.000000000000000000, -6.000000000000005329 ) ) ;
#19115=CARTESIAN_POINT ( 'NONE',  ( 140.5384615384615756, -11.07692307692306777, -4.615384615384604317 ) ) ;
#19118=CARTESIAN_POINT ( 'NONE',  ( -0.5000000000000007772, -10.00000000000000711, -4.414213562373099364 ) ) ;
#19120=LINE ( 'NONE', #502, #11880 ) ;
#19131=CARTESIAN_POINT ( 'NONE',  ( 157.9687500000000568, -2.485281374238585972, 6.000000000000005329 ) ) ;
#19135=ORIENTED_EDGE ( 'NONE', *, *, #1974, .F. ) ;
#19137=CARTESIAN_POINT ( 'NONE',  ( 152.7187500000000284, 2.485281374238555774, -6.000000000000005329 ) ) ;
#19142=DIRECTION ( 'NONE',  ( -1.000000000000000000, 0.000000000000000000, 0.000000000000000000 ) ) ;
#19146=ORIENTED_EDGE ( 'NONE', *, *, #2081, .F. ) ;
#19151=EDGE_LOOP ( 'NONE', ( #4345, #18069, #17484, #17233 ) ) ;
#19153=CARTESIAN_POINT ( 'NONE',  ( 156.3601497308104058, -3.535533905932725318, -3.535533905932725318 ) ) ;
#19156=MECHANICAL_DESIGN_GEOMETRIC_PRESENTATION_REPRESENTATION('',(#13788),#8864);
#19157=CARTESIAN_POINT ( 'NONE',  ( -4.999999999999990230, -24.99999999999999289, -4.000000000000003553 ) ) ;
#19167=CARTESIAN_POINT ( 'NONE',  ( 155.2648502691896510, 3.535533905932725318, 3.535533905932752852 ) ) ;
#19172=SURFACE_STYLE_FILL_AREA ( #3149 ) ;
#19176=CARTESIAN_POINT ( 'NONE',  ( -0.08335392965452037561, -15.22338135603291853, -7.695243043971561114 ) ) ;
#19183=( BOUNDED_SURFACE ( )  B_SPLINE_SURFACE ( 3, 2, ( 
 ( #6517, #20974, #25398 ),
 ( #25235, #2514, #19425 ),
 ( #14820, #28752, #24162 ),
 ( #665, #24015, #7721 ),
 ( #25868, #12377, #19276 ),
 ( #2660, #21725, #17129 ),
 ( #16689, #7286, #21423 ),
 ( #10047, #26455, #4958 ),
 ( #26011, #354, #14529 ),
 ( #5406, #3104, #5108 ),
 ( #2960, #12530, #21871 ),
 ( #811, #12083, #18828 ) ),
 .UNSPECIFIED., .F., .F., .T. ) 
 B_SPLINE_SURFACE_WITH_KNOTS ( ( 4, 2, 2, 2, 2, 4 ),
 ( 3, 3 ),
 ( 0.0005482801588371855397, 0.001000919478279807106, 0.001227239138001117889, 0.001453558797722428672, 0.001906198117165050238, 0.002358837436607671804 ),
 ( 0.000000000000000000, 1.000000000000000000 ),
 .UNSPECIFIED. ) 
 GEOMETRIC_REPRESENTATION_ITEM ( )  RATIONAL_B_SPLINE_SURFACE ( (
 ( 1.000000000000000000, 0.9165151389911680990, 1.000000000000000000),
 ( 1.000000000000000000, 0.9166361146696374584, 1.000000000000000000),
 ( 1.000000000000000000, 0.9090514103963388548, 1.000000000000000000),
 ( 1.000000000000000000, 0.8902690042825124328, 1.000000000000000000),
 ( 1.000000000000000000, 0.8826973805417798191, 1.000000000000000000),
 ( 1.000000000000000000, 0.8660311221766173739, 1.000000000000000000),
 ( 1.000000000000000000, 0.8568659817695165604, 1.000000000000000000),
 ( 1.000000000000000000, 0.8270719941331442504, 1.000000000000000000),
 ( 1.000000000000000000, 0.8050517830292033272, 1.000000000000000000),
 ( 1.000000000000000000, 0.7576724516402112419, 1.000000000000000000),
 ( 1.000000000000000000, 0.7325062753274510507, 1.000000000000000000),
 ( 1.000000000000000000, 0.7071067811865453523, 1.000000000000000000) ) ) 
 REPRESENTATION_ITEM ( '' )  SURFACE ( )  );
#19186=UNCERTAINTY_MEASURE_WITH_UNIT (LENGTH_MEASURE( 1.000000000000000082E-05 ), #18415, 'distance_accuracy_value', 'NONE');
#19192=CARTESIAN_POINT ( 'NONE',  ( 0.2066402860832207145, -15.46612969915937086, -8.189149229532207031 ) ) ;
#19199=DIRECTION ( 'NONE',  ( 1.000000000000000000, -0.000000000000000000, -0.000000000000000000 ) ) ;
#19201=CYLINDRICAL_SURFACE ( 'NONE', #25174, 5.500000000000000000 ) ;
#19203=COLOUR_RGB ( '', 0.40784314, 0.44705882, 0.49803922) ;
#19210=COLOUR_RGB ( '', 0.31764706, 0.68627451, 0.89019608) ;
#19211=DIRECTION ( 'NONE',  ( -1.000000000000000000, 0.000000000000000000, 0.000000000000000000 ) ) ;
#19217=ORIENTED_EDGE ( 'NONE', *, *, #18120, .T. ) ;
#19220=CARTESIAN_POINT ( 'NONE',  ( 134.9211002691897079, -4.999999999999989342, -2.071067811865468400 ) ) ;
#19228=CARTESIAN_POINT ( 'NONE',  ( 144.1949251345948255, 5.500000000000012434, -2.278174593052012309 ) ) ;
#19229=ORIENTED_EDGE ( 'NONE', *, *, #24816, .F. ) ;
#19232=CARTESIAN_POINT ( 'NONE',  ( 149.6324251345948539, -5.500000000000012434, -2.278174593052012309 ) ) ;
#19233=CARTESIAN_POINT ( 'NONE',  ( 135.5476497308104058, 0.000000000000000000, -5.000000000000004441 ) ) ;
#19237=AXIS2_PLACEMENT_3D ( 'NONE', #4596, #11405, #9065 ) ;
#19240=( BOUNDED_CURVE ( )  B_SPLINE_CURVE ( 2, ( #903, #21682, #28261, #19228, #10003, #28702, #21825, #7240, #26411 ),
 .UNSPECIFIED., .F., .F. ) 
 B_SPLINE_CURVE_WITH_KNOTS ( ( 3, 2, 2, 2, 3 ),
 ( 0.3874999999999999001, 0.3937499999999997669, 0.3999999999999994671, 0.4062499999999992228, 0.4124999999999989786 ),
 .UNSPECIFIED. ) 
 CURVE ( )  GEOMETRIC_REPRESENTATION_ITEM ( )  RATIONAL_B_SPLINE_CURVE ( ( 1.000000000000000666, 0.9238795325112860723, 1.000000000000000000, 0.9238795325112867385, 1.000000000000000000, 0.9238795325112867385, 1.000000000000000000, 0.9238795325112989509, 0.9999999999999877875 ) ) 
 REPRESENTATION_ITEM ( '' )  );
#19245=VECTOR ( 'NONE', #12698, 1000.000000000000000 ) ;
#19248=ORIENTED_EDGE ( 'NONE', *, *, #15240, .F. ) ;
#19254=( LENGTH_UNIT ( ) NAMED_UNIT ( * ) SI_UNIT ( .MILLI., .METRE. ) );
#19255=CARTESIAN_POINT ( 'NONE',  ( 134.9062500000000284, 6.000000000000005329, -2.485281374238555774 ) ) ;
#19268=CARTESIAN_POINT ( 'NONE',  ( 152.6324251345948824, -5.500000000000012434, -2.278174593052012309 ) ) ;
#19269=AXIS2_PLACEMENT_3D ( 'NONE', #8156, #3099, #8014 ) ;
#19276=CARTESIAN_POINT ( 'NONE',  ( 139.7755489643691078, -9.313758021888212113, 7.918536325242551577 ) ) ;
#19283=CARTESIAN_POINT ( 'NONE',  ( 145.7961002691896510, 2.071067811865468400, -4.999999999999989342 ) ) ;
#19284=CARTESIAN_POINT ( 'NONE',  ( 151.2187500000000000, 2.485281374238556218, -6.000000000000005329 ) ) ;
#19286=ADVANCED_FACE ( 'NONE', ( #21240 ), #11450, .F. ) ;
#19288=AXIS2_PLACEMENT_3D ( 'NONE', #16058, #19, #16505 ) ;
#19289=EDGE_LOOP ( 'NONE', ( #25455, #19651, #29007, #9840, #9198, #29915, #10728, #26692 ) ) ;
#19290=CARTESIAN_POINT ( 'NONE',  ( 149.5312500000000284, -2.485281374238555774, -6.000000000000005329 ) ) ;
#19291=UNCERTAINTY_MEASURE_WITH_UNIT (LENGTH_MEASURE( 1.000000000000000082E-05 ), #16842, 'distance_accuracy_value', 'NONE');
#19292=ADVANCED_FACE ( 'NONE', ( #9103 ), #16362, .F. ) ;
#19297=ORIENTED_EDGE ( 'NONE', *, *, #14420, .T. ) ;
#19300=VERTEX_POINT ( 'NONE', #25683 ) ;
#19301=CARTESIAN_POINT ( 'NONE',  ( 124.9999999999999432, -70.00000000000000000, -5.000000000000004441 ) ) ;
#19312=CARTESIAN_POINT ( 'NONE',  ( 149.3363248654052029, 0.000000000000000000, -5.500000000000005329 ) ) ;
#19317=CARTESIAN_POINT ( 'NONE',  ( 158.2648502691896510, 3.535533905932725318, 3.535533905932752852 ) ) ;
#19323=ADVANCED_FACE ( 'NONE', ( #11748 ), #15559, .F. ) ;
#19324=CARTESIAN_POINT ( 'NONE',  ( -15.49999999999999289, -54.99999999999990763, 8.000000000000007105 ) ) ;
#19325=EDGE_CURVE ( 'NONE', #7800, #17999, #10108, .T. ) ;
#19327=LINE ( 'NONE', #26357, #4801 ) ;
#19330=VERTEX_POINT ( 'NONE', #7094 ) ;
#19331=CIRCLE ( 'NONE', #23268, 1.000000000000000000 ) ;
#19333=( GEOMETRIC_REPRESENTATION_CONTEXT ( 3 ) GLOBAL_UNCERTAINTY_ASSIGNED_CONTEXT ( ( #17714 ) ) GLOBAL_UNIT_ASSIGNED_CONTEXT ( ( #17303, #29965, #12550 ) ) REPRESENTATION_CONTEXT ( 'NONE', 'WORKASPACE' ) );
#19342=CARTESIAN_POINT ( 'NONE',  ( 133.6726497308104058, -5.000000000000004441, 0.000000000000000000 ) ) ;
#19344=VERTEX_POINT ( 'NONE', #23550 ) ;
#19345=CYLINDRICAL_SURFACE ( 'NONE', #21109, 0.5000000000000004441 ) ;
#19347=CARTESIAN_POINT ( 'NONE',  ( 141.6488248654052029, -3.889087296526011706, -3.889087296526011706 ) ) ;
#19354=CARTESIAN_POINT ( 'NONE',  ( 135.1170067730392361, -7.914203246654652801, 8.323901939971086961 ) ) ;
#19356=PRESENTATION_STYLE_ASSIGNMENT (( #29984 ) ) ;
#19358=CARTESIAN_POINT ( 'NONE',  ( 149.1636751345948255, 0.000000000000000000, 5.500000000000005329 ) ) ;
#19359=ORIENTED_EDGE ( 'NONE', *, *, #4238, .T. ) ;
#19360=CARTESIAN_POINT ( 'NONE',  ( 0.07046192191372500913, -16.32887961881856853, 6.302507423776497752 ) ) ;
#19363=EDGE_CURVE ( 'NONE', #6339, #29963, #5686, .T. ) ;
#19367=VERTEX_POINT ( 'NONE', #10169 ) ;
#19372=DIRECTION ( 'NONE',  ( 0.000000000000000000, 0.000000000000000000, 1.000000000000000000 ) ) ;
#19373=CARTESIAN_POINT ( 'NONE',  ( 134.3586002691896510, 2.071067811865468400, 4.999999999999989342 ) ) ;
#19375=FACE_OUTER_BOUND ( 'NONE', #14481, .T. ) ;
#19377=CARTESIAN_POINT ( 'NONE',  ( 161.0000000000000284, 0.000000000000000000, 0.000000000000000000 ) ) ;
#19379=ORIENTED_EDGE ( 'NONE', *, *, #26197, .F. ) ;
#19382=CARTESIAN_POINT ( 'NONE',  ( 149.5386751345948539, -5.500000000000005329, 0.000000000000000000 ) ) ;
#19383=CARTESIAN_POINT ( 'NONE',  ( 137.8913997308104058, -2.071067811865468400, 4.999999999999989342 ) ) ;
#19398=CARTESIAN_POINT ( 'NONE',  ( 153.3675748654052597, -5.500000000000012434, 2.278174593052012309 ) ) ;
#19402=DIRECTION ( 'NONE',  ( 0.000000000000000000, 0.000000000000000000, 1.000000000000000000 ) ) ;
#19406=VECTOR ( 'NONE', #16783, 1000.000000000000000 ) ;
#19411=AXIS2_PLACEMENT_3D ( 'NONE', #8690, #16255, #30334 ) ;
#19418=CARTESIAN_POINT ( 'NONE',  ( -4.999999999999990230, -14.50000000000001243, 7.500000000000007105 ) ) ;
#19421=CARTESIAN_POINT ( 'NONE',  ( 140.6985356443576620, -11.69853564435973503, -4.029618091915715183 ) ) ;
#19425=CARTESIAN_POINT ( 'NONE',  ( 139.5759038609257061, -9.165151425709554545, 8.000000000000007105 ) ) ;
#19430=EDGE_CURVE ( 'NONE', #10447, #3203, #23576, .T. ) ;
#19433=CYLINDRICAL_SURFACE ( 'NONE', #28273, 17.50000000000000355 ) ;
#19434=CARTESIAN_POINT ( 'NONE',  ( 146.4523502691896510, 0.000000000000000000, 5.000000000000004441 ) ) ;
#19435=CARTESIAN_POINT ( 'NONE',  ( 149.7187500000000284, 2.485281374238556218, -6.000000000000005329 ) ) ;
#19441=( NAMED_UNIT ( * ) SI_UNIT ( $, .STERADIAN. ) SOLID_ANGLE_UNIT ( ) );
#19442=ORIENTED_EDGE ( 'NONE', *, *, #5382, .F. ) ;
#19443=CARTESIAN_POINT ( 'NONE',  ( 142.1250000000000284, 0.000000000000000000, -6.000000000000005329 ) ) ;
#19445=COLOUR_RGB ( '', 0.66274510, 0.83137255, 0.94901961) ;
#19455=CARTESIAN_POINT ( 'NONE',  ( 135.1084928141470414, -8.790281914036096822, 8.000000000000007105 ) ) ;
#19465=CARTESIAN_POINT ( 'NONE',  ( 157.2336002691896226, -4.999999999999989342, 2.071067811865468400 ) ) ;
#19471=CARTESIAN_POINT ( 'NONE',  ( -4.999999999999879208, -71.00000000000002842, 5.000000000000004441 ) ) ;
#19476=ORIENTED_EDGE ( 'NONE', *, *, #9715, .T. ) ;
#19483=CARTESIAN_POINT ( 'NONE',  ( -9.999999999999793943, 10.00000000000000888, -3.000000000000002665 ) ) ;
#19486=AXIS2_PLACEMENT_3D ( 'NONE', #19550, #22150, #21850 ) ;
#19487=CARTESIAN_POINT ( 'NONE',  ( 132.0788997308104058, -4.999999999999989342, 2.071067811865468400 ) ) ;
#19488=EDGE_CURVE ( 'NONE', #1706, #28330, #296, .T. ) ;
#19491=CARTESIAN_POINT ( 'NONE',  ( 0.8055949159889823630, -15.44753772930997116, -8.223435417591852925 ) ) ;
#19498=DIRECTION ( 'NONE',  ( 0.000000000000000000, 0.4000000000000005773, -0.9165151389911678770 ) ) ;
#19502=( NAMED_UNIT ( * ) PLANE_ANGLE_UNIT ( ) SI_UNIT ( $, .RADIAN. ) );
#19504=DIRECTION ( 'NONE',  ( 1.000000000000000000, 0.000000000000000000, 0.000000000000000000 ) ) ;
#19509=TOROIDAL_SURFACE ( 'NONE', #10681, 16.00000000000000000, 1.000000000000000000 ) ;
#19511=VERTEX_POINT ( 'NONE', #4301 ) ;
#19512=PRESENTATION_STYLE_ASSIGNMENT (( #7224 ) ) ;
#19517=VECTOR ( 'NONE', #29485, 1000.000000000000000 ) ;
#19521=CARTESIAN_POINT ( 'NONE',  ( 134.0773502691896510, 5.000000000000004441, 0.000000000000000000 ) ) ;
#19525=DIRECTION ( 'NONE',  ( 1.000000000000000000, -0.000000000000000000, -0.000000000000000000 ) ) ;
#19526=ORIENTED_EDGE ( 'NONE', *, *, #7096, .F. ) ;
#19527=CIRCLE ( 'NONE', #3796, 1.000000000000000000 ) ;
#19531=CARTESIAN_POINT ( 'NONE',  ( 116.0000000000000142, 0.000000000000000000, 0.000000000000000000 ) ) ;
#19532=CARTESIAN_POINT ( 'NONE',  ( 136.8601497308104058, -3.535533905932725318, -3.535533905932725318 ) ) ;
#19534=LINE ( 'NONE', #10010, #1118 ) ;
#19542=CARTESIAN_POINT ( 'NONE',  ( 159.0000000000000284, -59.99999999999980105, 3.000000000000002665 ) ) ;
#19543=CARTESIAN_POINT ( 'NONE',  ( 153.6488248654052029, -3.889087296526011706, -3.889087296526011706 ) ) ;
#19547=MECHANICAL_DESIGN_GEOMETRIC_PRESENTATION_REPRESENTATION('',(#11728),#12214);
#19550=CARTESIAN_POINT ( 'NONE',  ( 161.0000000000000284, 0.000000000000000000, 0.000000000000000000 ) ) ;
#19553=EDGE_CURVE ( 'NONE', #9311, #6732, #29710, .T. ) ;
#19562=ADVANCED_FACE ( 'NONE', ( #21658 ), #6194, .F. ) ;
#19565=FILL_AREA_STYLE ('',( #2955 ) ) ;
#19574=ORIENTED_EDGE ( 'NONE', *, *, #3218, .T. ) ;
#19575=CARTESIAN_POINT ( 'NONE',  ( 141.4836002691896510, 4.999999999999989342, -2.071067811865468400 ) ) ;
#19576=CARTESIAN_POINT ( 'NONE',  ( 149.3437500000000284, -6.000000000000005329, -2.485281374238556218 ) ) ;
#19580=ORIENTED_EDGE ( 'NONE', *, *, #7275, .F. ) ;
#19581=CARTESIAN_POINT ( 'NONE',  ( 146.4375000000000284, -4.242640687119298093, -4.242640687119298093 ) ) ;
#19582=EDGE_CURVE ( 'NONE', #16955, #11567, #2569, .T. ) ;
#19584=LINE ( 'NONE', #17299, #1569 ) ;
#19589=FACE_OUTER_BOUND ( 'NONE', #18402, .T. ) ;
#19596=FILL_AREA_STYLE_COLOUR ( '', #18170 ) ;
#19597=CARTESIAN_POINT ( 'NONE',  ( 135.2945438920438903, -8.600858288651318517, 8.000000000000007105 ) ) ;
#19599=DIRECTION ( 'NONE',  ( -1.000000000000000000, -1.067522139062651904E-16, -0.000000000000000000 ) ) ;
#19601=CARTESIAN_POINT ( 'NONE',  ( 135.0000000000000284, -8.500000000000007105, -7.500000000000007105 ) ) ;
#19604=SURFACE_SIDE_STYLE ('',( #15479 ) ) ;
#19606=AXIS2_PLACEMENT_3D ( 'NONE', #15677, #11205, #17970 ) ;
#19611=CARTESIAN_POINT ( 'NONE',  ( 160.2187500000000000, 2.485281374238555774, -6.000000000000005329 ) ) ;
#19626=ORIENTED_EDGE ( 'NONE', *, *, #29347, .T. ) ;
#19629=CARTESIAN_POINT ( 'NONE',  ( 135.0000000000000568, -8.128079051996127902, 7.787350685426587482 ) ) ;
#19631=VECTOR ( 'NONE', #15407, 1000.000000000000000 ) ;
#19634=CARTESIAN_POINT ( 'NONE',  ( 0.1148264294874666441, -15.24996949206075314, -8.589764806507680817 ) ) ;
#19637=( LENGTH_UNIT ( ) NAMED_UNIT ( * ) SI_UNIT ( .MILLI., .METRE. ) );
#19641=CARTESIAN_POINT ( 'NONE',  ( -6.110151747003138060E-09, -9.999999993889911565, 4.800749288174370299 ) ) ;
#19647=EDGE_LOOP ( 'NONE', ( #29918, #9419, #3943, #8008 ) ) ;
#19649=CARTESIAN_POINT ( 'NONE',  ( 0.8631338372297875372, -15.37878787878788067, -8.351220472436777342 ) ) ;
#19651=ORIENTED_EDGE ( 'NONE', *, *, #26865, .T. ) ;
#19654=EDGE_CURVE ( 'NONE', #2429, #28218, #13104, .T. ) ;
#19655=( NAMED_UNIT ( * ) PLANE_ANGLE_UNIT ( ) SI_UNIT ( $, .RADIAN. ) );
#19656=ORIENTED_EDGE ( 'NONE', *, *, #14744, .F. ) ;
#19657=DIRECTION ( 'NONE',  ( 1.000000000000000000, 0.000000000000000000, 0.000000000000000000 ) ) ;
#19660=CARTESIAN_POINT ( 'NONE',  ( 161.2500000000000284, -6.000000000000005329, 0.000000000000000000 ) ) ;
#19663=CARTESIAN_POINT ( 'NONE',  ( 160.0000000000000284, 0.000000000000000000, 0.000000000000000000 ) ) ;
#19666=COLOUR_RGB ( '', 0.40784314, 0.44705882, 0.49803922) ;
#19669=CARTESIAN_POINT ( 'NONE',  ( 8.673617379884035472E-16, -15.50000000000001421, -5.656854249492387687 ) ) ;
#19672=CARTESIAN_POINT ( 'NONE',  ( 136.7663997308104058, -4.999999999999989342, -2.071067811865468400 ) ) ;
#19673=CARTESIAN_POINT ( 'NONE',  ( 137.3363248654052029, 0.000000000000000000, -5.500000000000005329 ) ) ;
#19674=CARTESIAN_POINT ( 'NONE',  ( -0.04562205425673532266, -14.50000000000001243, -8.291335958003946516 ) ) ;
#19677=CARTESIAN_POINT ( 'NONE',  ( 135.0000000000000568, 2.227365967767792831, 5.061342792685060488 ) ) ;
#19679=PLANE ( 'NONE',  #11331 ) ;
#19682=DIRECTION ( 'NONE',  ( -1.000000000000000000, -0.000000000000000000, 0.000000000000000000 ) ) ;
#19683=CARTESIAN_POINT ( 'NONE',  ( 154.1324251345948539, -5.500000000000012434, -2.278174593052012309 ) ) ;
#19688=CARTESIAN_POINT ( 'NONE',  ( -10.00000000000000178, -19.99999999999998934, 4.000000000000003553 ) ) ;
#19690=ORIENTED_EDGE ( 'NONE', *, *, #8732, .T. ) ;
#19697=CARTESIAN_POINT ( 'NONE',  ( 116.0000000000000142, 0.000000000000000000, 0.000000000000000000 ) ) ;
#19705=CARTESIAN_POINT ( 'NONE',  ( 156.6413997308104342, 2.071067811865468400, -4.999999999999989342 ) ) ;
#19708=VECTOR ( 'NONE', #20785, 1000.000000000000000 ) ;
#19711=CARTESIAN_POINT ( 'NONE',  ( 159.0000000000000284, -11.07692307692306777, -4.615384615384604317 ) ) ;
#19713=CARTESIAN_POINT ( 'NONE',  ( 140.0000000000000284, -54.99999999999990763, 8.000000000000007105 ) ) ;
#19718=CARTESIAN_POINT ( 'NONE',  ( 153.6562500000000568, -6.000000000000005329, 2.485281374238556218 ) ) ;
#19720=CIRCLE ( 'NONE', #23664, 9.999999999999996447 ) ;
#19722=ADVANCED_FACE ( 'NONE', ( #12761 ), #1652, .T. ) ;
#19724=CARTESIAN_POINT ( 'NONE',  ( 144.0000000000000284, 6.000000000000005329, 0.000000000000000000 ) ) ;
#19728=ORIENTED_EDGE ( 'NONE', *, *, #6618, .F. ) ;
#19732=CARTESIAN_POINT ( 'NONE',  ( 116.0000000000000142, 0.000000000000000000, -5.500000000000000000 ) ) ;
#19733=PRESENTATION_STYLE_ASSIGNMENT (( #10380 ) ) ;
#19735=CARTESIAN_POINT ( 'NONE',  ( 140.0000000000000284, -11.45643923738959202, -5.000000000000004441 ) ) ;
#19741=CARTESIAN_POINT ( 'NONE',  ( 135.0000000000000000, 5.116053516637836474, 2.738964164488275621 ) ) ;
#19746=DIRECTION ( 'NONE',  ( 0.000000000000000000, 0.000000000000000000, 1.000000000000000000 ) ) ;
#19747=CARTESIAN_POINT ( 'NONE',  ( 151.2336002691896510, -4.999999999999989342, 2.071067811865468400 ) ) ;
#19749=CARTESIAN_POINT ( 'NONE',  ( 161.4187058191337769, -3.655040188723187367, -4.674867660659138835 ) ) ;
#19755=( GEOMETRIC_REPRESENTATION_CONTEXT ( 3 ) GLOBAL_UNCERTAINTY_ASSIGNED_CONTEXT ( ( #2596 ) ) GLOBAL_UNIT_ASSIGNED_CONTEXT ( ( #27730, #10893, #23006 ) ) REPRESENTATION_CONTEXT ( 'NONE', 'WORKASPACE' ) );
#19757=CARTESIAN_POINT ( 'NONE',  ( 159.1875000000000284, 4.242640687119269671, 4.242640687119298093 ) ) ;
#19759=CARTESIAN_POINT ( 'NONE',  ( -4.999999999999886313, -69.50000000000001421, 8.000000000000007105 ) ) ;
#19765=( GEOMETRIC_REPRESENTATION_CONTEXT ( 3 ) GLOBAL_UNCERTAINTY_ASSIGNED_CONTEXT ( ( #18880 ) ) GLOBAL_UNIT_ASSIGNED_CONTEXT ( ( #2670, #16701, #25875 ) ) REPRESENTATION_CONTEXT ( 'NONE', 'WORKASPACE' ) );
#19766=ORIENTED_EDGE ( 'NONE', *, *, #26197, .T. ) ;
#19771=ORIENTED_EDGE ( 'NONE', *, *, #20815, .T. ) ;
#19775=CARTESIAN_POINT ( 'NONE',  ( 155.6175748654052313, 5.500000000000012434, -2.278174593052012309 ) ) ;
#19778=CARTESIAN_POINT ( 'NONE',  ( 152.8050748654052029, 5.500000000000012434, 2.278174593052012309 ) ) ;
#19780=CARTESIAN_POINT ( 'NONE',  ( 155.3363248654052313, 0.000000000000000000, -5.500000000000005329 ) ) ;
#19781=ADVANCED_FACE ( 'NONE', ( #1180 ), #13009, .T. ) ;
#19783=PRESENTATION_STYLE_ASSIGNMENT (( #3331 ) ) ;
#19785=SURFACE_STYLE_USAGE ( .BOTH. , #12912 ) ;
#19796=AXIS2_PLACEMENT_3D ( 'NONE', #21054, #30401, #28083 ) ;
#19798=CARTESIAN_POINT ( 'NONE',  ( 0.000000000000000000, 0.000000000000000000, 0.000000000000000000 ) ) ;
#19803=CARTESIAN_POINT ( 'NONE',  ( 161.6250000000000568, 0.000000000000000000, -6.000000000000005329 ) ) ;
#19808=CARTESIAN_POINT ( 'NONE',  ( 135.6566535407617948, -9.123793365789314436, -8.000000000000007105 ) ) ;
#19810=VERTEX_POINT ( 'NONE', #2273 ) ;
#19813=FILL_AREA_STYLE ('',( #21976 ) ) ;
#19821=ADVANCED_FACE ( 'NONE', ( #25612 ), #26498, .T. ) ;
#19824=FILL_AREA_STYLE ('',( #24423 ) ) ;
#19825=ORIENTED_EDGE ( 'NONE', *, *, #6081, .T. ) ;
#19826=DIRECTION ( 'NONE',  ( 1.000000000000000000, 1.067522139062651904E-16, -0.000000000000000000 ) ) ;
#19830=CARTESIAN_POINT ( 'NONE',  ( 153.2738248654052313, -3.889087296526011706, 3.889087296526011706 ) ) ;
#19837=LINE ( 'NONE', #14942, #19024 ) ;
#19839=CARTESIAN_POINT ( 'NONE',  ( 161.0000000000000284, 0.000000000000000000, 0.000000000000000000 ) ) ;
#19841=ORIENTED_EDGE ( 'NONE', *, *, #6887, .T. ) ;
#19848=CARTESIAN_POINT ( 'NONE',  ( 149.9851497308104342, -3.535533905932725318, 3.535533905932725318 ) ) ;
#19852=SURFACE_STYLE_USAGE ( .BOTH. , #26598 ) ;
#19854=CARTESIAN_POINT ( 'NONE',  ( 135.0781295278050322, -7.870998221347940138, 8.267028835410057397 ) ) ;
#19855=EDGE_CURVE ( 'NONE', #28218, #22758, #10096, .T. ) ;
#19863=FACE_OUTER_BOUND ( 'NONE', #10636, .T. ) ;
#19865=CARTESIAN_POINT ( 'NONE',  ( 153.0937500000000284, 6.000000000000005329, 2.485281374238585972 ) ) ;
#19866=FACE_OUTER_BOUND ( 'NONE', #2172, .T. ) ;
#19871=CARTESIAN_POINT ( 'NONE',  ( 145.4062500000000284, 6.000000000000005329, -2.485281374238555774 ) ) ;
#19872=CARTESIAN_POINT ( 'NONE',  ( 161.1460176603489458, -1.573196579648956872, 5.431622084658472183 ) ) ;
#19873=ORIENTED_EDGE ( 'NONE', *, *, #23661, .F. ) ;
#19874=AXIS2_PLACEMENT_3D ( 'NONE', #9456, #10323, #21582 ) ;
#19883=( BOUNDED_CURVE ( )  B_SPLINE_CURVE ( 2, ( #21933, #867, #7933, #17344, #26659, #8075, #17493, #26805, #5771 ),
 .UNSPECIFIED., .F., .T. ) 
 B_SPLINE_CURVE_WITH_KNOTS ( ( 3, 2, 2, 2, 3 ),
 ( 0.4875000000000000444, 0.4937499999999998002, 0.4999999999999995559, 0.5062499999999993117, 0.5124999999999990674 ),
 .UNSPECIFIED. ) 
 CURVE ( )  GEOMETRIC_REPRESENTATION_ITEM ( )  RATIONAL_B_SPLINE_CURVE ( ( 1.000000000000000000, 0.9238795325112867385, 1.000000000000000000, 0.9238795325112867385, 1.000000000000000000, 0.9238795325112867385, 1.000000000000000000, 0.9238795325112975076, 0.9999999999999892308 ) ) 
 REPRESENTATION_ITEM ( '' )  );
#19885=CYLINDRICAL_SURFACE ( 'NONE', #13306, 5.500000000000000000 ) ;
#19887=CARTESIAN_POINT ( 'NONE',  ( -14.99999999999999289, -54.99999999999990763, 8.000000000000007105 ) ) ;
#19891=FACE_OUTER_BOUND ( 'NONE', #24575, .T. ) ;
#19894=CARTESIAN_POINT ( 'NONE',  ( 137.4449251345948255, -5.500000000000012434, 2.278174593052012309 ) ) ;
#19896=UNCERTAINTY_MEASURE_WITH_UNIT (LENGTH_MEASURE( 1.000000000000000082E-05 ), #13024, 'distance_accuracy_value', 'NONE');
#19898=DIRECTION ( 'NONE',  ( 0.000000000000000000, 0.000000000000000000, -1.000000000000000000 ) ) ;
#19902=CARTESIAN_POINT ( 'NONE',  ( 151.9836002691896226, 4.999999999999989342, -2.071067811865468400 ) ) ;
#19903=CARTESIAN_POINT ( 'NONE',  ( 161.2178144456196378, -4.907762444546311720, -2.963993361882520272 ) ) ;
#19904=CARTESIAN_POINT ( 'NONE',  ( 135.1011751345948539, 3.889087296526011706, -3.889087296526011706 ) ) ;
#19909=CARTESIAN_POINT ( 'NONE',  ( 161.7187500000000000, 2.485281374238555774, -6.000000000000005329 ) ) ;
#19911=CARTESIAN_POINT ( 'NONE',  ( -19.49999999999998224, -25.00000000000010658, -8.000000000000007105 ) ) ;
#19930=CARTESIAN_POINT ( 'NONE',  ( 156.0863248654052597, 0.000000000000000000, 5.500000000000005329 ) ) ;
#19935=CARTESIAN_POINT ( 'NONE',  ( -1.000000000000001776, -9.000000000000005329, 4.000000000000005329 ) ) ;
#19939=CARTESIAN_POINT ( 'NONE',  ( -4.999999999999886313, -71.00000000000002842, -4.000000000000003553 ) ) ;
#19940=CARTESIAN_POINT ( 'NONE',  ( 135.4618192888269164, -8.932050916383428074, 8.000000000000005329 ) ) ;
#19944=CARTESIAN_POINT ( 'NONE',  ( 161.5000000000000853, -2.984449860524901688, -5.205099329504969674 ) ) ;
#19946=ORIENTED_EDGE ( 'NONE', *, *, #18958, .F. ) ;
#19948=CARTESIAN_POINT ( 'NONE',  ( 139.3050748654052313, 5.500000000000012434, 2.278174593052012309 ) ) ;
#19955=CARTESIAN_POINT ( 'NONE',  ( 155.5312500000000568, -2.485281374238555774, -6.000000000000005329 ) ) ;
#19956=EDGE_CURVE ( 'NONE', #12037, #22266, #25910, .T. ) ;
#19964=FACE_OUTER_BOUND ( 'NONE', #20301, .T. ) ;
#19973=CARTESIAN_POINT ( 'NONE',  ( 147.7574251345948255, -2.278174593051764951, 5.500000000000262013 ) ) ;
#19974=DIRECTION ( 'NONE',  ( -1.734723475976824844E-16, 1.000000000000000000, 0.000000000000000000 ) ) ;
#19977=( BOUNDED_SURFACE ( )  B_SPLINE_SURFACE ( 3, 2, ( 
 ( #10988, #29840, #2056 ),
 ( #8818, #6498, #25535 ),
 ( #15921, #11459, #30150 ),
 ( #9113, #25222, #22949 ),
 ( #1888, #30302, #11293 ),
 ( #6139, #18003, #22891 ),
 ( #15399, #22591, #29475 ),
 ( #1206, #10615, #8911 ),
 ( #13395, #12943, #1373 ),
 ( #17851, #1522, #10933 ),
 ( #20425, #15554, #29783 ),
 ( #22739, #20283, #1682 ),
 ( #8277, #11080, #8759 ),
 ( #25163, #20583, #4127 ) ),
 .UNSPECIFIED., .F., .F., .T. ) 
 B_SPLINE_SURFACE_WITH_KNOTS ( ( 4, 2, 2, 2, 2, 2, 4 ),
 ( 3, 3 ),
 ( 0.001367763536538648284, 0.002168948318176349387, 0.002569540708995199721, 0.002970133099814050055, 0.003370725490632900390, 0.003771317881451751158, 0.004572502663089452260 ),
 ( 0.000000000000000000, 1.000000000000000000 ),
 .UNSPECIFIED. ) 
 GEOMETRIC_REPRESENTATION_ITEM ( )  RATIONAL_B_SPLINE_SURFACE ( (
 ( 1.000000000000000000, 0.7071067811865475727, 1.000000000000000000),
 ( 1.000000000000000000, 0.7177463599871298783, 1.000000000000000000),
 ( 1.000000000000000000, 0.7309160594376725717, 1.000000000000000000),
 ( 1.000000000000000000, 0.7518982708267778481, 1.000000000000000000),
 ( 1.000000000000000000, 0.7589818330818417502, 1.000000000000000000),
 ( 1.000000000000000000, 0.7730316713029788955, 1.000000000000000000),
 ( 1.000000000000000000, 0.7800646516387804708, 1.000000000000000000),
 ( 1.000000000000000000, 0.7931882794879633325, 1.000000000000000000),
 ( 1.000000000000000000, 0.7993227671868792239, 1.000000000000000000),
 ( 1.000000000000000000, 0.8104421674205291026, 1.000000000000000000),
 ( 1.000000000000000000, 0.8154231620175333983, 1.000000000000000000),
 ( 1.000000000000000000, 0.8275153884601259557, 1.000000000000000000),
 ( 1.000000000000000000, 0.8321080538050803499, 1.000000000000000000),
 ( 1.000000000000000000, 0.8320502943378441651, 1.000000000000000000) ) ) 
 REPRESENTATION_ITEM ( '' )  SURFACE ( )  );
#19983=DIRECTION ( 'NONE',  ( 0.000000000000000000, 0.000000000000000000, -1.000000000000000000 ) ) ;
#19985=ORIENTED_EDGE ( 'NONE', *, *, #26629, .T. ) ;
#19988=FILL_AREA_STYLE_COLOUR ( '', #28180 ) ;
#19990=CARTESIAN_POINT ( 'NONE',  ( 140.0252556714799539, -11.51262782845630817, -4.739386388448244780 ) ) ;
#19991=CARTESIAN_POINT ( 'NONE',  ( 155.2574251345948255, -2.278174593051826236, 5.500000000000198064 ) ) ;
#19993=CARTESIAN_POINT ( 'NONE',  ( 140.8041911596567957, -11.60838231931457365, 4.059228028635632590 ) ) ;
#19994=CARTESIAN_POINT ( 'NONE',  ( 140.3437500000000284, -6.000000000000005329, -2.485281374238555774 ) ) ;
#19995=EDGE_CURVE ( 'NONE', #17372, #13456, #21315, .T. ) ;
#19998=CARTESIAN_POINT ( 'NONE',  ( 136.3988248654052313, 3.889087296526011706, 3.889087296526011706 ) ) ;
#20002=DIRECTION ( 'NONE',  ( 0.000000000000000000, 0.000000000000000000, 1.000000000000000000 ) ) ;
#20004=CARTESIAN_POINT ( 'NONE',  ( 148.8601497308104058, -3.535533905932725318, -3.535533905932725318 ) ) ;
#20005=CIRCLE ( 'NONE', #25899, 0.5000000000000004441 ) ;
#20006=DIRECTION ( 'NONE',  ( -0.2768592823360734867, 0.4367774878841467201, 0.8559055811606609554 ) ) ;
#20015=ORIENTED_EDGE ( 'NONE', *, *, #2585, .F. ) ;
#20020=DIRECTION ( 'NONE',  ( 0.000000000000000000, 1.000000000000000000, 0.000000000000000000 ) ) ;
#20023=CARTESIAN_POINT ( 'NONE',  ( 144.2812500000000284, 2.485281374238585972, 6.000000000000005329 ) ) ;
#20026=( LENGTH_UNIT ( ) NAMED_UNIT ( * ) SI_UNIT ( .MILLI., .METRE. ) );
#20028=VERTEX_POINT ( 'NONE', #17624 ) ;
#20029=CARTESIAN_POINT ( 'NONE',  ( 143.0625000000000284, -4.242640687119298093, 4.242640687119298093 ) ) ;
#20032=EDGE_CURVE ( 'NONE', #19810, #3216, #3534, .T. ) ;
#20045=CARTESIAN_POINT ( 'NONE',  ( -10.00000000000000178, -19.99999999999998934, -3.000000000000002665 ) ) ;
#20054=DIRECTION ( 'NONE',  ( 0.000000000000000000, 0.000000000000000000, -1.000000000000000000 ) ) ;
#20057=CARTESIAN_POINT ( 'NONE',  ( 150.8586002691896510, 2.071067811865468400, 4.999999999999989342 ) ) ;
#20058=DIRECTION ( 'NONE',  ( -1.000000000000000000, -0.000000000000000000, -0.000000000000000000 ) ) ;
#20059=CYLINDRICAL_SURFACE ( 'NONE', #14976, 1.000000000000000000 ) ;
#20069=EDGE_CURVE ( 'NONE', #8862, #20381, #14519, .T. ) ;
#20074=UNCERTAINTY_MEASURE_WITH_UNIT (LENGTH_MEASURE( 1.000000000000000082E-05 ), #1701, 'distance_accuracy_value', 'NONE');
#20080=CARTESIAN_POINT ( 'NONE',  ( 147.0863248654052313, 0.000000000000000000, 5.500000000000005329 ) ) ;
#20085=ORIENTED_EDGE ( 'NONE', *, *, #21297, .F. ) ;
#20087=CARTESIAN_POINT ( 'NONE',  ( 146.5386751345948539, -5.500000000000005329, 0.000000000000000000 ) ) ;
#20088=CARTESIAN_POINT ( 'NONE',  ( -4.999999999999886313, -70.00000000000001421, 7.500000000000007105 ) ) ;
#20092=CARTESIAN_POINT ( 'NONE',  ( -1.000000000000000888, 10.00000000000000888, -3.000000000000002665 ) ) ;
#20094=CARTESIAN_POINT ( 'NONE',  ( 160.0386751345948539, -5.500000000000005329, 0.000000000000000000 ) ) ;
#20096=( NAMED_UNIT ( * ) PLANE_ANGLE_UNIT ( ) SI_UNIT ( $, .RADIAN. ) );
#20097=CARTESIAN_POINT ( 'NONE',  ( 141.0074251345948255, 2.278174593051965235, -5.500000000000058620 ) ) ;
#20109=CARTESIAN_POINT ( 'NONE',  ( 149.8988248654052313, 3.889087296526011706, 3.889087296526011706 ) ) ;
#20112=EDGE_CURVE ( 'NONE', #28771, #16741, #13466, .T. ) ;
#20113=AXIS2_PLACEMENT_3D ( 'NONE', #24904, #25052, #1868 ) ;
#20114=ORIENTED_EDGE ( 'NONE', *, *, #22820, .T. ) ;
#20116=CARTESIAN_POINT ( 'NONE',  ( 157.5937500000000284, 6.000000000000005329, 2.485281374238585972 ) ) ;
#20121=DIRECTION ( 'NONE',  ( 0.000000000000000000, 0.000000000000000000, 1.000000000000000000 ) ) ;
#20125=CARTESIAN_POINT ( 'NONE',  ( 159.0865522212051815, -11.33333333501752982, 3.999999995034633216 ) ) ;
#20137=CARTESIAN_POINT ( 'NONE',  ( 148.3199251345948255, -2.278174593052012309, -5.500000000000012434 ) ) ;
#20139=AXIS2_PLACEMENT_3D ( 'NONE', #24293, #14126, #4549 ) ;
#20144=EDGE_CURVE ( 'NONE', #23494, #15499, #5362, .T. ) ;
#20148=CARTESIAN_POINT ( 'NONE',  ( 139.2336002691896510, -4.999999999999989342, 2.071067811865468400 ) ) ;
#20154=FACE_OUTER_BOUND ( 'NONE', #20843, .T. ) ;
#20155=ADVANCED_FACE ( 'NONE', ( #10715 ), #20059, .F. ) ;
#20159=CARTESIAN_POINT ( 'NONE',  ( 142.7812500000000568, 2.485281374238585972, 6.000000000000005329 ) ) ;
#20160=AXIS2_PLACEMENT_3D ( 'NONE', #9850, #12333, #18945 ) ;
#20161=ORIENTED_EDGE ( 'NONE', *, *, #11869, .T. ) ;
#20162=ORIENTED_EDGE ( 'NONE', *, *, #8515, .F. ) ;
#20163=CARTESIAN_POINT ( 'NONE',  ( 135.9300748654051745, 2.278174593051671692, -5.500000000000352607 ) ) ;
#20166=CARTESIAN_POINT ( 'NONE',  ( 135.8511751345948255, -3.889087296526011706, 3.889087296526011706 ) ) ;
#20171=CARTESIAN_POINT ( 'NONE',  ( 150.9226497308104058, 5.000000000000004441, 0.000000000000000000 ) ) ;
#20176=DIRECTION ( 'NONE',  ( 0.000000000000000000, 0.000000000000000000, 1.000000000000000000 ) ) ;
#20179=EDGE_CURVE ( 'NONE', #6130, #6918, #20361, .T. ) ;
#20184=ORIENTED_EDGE ( 'NONE', *, *, #13663, .T. ) ;
#20185=VECTOR ( 'NONE', #21482, 1000.000000000000000 ) ;
#20187=CARTESIAN_POINT ( 'NONE',  ( 146.0625000000000284, -4.242640687119298093, 4.242640687119298093 ) ) ;
#20189=AXIS2_PLACEMENT_3D ( 'NONE', #28528, #26235, #7497 ) ;
#20191=EDGE_CURVE ( 'NONE', #20568, #13841, #13635, .T. ) ;
#20194=CARTESIAN_POINT ( 'NONE',  ( 136.5937500000000853, 6.000000000000005329, 2.485281374238585972 ) ) ;
#20195=CARTESIAN_POINT ( 'NONE',  ( 161.2468146748790332, -4.679509648744853756, 3.350853646919034201 ) ) ;
#20198=VERTEX_POINT ( 'NONE', #23139 ) ;
#20201=ORIENTED_EDGE ( 'NONE', *, *, #15752, .F. ) ;
#20203=TOROIDAL_SURFACE ( 'NONE', #557, 14.49999999999999289, 0.5000000000000000000 ) ;
#20207=CARTESIAN_POINT ( 'NONE',  ( 125.0000000000000568, -55.00000000000000711, -7.500000000000007105 ) ) ;
#20209=CARTESIAN_POINT ( 'NONE',  ( 140.0769230769231228, -11.53846153846155254, -4.615384615384604317 ) ) ;
#20210=DIRECTION ( 'NONE',  ( 0.000000000000000000, 0.000000000000000000, -1.000000000000000000 ) ) ;
#20217=( BOUNDED_CURVE ( )  B_SPLINE_CURVE ( 2, ( #9741, #13779, #26006, #30318, #28149, #25706, #16536, #25551, #23120 ),
 .UNSPECIFIED., .F., .F. ) 
 B_SPLINE_CURVE_WITH_KNOTS ( ( 3, 2, 2, 2, 3 ),
 ( 0.7375000000000002665, 0.7437500000000000222, 0.7499999999999997780, 0.7562499999999995337, 0.7624999999999992895 ),
 .UNSPECIFIED. ) 
 CURVE ( )  GEOMETRIC_REPRESENTATION_ITEM ( )  RATIONAL_B_SPLINE_CURVE ( ( 0.9999999999999973355, 0.9238795325112894030, 1.000000000000000000, 0.9238795325112867385, 1.000000000000000000, 0.9238795325112867385, 1.000000000000000000, 0.9238795325112948431, 0.9999999999999918954 ) ) 
 REPRESENTATION_ITEM ( '' )  );
#20221=AXIS2_PLACEMENT_3D ( 'NONE', #4670, #11790, #23586 ) ;
#20222=CARTESIAN_POINT ( 'NONE',  ( 154.5148502691896510, -3.535533905932725318, -3.535533905932725318 ) ) ;
#20224=DIRECTION ( 'NONE',  ( 0.000000000000000000, 0.000000000000000000, -1.000000000000000000 ) ) ;
#20228=AXIS2_PLACEMENT_3D ( 'NONE', #15906, #4166, #15437 ) ;
#20230=EDGE_CURVE ( 'NONE', #13576, #7302, #26713, .T. ) ;
#20232=ORIENTED_EDGE ( 'NONE', *, *, #22403, .F. ) ;
#20233=SURFACE_STYLE_FILL_AREA ( #24353 ) ;
#20236=VECTOR ( 'NONE', #12246, 1000.000000000000000 ) ;
#20237=ORIENTED_EDGE ( 'NONE', *, *, #7025, .T. ) ;
#20247=CARTESIAN_POINT ( 'NONE',  ( 146.9136751345948539, 0.000000000000000000, -5.500000000000005329 ) ) ;
#20256=EDGE_CURVE ( 'NONE', #17671, #15465, #12072, .T. ) ;
#20260=VERTEX_POINT ( 'NONE', #27548 ) ;
#20264=( BOUNDED_CURVE ( )  B_SPLINE_CURVE ( 2, ( #19944, #20514, #29293, #17663, #5952, #29867, #16699, #4530, #12092, #26021, #21434, #366, #28318, #21280, #4969, #9298, #7296, #2240, #25575, #14251, #18840, #18995, #14404, #11642, #13955, #23296, #18690, #11794, #28465, #23738, #2668, #2384, #20988, #23589, #28166, #30335, #16105, #9755, #28012, #19131, #6985, #21135, #25408, #4369, #13797, #72, #16404, #219, #23141, #2086, #11490, #20831, #30179, #9457, #9145, #7136, #18537, #23445, #9605, #25728, #27864, #16554, #25874, #6830, #16256, #4673, #14109, #4826, #2526, #11953, #29064, #7433, #7576, #16989, #10214, #9908, #26748, #3258, #21583, #12689, #5117, #26313, #515, #12836, #17435, #19718, #8029, #22178, #3411, #17136, #10360, #19865, #26611, #26168, #22022, #17291, #2822, #26461, #2966, #818, #5417, #23877, #21880, #14829, #5715, #10511, #15126, #24172, #5566, #28606, #24457, #19284, #958, #1111, #12389, #16844, #14537, #12245, #5269, #24022, #14969, #3115, #14677, #21734, #673, #24309, #10059, #19435, #28760, #7728, #12537, #19576, #28911, #7877, #10834, #15288, #25221, #15609, #4189, #11130, #22642, #15452, #22492, #22331, #12994, #29839, #17744, #13604, #8817, #22948, #1887, #20478, #4028, #18202, #1425, #27520, #24778, #8334, #18056, #11292, #13153, #6497, #13300, #15920, #6193, #13447, #20187, #1265, #29210, #29539, #1581, #10987, #27068, #1735, #20332, #3563, #8172, #29683, #17589, #8496, #8655, #27371, #10676, #26905, #25071, #20023, #22795, #5869, #24613, #29370, #17902, #6334, #6033, #24922, #3724, #27219, #3872, #15764, #2204, #25534, #13760, #4792, #33, #16074, #9265, #16222, #14075, #18658, #4937, #9421, #14368, #28134, #4338, #25692, #16523, #6951, #25845, #11919, #23556, #18809, #4642, #6655, #23107, #30149, #7103, #27977, #16369, #14218, #23411, #2494, #9572, #23706, #21248, #16669, #2640, #28283, #20647, #18966, #25376, #189, #2055, #11458, #7261, #25992, #20802, #9112, #18358, #29993, #6798, #13920, #18507, #27830, #8969, #4497, #27675, #23263, #11609, #20950, #30301, #2356, #11759, #21104, #19105, #5533, #12506, #14646, #26285, #14939, #927, #28579, #9875, #481, #23993, #7696, #24431, #3224, #24277, #28725, #16957, #17257, #29034, #8000, #5681, #10326, #7408 ),
 .UNSPECIFIED., .F., .T. ) 
 B_SPLINE_CURVE_WITH_KNOTS ( ( 3, 2, 2, 2, 2, 2, 2, 2, 2, 2, 2, 2, 2, 2, 2, 2, 2, 2, 2, 2, 2, 2, 2, 2, 2, 2, 2, 2, 2, 2, 2, 2, 2, 2, 2, 2, 2, 2, 2, 2, 2, 2, 2, 2, 2, 2, 2, 2, 2, 2, 2, 2, 2, 2, 2, 2, 2, 2, 2, 2, 2, 2, 2, 2, 2, 2, 2, 2, 2, 2, 2, 2, 2, 2, 2, 2, 2, 2, 2, 2, 2, 2, 2, 2, 2, 2, 2, 2, 2, 2, 2, 2, 2, 2, 2, 2, 2, 2, 2, 2, 2, 2, 2, 2, 2, 2, 2, 2, 2, 2, 2, 2, 2, 2, 2, 2, 2, 2, 2, 2, 2, 2, 2, 2, 2, 2, 2, 2, 2, 2, 2, 2, 2, 2, 2, 2, 2, 2, 2, 2, 2, 2, 3 ),
 ( 0.01663113027555142287, 0.01874999999999999931, 0.02500000000000000139, 0.03125000000000000000, 0.03749999999999999861, 0.04374999999999999722, 0.05000000000000000278, 0.05625000000000000139, 0.06249999999999999306, 0.06875000000000000555, 0.07499999999999998335, 0.08125000000000000278, 0.08749999999999998057, 0.09375000000000000000, 0.09999999999999999167, 0.1062499999999999833, 0.1125000000000000028, 0.1187499999999999806, 0.1249999999999999861, 0.1312499999999999778, 0.1375000000000000111, 0.1437499999999999889, 0.1499999999999999667, 0.1562500000000000000, 0.1624999999999999778, 0.1687500000000000111, 0.1749999999999999889, 0.1812499999999999667, 0.1875000000000000000, 0.1937499999999999778, 0.2000000000000000111, 0.2062499999999999889, 0.2124999999999999667, 0.2187500000000000000, 0.2249999999999999778, 0.2312500000000000111, 0.2374999999999999889, 0.2437499999999999667, 0.2500000000000000000, 0.2562499999999999778, 0.2625000000000000111, 0.2687499999999999334, 0.2749999999999999667, 0.2812500000000000000, 0.2874999999999999223, 0.2937499999999999556, 0.2999999999999999889, 0.3062499999999999667, 0.3124999999999999445, 0.3187499999999999778, 0.3249999999999999556, 0.3312499999999999334, 0.3375000000000000222, 0.3437499999999999445, 0.3499999999999999223, 0.3562500000000000111, 0.3624999999999999334, 0.3687499999999999667, 0.3750000000000000000, 0.3812499999999999223, 0.3874999999999999556, 0.3937499999999999334, 0.3999999999999999667, 0.4062499999999999445, 0.4124999999999999223, 0.4187499999999999556, 0.4249999999999999334, 0.4312499999999999667, 0.4374999999999999445, 0.4437499999999999223, 0.4499999999999999556, 0.4562499999999999334, 0.4624999999999999667, 0.4687499999999999445, 0.4749999999999999223, 0.4812499999999999556, 0.4874999999999999334, 0.4937499999999999667, 0.4999999999999999445, 0.5062499999999999778, 0.5124999999999998446, 0.5187500000000000444, 0.5250000000000000222, 0.5312499999999998890, 0.5374999999999998668, 0.5437499999999999556, 0.5499999999999999334, 0.5562499999999999112, 0.5625000000000000000, 0.5687499999999998668, 0.5749999999999998446, 0.5812499999999999334, 0.5874999999999999112, 0.5937499999999998890, 0.5999999999999999778, 0.6062499999999998446, 0.6124999999999999334, 0.6187500000000000222, 0.6249999999999998890, 0.6312499999999998668, 0.6374999999999999556, 0.6437499999999999334, 0.6499999999999999112, 0.6562500000000000000, 0.6624999999999998668, 0.6687499999999998446, 0.6750000000000000444, 0.6812499999999999112, 0.6874999999999998890, 0.6937499999999998668, 0.6999999999999998446, 0.7062499999999999334, 0.7125000000000000222, 0.7187499999999998890, 0.7249999999999998668, 0.7312499999999998446, 0.7374999999999999334, 0.7437499999999999112, 0.7499999999999998890, 0.7562499999999998668, 0.7624999999999998446, 0.7687500000000000444, 0.7749999999999999112, 0.7812499999999998890, 0.7874999999999998668, 0.7937499999999998446, 0.7999999999999999334, 0.8062499999999999112, 0.8124999999999998890, 0.8187499999999998668, 0.8249999999999998446, 0.8312499999999999334, 0.8374999999999999112, 0.8437499999999998890, 0.8499999999999998668, 0.8562499999999998446, 0.8624999999999999334, 0.8687499999999999112, 0.8749999999999998890, 0.8812499999999998668, 0.8874999999999998446, 0.8937499999999999334, 0.8999999999999999112 ),
 .UNSPECIFIED. ) 
 CURVE ( )  GEOMETRIC_REPRESENTATION_ITEM ( )  RATIONAL_B_SPLINE_CURVE ( ( 0.9658850645339760455, 0.9741937033643669475, 1.000000000000000000, 0.9238795325112867385, 1.000000000000000000, 0.9238795325112867385, 1.000000000000000000, 0.9238795325112867385, 1.000000000000000000, 0.9238795325112867385, 1.000000000000000000, 0.9238795325112867385, 1.000000000000000000, 0.9238795325112867385, 1.000000000000000000, 0.9238795325112867385, 1.000000000000000000, 0.9238795325112867385, 1.000000000000000000, 0.9238795325112867385, 1.000000000000000000, 0.9238795325112867385, 1.000000000000000000, 0.9238795325112867385, 1.000000000000000000, 0.9238795325112867385, 1.000000000000000000, 0.9238795325112867385, 1.000000000000000000, 0.9238795325112867385, 1.000000000000000000, 0.9238795325112867385, 1.000000000000000000, 0.9238795325112867385, 1.000000000000000000, 0.9238795325112867385, 1.000000000000000000, 0.9238795325112867385, 1.000000000000000000, 0.9238795325112867385, 1.000000000000000000, 0.9238795325112867385, 1.000000000000000000, 0.9238795325112867385, 1.000000000000000000, 0.9238795325112867385, 1.000000000000000000, 0.9238795325112867385, 1.000000000000000000, 0.9238795325112867385, 1.000000000000000000, 0.9238795325112867385, 1.000000000000000000, 0.9238795325112867385, 1.000000000000000000, 0.9238795325112867385, 1.000000000000000000, 0.9238795325112867385, 1.000000000000000000, 0.9238795325112867385, 1.000000000000000000, 0.9238795325112867385, 1.000000000000000000, 0.9238795325112867385, 1.000000000000000000, 0.9238795325112867385, 1.000000000000000000, 0.9238795325112867385, 1.000000000000000000, 0.9238795325112867385, 1.000000000000000000, 0.9238795325112867385, 1.000000000000000000, 0.9238795325112867385, 1.000000000000000000, 0.9238795325112867385, 1.000000000000000000, 0.9238795325112867385, 1.000000000000000000, 0.9238795325112867385, 1.000000000000000000, 0.9238795325112867385, 1.000000000000000000, 0.9238795325112867385, 1.000000000000000000, 0.9238795325112867385, 1.000000000000000000, 0.9238795325112867385, 1.000000000000000000, 0.9238795325112867385, 1.000000000000000000, 0.9238795325112867385, 1.000000000000000000, 0.9238795325112867385, 1.000000000000000000, 0.9238795325112867385, 1.000000000000000000, 0.9238795325112867385, 1.000000000000000000, 0.9238795325112867385, 1.000000000000000000, 0.9238795325112867385, 1.000000000000000000, 0.9238795325112867385, 1.000000000000000000, 0.9238795325112867385, 1.000000000000000000, 0.9238795325112867385, 1.000000000000000000, 0.9238795325112867385, 1.000000000000000000, 0.9238795325112867385, 1.000000000000000000, 0.9238795325112867385, 1.000000000000000000, 0.9238795325112867385, 1.000000000000000000, 0.9238795325112867385, 1.000000000000000000, 0.9238795325112867385, 1.000000000000000000, 0.9238795325112867385, 1.000000000000000000, 0.9238795325112867385, 1.000000000000000000, 0.9238795325112867385, 1.000000000000000000, 0.9238795325112867385, 1.000000000000000000, 0.9238795325112867385, 1.000000000000000000, 0.9238795325112867385, 1.000000000000000000, 0.9238795325112867385, 1.000000000000000000, 0.9238795325112867385, 1.000000000000000000, 0.9238795325112867385, 1.000000000000000000, 0.9238795325112867385, 1.000000000000000000, 0.9238795325112867385, 1.000000000000000000, 0.9238795325112867385, 1.000000000000000000, 0.9238795325112867385, 1.000000000000000000, 0.9238795325112867385, 1.000000000000000000, 0.9238795325112867385, 1.000000000000000000, 0.9238795325112867385, 1.000000000000000000, 0.9238795325112867385, 1.000000000000000000, 0.9238795325112867385, 1.000000000000000000, 0.9238795325112867385, 1.000000000000000000, 0.9238795325112867385, 1.000000000000000000, 0.9238795325112867385, 1.000000000000000000, 0.9238795325112867385, 1.000000000000000000, 0.9238795325112867385, 1.000000000000000000, 0.9238795325112867385, 1.000000000000000000, 0.9238795325112867385, 1.000000000000000000, 0.9238795325112867385, 1.000000000000000000, 0.9238795325112867385, 1.000000000000000000, 0.9238795325112867385, 1.000000000000000000, 0.9238795325112867385, 1.000000000000000000, 0.9238795325112867385, 1.000000000000000000, 0.9238795325112867385, 1.000000000000000000, 0.9238795325112867385, 1.000000000000000000, 0.9238795325112867385, 1.000000000000000000, 0.9238795325112867385, 1.000000000000000000, 0.9238795325112867385, 1.000000000000000000, 0.9238795325112867385, 1.000000000000000000, 0.9238795325112867385, 1.000000000000000000, 0.9238795325112867385, 1.000000000000000000, 0.9238795325112867385, 1.000000000000000000, 0.9238795325112867385, 1.000000000000000000, 0.9238795325112867385, 1.000000000000000000, 0.9238795325112867385, 1.000000000000000000, 0.9238795325112867385, 1.000000000000000000, 0.9238795325112867385, 1.000000000000000000, 0.9238795325112867385, 1.000000000000000000, 0.9238795325112867385, 1.000000000000000000, 0.9238795325112867385, 1.000000000000000000, 0.9238795325112867385, 1.000000000000000000, 0.9238795325112867385, 1.000000000000000000, 0.9238795325112867385, 1.000000000000000000, 0.9238795325112867385, 1.000000000000000000, 0.9238795325112867385, 1.000000000000000000, 0.9238795325112867385, 1.000000000000000000, 0.9238795325112867385, 1.000000000000000000, 0.9238795325112867385, 1.000000000000000000, 0.9238795325112867385, 1.000000000000000000, 0.9238795325112867385, 1.000000000000000000, 0.9238795325112867385, 1.000000000000000000, 0.9238795325112867385, 1.000000000000000000, 0.9238795325112867385, 1.000000000000000000, 0.9238795325112867385, 1.000000000000000000, 0.9238795325112867385, 1.000000000000000000, 0.9238795325112867385, 1.000000000000000000, 0.9238795325112867385, 1.000000000000000000, 0.9238795325112867385, 1.000000000000000000, 0.9238795325112867385, 1.000000000000000000, 0.9238795325112867385, 1.000000000000000000, 0.9238795325112867385, 1.000000000000000000, 0.9238795325112867385, 1.000000000000000000, 0.9238795325112867385, 1.000000000000000000, 0.9238795325112867385, 1.000000000000000000, 0.9238795325112867385, 1.000000000000000000, 0.9238795325112867385, 1.000000000000000000, 0.9238795325112867385, 1.000000000000000000, 0.9238795325112867385, 1.000000000000000000, 0.9238795325112867385, 1.000000000000000000, 0.9238795325112867385, 1.000000000000000000, 0.9238795325112867385, 1.000000000000000000, 0.9238795325112867385, 1.000000000000000000, 0.9238795325112867385, 1.000000000000000000, 0.9238795325112867385, 1.000000000000000000, 0.9238795325112880708, 0.9999999999999986677 ) ) 
 REPRESENTATION_ITEM ( '' )  );
#20272=CARTESIAN_POINT ( 'NONE',  ( 153.9375000000000284, -4.242640687119298093, -4.242640687119298093 ) ) ;
#20274=FACE_OUTER_BOUND ( 'NONE', #19151, .T. ) ;
#20278=CYLINDRICAL_SURFACE ( 'NONE', #28289, 15.00000000000000000 ) ;
#20283=CARTESIAN_POINT ( 'NONE',  ( 159.3438746676124254, -11.34859173182233860, -3.955658370643484911 ) ) ;
#20293=CIRCLE ( 'NONE', #13452, 1.000000000000001554 ) ;
#20295=AXIS2_PLACEMENT_3D ( 'NONE', #13220, #29900, #10900 ) ;
#20296=VERTEX_POINT ( 'NONE', #27702 ) ;
#20298=CARTESIAN_POINT ( 'NONE',  ( 160.3988248654052313, 3.889087296526011706, 3.889087296526011706 ) ) ;
#20300=CARTESIAN_POINT ( 'NONE',  ( 142.4211002691896226, -4.999999999999989342, -2.071067811865468400 ) ) ;
#20301=EDGE_LOOP ( 'NONE', ( #23676, #2835, #20689, #1493 ) ) ;
#20306=CARTESIAN_POINT ( 'NONE',  ( 140.1363996827915059, -11.13639968279144910, -4.472640761300569423 ) ) ;
#20309=CARTESIAN_POINT ( 'NONE',  ( 138.0074251345948539, 2.278174593051927044, -5.500000000000096811 ) ) ;
#20310=CARTESIAN_POINT ( 'NONE',  ( 140.0625000000000284, -4.242640687119298093, 4.242640687119298093 ) ) ;
#20312=SURFACE_SIDE_STYLE ('',( #13278 ) ) ;
#20318=CARTESIAN_POINT ( 'NONE',  ( 134.5000410784369649, -6.964617708402288443, -8.000000000000007105 ) ) ;
#20319=CARTESIAN_POINT ( 'NONE',  ( 150.3601497308104058, -3.535533905932725318, -3.535533905932725318 ) ) ;
#20322=DIRECTION ( 'NONE',  ( -1.000000000000000000, 0.000000000000000000, -0.000000000000000000 ) ) ;
#20324=EDGE_CURVE ( 'NONE', #8182, #27945, #14038, .T. ) ;
#20330=ORIENTED_EDGE ( 'NONE', *, *, #22507, .T. ) ;
#20332=CARTESIAN_POINT ( 'NONE',  ( 145.3125000000000284, 4.242640687119298093, -4.242640687119298093 ) ) ;
#20333=CARTESIAN_POINT ( 'NONE',  ( 142.4136751345948539, 0.000000000000000000, -5.500000000000005329 ) ) ;
#20337=EDGE_LOOP ( 'NONE', ( #2, #13528, #3647, #21003 ) ) ;
#20340=VERTEX_POINT ( 'NONE', #28010 ) ;
#20342=VERTEX_POINT ( 'NONE', #18085 ) ;
#20348=( NAMED_UNIT ( * ) SI_UNIT ( $, .STERADIAN. ) SOLID_ANGLE_UNIT ( ) );
#20349=DIRECTION ( 'NONE',  ( 1.000000000000000000, 0.000000000000000000, 0.000000000000000000 ) ) ;
#20350=CARTESIAN_POINT ( 'NONE',  ( 0.8631338372297875372, -14.50000000000001243, 7.874007874011823560 ) ) ;
#20361=LINE ( 'NONE', #9297, #7111 ) ;
#20366=CARTESIAN_POINT ( 'NONE',  ( 150.2738248654052597, -3.889087296526011706, 3.889087296526011706 ) ) ;
#20368=ORIENTED_EDGE ( 'NONE', *, *, #20736, .F. ) ;
#20369=CARTESIAN_POINT ( 'NONE',  ( 158.9062500000000284, 6.000000000000005329, -2.485281374238555774 ) ) ;
#20377=ORIENTED_EDGE ( 'NONE', *, *, #23713, .F. ) ;
#20381=VERTEX_POINT ( 'NONE', #365 ) ;
#20383=EDGE_CURVE ( 'NONE', #13173, #14042, #5678, .T. ) ;
#20385=DIRECTION ( 'NONE',  ( 0.000000000000000000, 0.000000000000000000, -1.000000000000000000 ) ) ;
#20388=CARTESIAN_POINT ( 'NONE',  ( -0.07553485551683718213, -14.85597034017936124, 8.150736628208766987 ) ) ;
#20390=CARTESIAN_POINT ( 'NONE',  ( 146.1488248654052029, -3.889087296526011706, -3.889087296526011706 ) ) ;
#20397=B_SPLINE_CURVE_WITH_KNOTS ( 'NONE', 3,
 ( #23602, #4837, #26725, #9614 ),
 .UNSPECIFIED., .F., .F.,
 ( 4, 4 ),
 ( 0.000000000000000000, 0.0004007166227139687315 ),
 .UNSPECIFIED. ) ;
#20399=EDGE_LOOP ( 'NONE', ( #17864, #24367, #17102, #5844 ) ) ;
#20408=CARTESIAN_POINT ( 'NONE',  ( 156.9375000000000284, -4.242640687119298093, -4.242640687119298093 ) ) ;
#20411=EDGE_CURVE ( 'NONE', #13602, #15294, #20803, .T. ) ;
#20413=ORIENTED_EDGE ( 'NONE', *, *, #19855, .F. ) ;
#20414=CARTESIAN_POINT ( 'NONE',  ( 161.0000000000000284, 0.000000000000000000, -11.00000000000000355 ) ) ;
#20418=CYLINDRICAL_SURFACE ( 'NONE', #3771, 5.500000000000000000 ) ;
#20422=CARTESIAN_POINT ( 'NONE',  ( 124.9999999999999432, -71.00000000000001421, -5.000000000000004441 ) ) ;
#20425=CARTESIAN_POINT ( 'NONE',  ( 159.9008402799206863, -11.15565105496981779, -4.421997596351708637 ) ) ;
#20428=VECTOR ( 'NONE', #21621, 1000.000000000000000 ) ;
#20432=DIRECTION ( 'NONE',  ( -1.000000000000000000, 0.000000000000000000, 0.000000000000000000 ) ) ;
#20435=DIRECTION ( 'NONE',  ( 1.000000000000000000, -0.000000000000000000, -0.000000000000000000 ) ) ;
#20436=AXIS2_PLACEMENT_3D ( 'NONE', #28900, #8018, #3246 ) ;
#20437=VERTEX_POINT ( 'NONE', #2821 ) ;
#20438=CARTESIAN_POINT ( 'NONE',  ( 143.8199251345948255, -2.278174593052027408, -5.499999999999996447 ) ) ;
#20440=CARTESIAN_POINT ( 'NONE',  ( 141.5773502691896510, 5.000000000000004441, 0.000000000000000000 ) ) ;
#20445=DIRECTION ( 'NONE',  ( 1.000000000000000000, -1.387778780781444413E-14, 0.000000000000000000 ) ) ;
#20449=EDGE_LOOP ( 'NONE', ( #15601, #8252, #8429, #26103 ) ) ;
#20450=ORIENTED_EDGE ( 'NONE', *, *, #3456, .F. ) ;
#20452=CARTESIAN_POINT ( 'NONE',  ( 140.5312500000000284, -2.485281374238555774, -6.000000000000005329 ) ) ;
#20453=EDGE_CURVE ( 'NONE', #14299, #1664, #18436, .T. ) ;
#20455=AXIS2_PLACEMENT_3D ( 'NONE', #14234, #12365, #17119 ) ;
#20458=CARTESIAN_POINT ( 'NONE',  ( -0.5000000000000004441, -24.99999999999999289, 8.500000000000007105 ) ) ;
#20459=VECTOR ( 'NONE', #5043, 1000.000000000000000 ) ;
#20460=CARTESIAN_POINT ( 'NONE',  ( 130.0000000000000284, -60.00000000000001421, 3.000000000000002665 ) ) ;
#20462=CARTESIAN_POINT ( 'NONE',  ( 135.2945438920399681, -8.600858288645461869, -8.000000000000007105 ) ) ;
#20463=CARTESIAN_POINT ( 'NONE',  ( 151.3913997308104058, -2.071067811865468400, 4.999999999999989342 ) ) ;
#20466=AXIS2_PLACEMENT_3D ( 'NONE', #1233, #5841, #8144 ) ;
#20467=DIRECTION ( 'NONE',  ( -1.000000000000000000, -0.000000000000000000, -0.000000000000000000 ) ) ;
#20470=CARTESIAN_POINT ( 'NONE',  ( 137.8199251345948539, -2.278174593052098018, -5.499999999999928058 ) ) ;
#20471=CARTESIAN_POINT ( 'NONE',  ( 135.0000000000000284, 6.000000000000005329, 0.000000000000000000 ) ) ;
#20478=CARTESIAN_POINT ( 'NONE',  ( 147.4687500000000853, -2.485281374238585972, 6.000000000000005329 ) ) ;
#20481=EDGE_CURVE ( 'NONE', #8567, #23700, #25756, .T. ) ;
#20483=STYLED_ITEM ( 'NONE', ( #5650 ), #5179 ) ;
#20484=CARTESIAN_POINT ( 'NONE',  ( 140.7187500000000284, 2.485281374238555774, -6.000000000000005329 ) ) ;
#20486=ORIENTED_EDGE ( 'NONE', *, *, #20813, .T. ) ;
#20489=ORIENTED_EDGE ( 'NONE', *, *, #28029, .F. ) ;
#20498=DIRECTION ( 'NONE',  ( 0.000000000000000000, 0.000000000000000000, -1.000000000000000000 ) ) ;
#20500=DIRECTION ( 'NONE',  ( -1.000000000000000000, -1.067522139062651904E-16, 0.000000000000000000 ) ) ;
#20501=STYLED_ITEM ( 'NONE', ( #26451 ), #23889 ) ;
#20505=CARTESIAN_POINT ( 'NONE',  ( 139.8316809845309763, -9.383857069608923851, -7.879428590029234236 ) ) ;
#20510=CARTESIAN_POINT ( 'NONE',  ( 150.2961002691897079, 2.071067811865468400, -4.999999999999989342 ) ) ;
#20511=CARTESIAN_POINT ( 'NONE',  ( 150.1949251345948539, 5.500000000000012434, -2.278174593052012309 ) ) ;
#20513=AXIS2_PLACEMENT_3D ( 'NONE', #30330, #7291, #11788 ) ;
#20514=CARTESIAN_POINT ( 'NONE',  ( 161.4676415472669930, -3.677632379980754873, -4.807648994257829322 ) ) ;
#20518=CARTESIAN_POINT ( 'NONE',  ( 139.4136751345948539, 0.000000000000000000, -5.500000000000005329 ) ) ;
#20520=DIRECTION ( 'NONE',  ( 0.000000000000000000, -1.000000000000000000, 0.000000000000000000 ) ) ;
#20523=ORIENTED_EDGE ( 'NONE', *, *, #13379, .F. ) ;
#20524=CARTESIAN_POINT ( 'NONE',  ( 154.5937500000000284, 6.000000000000005329, 2.485281374238585972 ) ) ;
#20527=ORIENTED_EDGE ( 'NONE', *, *, #3467, .T. ) ;
#20530=ADVANCED_FACE ( 'NONE', ( #8297 ), #15415, .T. ) ;
#20532=ORIENTED_EDGE ( 'NONE', *, *, #21919, .T. ) ;
#20536=EDGE_LOOP ( 'NONE', ( #18957, #25778, #18393, #14162 ) ) ;
#20538=LINE ( 'NONE', #4237, #17002 ) ;
#20550=CARTESIAN_POINT ( 'NONE',  ( 159.3898502691896510, 3.535533905932725318, -3.535533905932725318 ) ) ;
#20552=CARTESIAN_POINT ( 'NONE',  ( 0.2148296108471211552, -15.54268077391681047, 8.042193295382688234 ) ) ;
#20553=EDGE_LOOP ( 'NONE', ( #28651, #6407, #5459, #15371 ) ) ;
#20559=ORIENTED_EDGE ( 'NONE', *, *, #28784, .F. ) ;
#20560=DIRECTION ( 'NONE',  ( 1.000000000000000000, -0.000000000000000000, -0.000000000000000000 ) ) ;
#20566=EDGE_CURVE ( 'NONE', #12588, #25384, #25140, .T. ) ;
#20567=EDGE_LOOP ( 'NONE', ( #24673, #13675, #20162 ) ) ;
#20568=VERTEX_POINT ( 'NONE', #24697 ) ;
#20569=CARTESIAN_POINT ( 'NONE',  ( 155.4375000000000284, -4.242640687119298093, -4.242640687119298093 ) ) ;
#20570=ORIENTED_EDGE ( 'NONE', *, *, #17249, .T. ) ;
#20578=CARTESIAN_POINT ( 'NONE',  ( 160.6082150250991276, -11.35260501843221448, 3.892452095878841778 ) ) ;
#20579=PRESENTATION_STYLE_ASSIGNMENT (( #4433 ) ) ;
#20582=CYLINDRICAL_SURFACE ( 'NONE', #489, 5.500000000000000000 ) ;
#20583=CARTESIAN_POINT ( 'NONE',  ( 159.0000000000000284, -11.33333333333333215, -4.000000000000004441 ) ) ;
#20584=CARTESIAN_POINT ( 'NONE',  ( 159.0000000000000284, -12.00000000000001066, -5.000000000000004441 ) ) ;
#20585=DIRECTION ( 'NONE',  ( -0.000000000000000000, -0.000000000000000000, 1.000000000000000000 ) ) ;
#20590=CARTESIAN_POINT ( 'NONE',  ( -9.999999999999772626, -90.00000000000001421, 3.000000000000002665 ) ) ;
#20599=DIRECTION ( 'NONE',  ( 0.000000000000000000, -1.000000000000000000, 0.000000000000000000 ) ) ;
#20600=CARTESIAN_POINT ( 'NONE',  ( -0.5000000000000004441, 0.000000000000000000, -8.500000000000007105 ) ) ;
#20601=CARTESIAN_POINT ( 'NONE',  ( 140.0773502691896510, 5.000000000000004441, 0.000000000000000000 ) ) ;
#20602=VECTOR ( 'NONE', #23443, 1000.000000000000000 ) ;
#20607=MECHANICAL_DESIGN_GEOMETRIC_PRESENTATION_REPRESENTATION('',(#18668),#28424);
#20612=ORIENTED_EDGE ( 'NONE', *, *, #10810, .F. ) ;
#20614=CARTESIAN_POINT ( 'NONE',  ( 141.8437500000000284, -6.000000000000005329, -2.485281374238555774 ) ) ;
#20618=CARTESIAN_POINT ( 'NONE',  ( -0.5000000000000004441, -15.50000000000001421, 0.000000000000000000 ) ) ;
#20619=LINE ( 'NONE', #18483, #1005 ) ;
#20620=STYLED_ITEM ( 'NONE', ( #7522 ), #27262 ) ;
#20625=CARTESIAN_POINT ( 'NONE',  ( 134.5875105163358683, -7.951309655782822006, -8.000000000000007105 ) ) ;
#20627=CARTESIAN_POINT ( 'NONE',  ( 142.2976497308104058, 0.000000000000000000, 5.000000000000004441 ) ) ;
#20629=CARTESIAN_POINT ( 'NONE',  ( 161.0000000000000284, -5.424442335930618420, -0.9085292203135086897 ) ) ;
#20631=DIRECTION ( 'NONE',  ( 0.000000000000000000, 0.000000000000000000, -1.000000000000000000 ) ) ;
#20634=DIRECTION ( 'NONE',  ( -0.000000000000000000, -1.000000000000000000, 0.000000000000000000 ) ) ;
#20643=ADVANCED_FACE ( 'NONE', ( #6567 ), #16143, .T. ) ;
#20647=CARTESIAN_POINT ( 'NONE',  ( 139.5000000000000284, 6.000000000000005329, 0.000000000000000000 ) ) ;
#20648=CYLINDRICAL_SURFACE ( 'NONE', #29763, 5.500000000000000000 ) ;
#20649=CARTESIAN_POINT ( 'NONE',  ( 136.4062500000000568, 6.000000000000005329, -2.485281374238555774 ) ) ;
#20656=DIRECTION ( 'NONE',  ( -0.000000000000000000, -0.000000000000000000, -1.000000000000000000 ) ) ;
#20658=VERTEX_POINT ( 'NONE', #14293 ) ;
#20661=CARTESIAN_POINT ( 'NONE',  ( 140.1656963055991412, -11.58284815279925262, -4.440052304730661703 ) ) ;
#20663=MECHANICAL_DESIGN_GEOMETRIC_PRESENTATION_REPRESENTATION('',(#17238),#24563);
#20665=LINE ( 'NONE', #2076, #24124 ) ;
#20667=CARTESIAN_POINT ( 'NONE',  ( 156.8363248654052313, 0.000000000000000000, -5.500000000000005329 ) ) ;
#20670=EDGE_CURVE ( 'NONE', #23700, #28026, #3169, .T. ) ;
#20672=CARTESIAN_POINT ( 'NONE',  ( 147.8586002691896510, 2.071067811865468400, 4.999999999999989342 ) ) ;
#20673=CARTESIAN_POINT ( 'NONE',  ( 0.8631338372297875372, -15.37878787878788067, 8.351220472436777342 ) ) ;
#20682=CARTESIAN_POINT ( 'NONE',  ( 153.2812500000000568, 2.485281374238585972, 6.000000000000005329 ) ) ;
#20686=CARTESIAN_POINT ( 'NONE',  ( 135.0000000000000284, -8.798545334315205579, -8.160000000000000142 ) ) ;
#20688=ORIENTED_EDGE ( 'NONE', *, *, #21805, .T. ) ;
#20689=ORIENTED_EDGE ( 'NONE', *, *, #20815, .F. ) ;
#20693=SURFACE_STYLE_USAGE ( .BOTH. , #1783 ) ;
#20694=CARTESIAN_POINT ( 'NONE',  ( -10.00000000000000178, -19.99999999999998934, 3.000000000000002665 ) ) ;
#20695=ADVANCED_FACE ( 'NONE', ( #4716 ), #18581, .F. ) ;
#20700=CARTESIAN_POINT ( 'NONE',  ( 0.000000000000000000, 0.000000000000000000, 0.000000000000000000 ) ) ;
#20703=MECHANICAL_DESIGN_GEOMETRIC_PRESENTATION_REPRESENTATION('',(#14358),#9916);
#20708=DIRECTION ( 'NONE',  ( 0.000000000000000000, 1.000000000000000000, -0.000000000000000000 ) ) ;
#20712=FILL_AREA_STYLE_COLOUR ( '', #10077 ) ;
#20713=CARTESIAN_POINT ( 'NONE',  ( -0.08172161153639843911, -15.06323960844747312, 7.964335018497379792 ) ) ;
#20714=ORIENTED_EDGE ( 'NONE', *, *, #23713, .T. ) ;
#20721=VECTOR ( 'NONE', #18449, 1000.000000000000000 ) ;
#20723=ORIENTED_EDGE ( 'NONE', *, *, #17249, .F. ) ;
#20726=CARTESIAN_POINT ( 'NONE',  ( 148.5937500000000284, 6.000000000000005329, 2.485281374238585972 ) ) ;
#20731=DIRECTION ( 'NONE',  ( -0.000000000000000000, -0.000000000000000000, -1.000000000000000000 ) ) ;
#20734=DIRECTION ( 'NONE',  ( 0.000000000000000000, 0.000000000000000000, -1.000000000000000000 ) ) ;
#20736=EDGE_CURVE ( 'NONE', #7007, #6912, #10664, .T. ) ;
#20739=CARTESIAN_POINT ( 'NONE',  ( 0.2015195925780142172, -15.64213524437055192, -7.848188837846724830 ) ) ;
#20742=FACE_OUTER_BOUND ( 'NONE', #27740, .T. ) ;
#20743=CARTESIAN_POINT ( 'NONE',  ( 158.0550748654052313, -5.500000000000012434, -2.278174593052012309 ) ) ;
#20748=CARTESIAN_POINT ( 'NONE',  ( -0.2114713642193687404, -9.788528635780680887, -4.341247053692759650 ) ) ;
#20755=( NAMED_UNIT ( * ) SI_UNIT ( $, .STERADIAN. ) SOLID_ANGLE_UNIT ( ) );
#20756=CARTESIAN_POINT ( 'NONE',  ( 154.4925748654052882, 2.278174593051942587, 5.500000000000080824 ) ) ;
#20761=AXIS2_PLACEMENT_3D ( 'NONE', #14290, #23631, #11989 ) ;
#20769=VERTEX_POINT ( 'NONE', #25619 ) ;
#20770=EDGE_LOOP ( 'NONE', ( #1160, #25853, #29589, #19476 ) ) ;
#20771=CARTESIAN_POINT ( 'NONE',  ( 159.0000000000000284, -12.00000000000001066, 4.000000000000003553 ) ) ;
#20772=CARTESIAN_POINT ( 'NONE',  ( 136.8750000000000284, 0.000000000000000000, 6.000000000000005329 ) ) ;
#20777=EDGE_CURVE ( 'NONE', #25006, #27165, #16420, .T. ) ;
#20779=FACE_OUTER_BOUND ( 'NONE', #2638, .T. ) ;
#20782=AXIS2_PLACEMENT_3D ( 'NONE', #3762, #21917, #17626 ) ;
#20783=CARTESIAN_POINT ( 'NONE',  ( 141.4538997308104058, -2.071067811865468400, -4.999999999999989342 ) ) ;
#20785=DIRECTION ( 'NONE',  ( 1.000000000000000000, -0.000000000000000000, -0.000000000000000000 ) ) ;
#20792=CARTESIAN_POINT ( 'NONE',  ( 137.1636751345948255, 0.000000000000000000, 5.500000000000005329 ) ) ;
#20794=CARTESIAN_POINT ( 'NONE',  ( 116.0000000000000142, 0.000000000000000000, 0.000000000000000000 ) ) ;
#20802=CARTESIAN_POINT ( 'NONE',  ( 138.7500000000000284, -6.000000000000005329, 0.000000000000000000 ) ) ;
#20803=B_SPLINE_CURVE_WITH_KNOTS ( 'NONE', 3,
 ( #23876, #11952, #17554, #7996, #21278, #17401 ),
 .UNSPECIFIED., .F., .F.,
 ( 4, 2, 4 ),
 ( 0.000000000000000000, 0.001072522389057926949, 0.002145044778115853899 ),
 .UNSPECIFIED. ) ;
#20806=CARTESIAN_POINT ( 'NONE',  ( 138.7500000000000284, -6.000000000000005329, 0.000000000000000000 ) ) ;
#20809=VERTEX_POINT ( 'NONE', #15009 ) ;
#20811=VERTEX_POINT ( 'NONE', #19324 ) ;
#20813=EDGE_CURVE ( 'NONE', #25966, #25175, #27207, .T. ) ;
#20815=EDGE_CURVE ( 'NONE', #12881, #5798, #29671, .T. ) ;
#20816=PRODUCT_DEFINITION ( 'UNKNOWN', '', #6531, #25523 ) ;
#20817=CARTESIAN_POINT ( 'NONE',  ( -4.999999999999990230, -24.99999999999999289, -7.500000000000007105 ) ) ;
#20821=CARTESIAN_POINT ( 'NONE',  ( 140.4999999682997895, -9.426604554197883346, -7.431193927736174487 ) ) ;
#20831=CARTESIAN_POINT ( 'NONE',  ( 156.8437500000000284, -6.000000000000005329, -2.485281374238556218 ) ) ;
#20838=CARTESIAN_POINT ( 'NONE',  ( 156.3750000000000284, 0.000000000000000000, 6.000000000000005329 ) ) ;
#20843=EDGE_LOOP ( 'NONE', ( #18116, #23711, #30038, #14361 ) ) ;
#20853=FILL_AREA_STYLE ('',( #13212 ) ) ;
#20858=AXIS2_PLACEMENT_3D ( 'NONE', #21760, #703, #17162 ) ;
#20864=CARTESIAN_POINT ( 'NONE',  ( 158.5461002691896510, -2.071067811865468400, 4.999999999999989342 ) ) ;
#20865=CARTESIAN_POINT ( 'NONE',  ( 0.2014817752041039023, -15.64225424449952229, 7.847953382956076140 ) ) ;
#20872=VECTOR ( 'NONE', #26289, 1000.000000000000000 ) ;
#20875=CARTESIAN_POINT ( 'NONE',  ( 124.9999999999999432, -65.00000000000000000, 8.000000000000007105 ) ) ;
#20876=CARTESIAN_POINT ( 'NONE',  ( 152.1562500000000284, -6.000000000000005329, 2.485281374238555774 ) ) ;
#20881=( BOUNDED_CURVE ( )  B_SPLINE_CURVE ( 3, ( #9000, #22675, #30182, #6832 ),
 .UNSPECIFIED., .F., .F. ) 
 B_SPLINE_CURVE_WITH_KNOTS ( ( 4, 4 ),
 ( 1.570796326794896558, 2.746801533890022906 ),
 .UNSPECIFIED. ) 
 CURVE ( )  GEOMETRIC_REPRESENTATION_ITEM ( )  RATIONAL_B_SPLINE_CURVE ( ( 1.000000000000000000, 0.8880335295585641830, 0.8880335295585641830, 1.000000000000000000 ) ) 
 REPRESENTATION_ITEM ( '' )  );
#20885=( NAMED_UNIT ( * ) SI_UNIT ( $, .STERADIAN. ) SOLID_ANGLE_UNIT ( ) );
#20890=CARTESIAN_POINT ( 'NONE',  ( 0.7528903888467955996, -15.55266350887514903, -8.022782003273663420 ) ) ;
#20892=( BOUNDED_SURFACE ( )  B_SPLINE_SURFACE ( 3, 2, ( 
 ( #26727, #5690, #24588 ),
 ( #29345, #21852, #29185 ),
 ( #3537, #15102, #19993 ),
 ( #22154, #797, #24285 ),
 ( #5241, #5392, #932 ),
 ( #17412, #3232, #12968 ),
 ( #12512, #17564, #10490 ),
 ( #12658, #8146, #16963 ) ),
 .UNSPECIFIED., .F., .F., .T. ) 
 B_SPLINE_SURFACE_WITH_KNOTS ( ( 4, 2, 2, 4 ),
 ( 3, 3 ),
 ( 1.570796326794896558, 2.158798930342461730, 2.452800232116244317, 2.746801533890027347 ),
 ( 0.000000000000000000, 1.000000000000000000 ),
 .UNSPECIFIED. ) 
 GEOMETRIC_REPRESENTATION_ITEM ( )  RATIONAL_B_SPLINE_SURFACE ( (
 ( 1.000000000000000000, 1.000000000000000000, 1.000000000000000000),
 ( 1.000000000000000000, 1.000817594376257835, 1.000000000000000000),
 ( 1.000000000000000000, 0.9690373989631937413, 1.000000000000000000),
 ( 1.000000000000000000, 0.8952806170301043087, 1.000000000000000000),
 ( 1.000000000000000000, 0.8665500556586805958, 1.000000000000000000),
 ( 1.000000000000000000, 0.8091552864627657993, 1.000000000000000000),
 ( 1.000000000000000000, 0.7805842023125286744, 1.000000000000000000),
 ( 1.000000000000000000, 0.7576044462920088485, 1.000000000000000000) ) ) 
 REPRESENTATION_ITEM ( '' )  SURFACE ( )  );
#20894=CARTESIAN_POINT ( 'NONE',  ( 153.2886751345948255, 5.500000000000005329, 0.000000000000000000 ) ) ;
#20896=CARTESIAN_POINT ( 'NONE',  ( -4.999999999999990230, -55.00000000000002132, -7.500000000000007105 ) ) ;
#20897=CARTESIAN_POINT ( 'NONE',  ( 157.5863248654052597, 0.000000000000000000, 5.500000000000005329 ) ) ;
#20903=CARTESIAN_POINT ( 'NONE',  ( -1.000000000000001776, -9.000000000000007105, -4.000000000000005329 ) ) ;
#20907=CARTESIAN_POINT ( 'NONE',  ( 135.0000000000000284, -8.793943684514120562, -7.941504649977358277 ) ) ;
#20910=CARTESIAN_POINT ( 'NONE',  ( 143.7261751345948539, -3.889087296526011706, -3.889087296526011706 ) ) ;
#20921=DIRECTION ( 'NONE',  ( 0.000000000000000000, -1.000000000000000000, 0.000000000000000000 ) ) ;
#20922=CARTESIAN_POINT ( 'NONE',  ( 136.2187500000000284, 2.485281374238555774, -6.000000000000005329 ) ) ;
#20929=PRESENTATION_STYLE_ASSIGNMENT (( #4010 ) ) ;
#20931=CARTESIAN_POINT ( 'NONE',  ( 135.7516005668298078, -9.165151352129356610, -8.000000000000007105 ) ) ;
#20932=CARTESIAN_POINT ( 'NONE',  ( 144.6413997308104342, 2.071067811865468400, -4.999999999999989342 ) ) ;
#20936=FACE_OUTER_BOUND ( 'NONE', #6538, .T. ) ;
#20937=DIRECTION ( 'NONE',  ( 1.000000000000000000, -0.000000000000000000, 0.000000000000000000 ) ) ;
#20943=VECTOR ( 'NONE', #5517, 1000.000000000000000 ) ;
#20950=CARTESIAN_POINT ( 'NONE',  ( 137.5312500000000284, -2.485281374238556218, -6.000000000000005329 ) ) ;
#20953=CARTESIAN_POINT ( 'NONE',  ( 143.0699251345947971, 2.278174593052322283, 5.499999999999701572 ) ) ;
#20954=CARTESIAN_POINT ( 'NONE',  ( 160.2976497308104342, 0.000000000000000000, 5.000000000000004441 ) ) ;
#20956=CIRCLE ( 'NONE', #12659, 0.5000000000000004441 ) ;
#20959=ORIENTED_EDGE ( 'NONE', *, *, #25688, .F. ) ;
#20962=ORIENTED_EDGE ( 'NONE', *, *, #4037, .F. ) ;
#20965=DIRECTION ( 'NONE',  ( 0.3742395684071963546, 0.4425345409093133231, -0.8149281720130793216 ) ) ;
#20967=CIRCLE ( 'NONE', #13144, 15.00000000000000000 ) ;
#20968=CARTESIAN_POINT ( 'NONE',  ( 152.3511751345948539, -3.889087296526011706, 3.889087296526011706 ) ) ;
#20971=DIRECTION ( 'NONE',  ( 1.000000000000000000, 0.000000000000000000, 0.000000000000000000 ) ) ;
#20974=CARTESIAN_POINT ( 'NONE',  ( 139.5000000000000000, -8.946933499675704837, 8.000000000000007105 ) ) ;
#20985=CARTESIAN_POINT ( 'NONE',  ( 149.6398502691896510, -3.535533905932752852, 3.535533905932725318 ) ) ;
#20988=CARTESIAN_POINT ( 'NONE',  ( 158.6250000000000568, 0.000000000000000000, -6.000000000000005329 ) ) ;
#20990=CARTESIAN_POINT ( 'NONE',  ( 138.8511751345948255, -3.889087296526011706, 3.889087296526011706 ) ) ;
#20994=PRESENTATION_STYLE_ASSIGNMENT (( #11648 ) ) ;
#20996=EDGE_LOOP ( 'NONE', ( #1279, #11261, #14720, #26356 ) ) ;
#20997=CARTESIAN_POINT ( 'NONE',  ( 150.8437500000000284, -6.000000000000005329, -2.485281374238555774 ) ) ;
#20998=VECTOR ( 'NONE', #16325, 1000.000000000000114 ) ;
#21001=ORIENTED_EDGE ( 'NONE', *, *, #26950, .T. ) ;
#21003=ORIENTED_EDGE ( 'NONE', *, *, #15240, .T. ) ;
#21006=EDGE_LOOP ( 'NONE', ( #187, #22720, #27444, #10916 ) ) ;
#21007=CYLINDRICAL_SURFACE ( 'NONE', #15239, 5.500000000000000000 ) ;
#21008=CARTESIAN_POINT ( 'NONE',  ( 156.0788997308104058, -4.999999999999989342, 2.071067811865468400 ) ) ;
#21018=CARTESIAN_POINT ( 'NONE',  ( 160.7023502691896510, 0.000000000000000000, -5.000000000000004441 ) ) ;
#21019=CARTESIAN_POINT ( 'NONE',  ( 134.9999999999997158, -6.982120021893415185, 8.500000000000007105 ) ) ;
#21020=AXIS2_PLACEMENT_3D ( 'NONE', #19697, #28475, #7146 ) ;
#21021=ORIENTED_EDGE ( 'NONE', *, *, #19430, .T. ) ;
#21027=CARTESIAN_POINT ( 'NONE',  ( 161.0957217774242736, 0.3141511273712443986, 5.595721777424251364 ) ) ;
#21037=ORIENTED_EDGE ( 'NONE', *, *, #23791, .T. ) ;
#21038=CARTESIAN_POINT ( 'NONE',  ( 149.1562500000000284, -6.000000000000005329, 2.485281374238555774 ) ) ;
#21042=ORIENTED_EDGE ( 'NONE', *, *, #88, .F. ) ;
#21043=CARTESIAN_POINT ( 'NONE',  ( 158.6175748654052313, 5.500000000000012434, -2.278174593052012309 ) ) ;
#21052=CARTESIAN_POINT ( 'NONE',  ( -39.00000000000000000, -20.00000000000021316, -4.000000000000003553 ) ) ;
#21054=CARTESIAN_POINT ( 'NONE',  ( -4.999999999999990230, -24.99999999999999289, -8.000000000000007105 ) ) ;
#21056=CARTESIAN_POINT ( 'NONE',  ( 135.0000000000000000, -7.896660352823049678, -8.122336518022390095 ) ) ;
#21065=CARTESIAN_POINT ( 'NONE',  ( 151.0238248654052313, 3.889087296526011706, -3.889087296526011706 ) ) ;
#21067=SURFACE_STYLE_USAGE ( .BOTH. , #11724 ) ;
#21070=( BOUNDED_CURVE ( )  B_SPLINE_CURVE ( 2, ( #30204, #30355, #30047, #4845, #9322, #7159, #14272, #16572, #8870 ),
 .UNSPECIFIED., .F., .F. ) 
 B_SPLINE_CURVE_WITH_KNOTS ( ( 3, 2, 2, 2, 3 ),
 ( 0.06250000000000052736, 0.06875000000000031086, 0.07500000000000006661, 0.08124999999999985012, 0.08749999999999961975 ),
 .UNSPECIFIED. ) 
 CURVE ( )  GEOMETRIC_REPRESENTATION_ITEM ( )  RATIONAL_B_SPLINE_CURVE ( ( 0.9999999999999935607, 0.9238795325112931778, 1.000000000000000000, 0.9238795325112867385, 1.000000000000000000, 0.9238795325112867385, 1.000000000000000000, 0.9238795325112912904, 0.9999999999999954481 ) ) 
 REPRESENTATION_ITEM ( '' )  );
#21074=CARTESIAN_POINT ( 'NONE',  ( 138.7500000000000284, -6.000000000000005329, 0.000000000000000000 ) ) ;
#21077=DIRECTION ( 'NONE',  ( 1.000000000000000000, 0.000000000000000000, 0.000000000000000000 ) ) ;
#21083=CARTESIAN_POINT ( 'NONE',  ( 142.0163997308104626, 4.999999999999989342, 2.071067811865468400 ) ) ;
#21085=LINE ( 'NONE', #23691, #3451 ) ;
#21086=ADVANCED_FACE ( 'NONE', ( #1462 ), #8380, .T. ) ;
#21093=AXIS2_PLACEMENT_3D ( 'NONE', #2218, #15818, #27268 ) ;
#21096=CARTESIAN_POINT ( 'NONE',  ( -4.999999999999913847, -65.50000000000001421, 7.500000000000007105 ) ) ;
#21104=CARTESIAN_POINT ( 'NONE',  ( 137.1562500000000284, -6.000000000000005329, 2.485281374238556218 ) ) ;
#21106=LINE ( 'NONE', #21404, #21457 ) ;
#21107=CARTESIAN_POINT ( 'NONE',  ( 134.8125000000000284, 4.242640687119298093, -4.242640687119298093 ) ) ;
#21109=AXIS2_PLACEMENT_3D ( 'NONE', #27124, #29596, #29740 ) ;
#21111=ORIENTED_EDGE ( 'NONE', *, *, #4997, .F. ) ;
#21119=( BOUNDED_CURVE ( )  B_SPLINE_CURVE ( 2, ( #24273, #10476, #19543, #10020, #24426, #19398, #19830, #7840, #10635 ),
 .UNSPECIFIED., .F., .T. ) 
 B_SPLINE_CURVE_WITH_KNOTS ( ( 3, 2, 2, 2, 3 ),
 ( 0.2625000000000007327, 0.2687500000000004885, 0.2750000000000002998, 0.2812500000000000555, 0.2874999999999998113 ),
 .UNSPECIFIED. ) 
 CURVE ( )  GEOMETRIC_REPRESENTATION_ITEM ( )  RATIONAL_B_SPLINE_CURVE ( ( 0.9999999999999912292, 0.9238795325112955092, 1.000000000000000000, 0.9238795325112867385, 1.000000000000000000, 0.9238795325112867385, 1.000000000000000000, 0.9238795325112887369, 0.9999999999999980016 ) ) 
 REPRESENTATION_ITEM ( '' )  );
#21122=CARTESIAN_POINT ( 'NONE',  ( 139.6069567752852265, -8.946933505375708862, -7.999999993627826989 ) ) ;
#21125=DIRECTION ( 'NONE',  ( 1.000000000000000000, -6.938893903907221278E-15, 0.000000000000000000 ) ) ;
#21126=CIRCLE ( 'NONE', #20139, 5.500000000000000000 ) ;
#21132=CARTESIAN_POINT ( 'NONE',  ( 144.1086002691896226, -2.071067811865468400, -4.999999999999989342 ) ) ;
#21135=CARTESIAN_POINT ( 'NONE',  ( 157.7812500000000284, 2.485281374238585972, 6.000000000000005329 ) ) ;
#21138=DIRECTION ( 'NONE',  ( 0.000000000000000000, 1.000000000000000000, 0.000000000000000000 ) ) ;
#21142=CARTESIAN_POINT ( 'NONE',  ( 150.4687500000000284, -2.485281374238585972, 6.000000000000005329 ) ) ;
#21146=EDGE_LOOP ( 'NONE', ( #28070, #25985, #412, #23857 ) ) ;
#21151=ORIENTED_EDGE ( 'NONE', *, *, #11446, .T. ) ;
#21154=CARTESIAN_POINT ( 'NONE',  ( 154.4851497308104058, -3.535533905932725318, 3.535533905932725318 ) ) ;
#21159=( BOUNDED_CURVE ( )  B_SPLINE_CURVE ( 2, ( #17625, #26947, #13030, #22368, #10718, #7297, #11795, #11329, #30180 ),
 .UNSPECIFIED., .F., .T. ) 
 B_SPLINE_CURVE_WITH_KNOTS ( ( 3, 2, 2, 2, 3 ),
 ( 0.5625000000000009992, 0.5687500000000007550, 0.5750000000000005107, 0.5812500000000003775, 0.5875000000000001332 ),
 .UNSPECIFIED. ) 
 CURVE ( )  GEOMETRIC_REPRESENTATION_ITEM ( )  RATIONAL_B_SPLINE_CURVE ( ( 0.9999999999999877875, 0.9238795325112989509, 1.000000000000000000, 0.9238795325112867385, 1.000000000000000000, 0.9238795325112867385, 1.000000000000000000, 0.9238795325112854062, 1.000000000000001332 ) ) 
 REPRESENTATION_ITEM ( '' )  );
#21160=VECTOR ( 'NONE', #4172, 1000.000000000000000 ) ;
#21169=CARTESIAN_POINT ( 'NONE',  ( 162.0148502691896510, -3.535533905932725318, -3.535533905932725318 ) ) ;
#21170=CARTESIAN_POINT ( 'NONE',  ( -0.07584961804942320918, -14.87383459521561591, 8.134942876244384280 ) ) ;
#21175=CIRCLE ( 'NONE', #14340, 0.9999999999999995559 ) ;
#21181=( GEOMETRIC_REPRESENTATION_CONTEXT ( 3 ) GLOBAL_UNCERTAINTY_ASSIGNED_CONTEXT ( ( #23785 ) ) GLOBAL_UNIT_ASSIGNED_CONTEXT ( ( #23670, #2607, #26396 ) ) REPRESENTATION_CONTEXT ( 'NONE', 'WORKASPACE' ) );
#21184=ORIENTED_EDGE ( 'NONE', *, *, #4064, .T. ) ;
#21185=CARTESIAN_POINT ( 'NONE',  ( 150.9375000000000284, -4.242640687119298093, -4.242640687119298093 ) ) ;
#21194=( LENGTH_UNIT ( ) NAMED_UNIT ( * ) SI_UNIT ( .MILLI., .METRE. ) );
#21195=TOROIDAL_SURFACE ( 'NONE', #6945, 10.49999999999999645, 0.5000000000000000000 ) ;
#21198=CARTESIAN_POINT ( 'NONE',  ( -0.07587193451662191390, -14.87436656268081414, -8.134582247911094299 ) ) ;
#21199=ADVANCED_FACE ( 'NONE', ( #30185 ), #23348, .T. ) ;
#21205=CARTESIAN_POINT ( 'NONE',  ( -0.9018315097318220230, -9.098168490268067288, -4.000092554054210048 ) ) ;
#21207=CARTESIAN_POINT ( 'NONE',  ( 161.0000000000000568, -11.64607081028603552, -2.895853930524592279 ) ) ;
#21210=ORIENTED_EDGE ( 'NONE', *, *, #8019, .F. ) ;
#21212=CARTESIAN_POINT ( 'NONE',  ( -0.004414515218767962011, -15.41919126527335315, 6.290392408496218835 ) ) ;
#21215=ORIENTED_EDGE ( 'NONE', *, *, #8554, .F. ) ;
#21217=CARTESIAN_POINT ( 'NONE',  ( 139.5000000000000000, -8.798545334315205579, 8.160000000000000142 ) ) ;
#21218=AXIS2_PLACEMENT_3D ( 'NONE', #4980, #24179, #28768 ) ;
#21220=CARTESIAN_POINT ( 'NONE',  ( -0.5000000000000004441, -10.00000000000000888, 5.000000000000004441 ) ) ;
#21224=CARTESIAN_POINT ( 'NONE',  ( -4.999999999999990230, -24.99999999999999289, 8.000000000000007105 ) ) ;
#21225=CARTESIAN_POINT ( 'NONE',  ( 133.1250000000000284, 0.000000000000000000, -6.000000000000005329 ) ) ;
#21229=DIRECTION ( 'NONE',  ( 0.000000000000000000, 0.000000000000000000, 1.000000000000000000 ) ) ;
#21232=DIRECTION ( 'NONE',  ( 0.000000000000000000, 0.000000000000000000, -1.000000000000000000 ) ) ;
#21233=CARTESIAN_POINT ( 'NONE',  ( 145.8601497308104058, -3.535533905932725318, -3.535533905932725318 ) ) ;
#21240=FACE_OUTER_BOUND ( 'NONE', #30298, .T. ) ;
#21241=ORIENTED_EDGE ( 'NONE', *, *, #845, .T. ) ;
#21248=CARTESIAN_POINT ( 'NONE',  ( 139.8750000000000284, 0.000000000000000000, 6.000000000000005329 ) ) ;
#21251=( BOUNDED_CURVE ( )  B_SPLINE_CURVE ( 2, ( #15412, #1696, #20298, #29644, #24738, #22294, #3836, #25031, #8611 ),
 .UNSPECIFIED., .F., .T. ) 
 B_SPLINE_CURVE_WITH_KNOTS ( ( 3, 2, 2, 2, 3 ),
 ( 0.03749999999999957534, 0.04374999999999980987, 0.05000000000000005829, 0.05625000000000029282, 0.06250000000000052736 ),
 .UNSPECIFIED. ) 
 CURVE ( )  GEOMETRIC_REPRESENTATION_ITEM ( )  RATIONAL_B_SPLINE_CURVE ( ( 1.000000000000005107, 0.9238795325112816315, 1.000000000000000000, 0.9238795325112867385, 1.000000000000000000, 0.9238795325112867385, 1.000000000000000000, 0.9238795325112802992, 1.000000000000006439 ) ) 
 REPRESENTATION_ITEM ( '' )  );
#21252=CARTESIAN_POINT ( 'NONE',  ( 134.4375000000000568, -4.242640687119298093, -4.242640687119298093 ) ) ;
#21254=EDGE_CURVE ( 'NONE', #19300, #8188, #16506, .T. ) ;
#21256=CIRCLE ( 'NONE', #20782, 9.999999999999996447 ) ;
#21257=ORIENTED_EDGE ( 'NONE', *, *, #17666, .F. ) ;
#21260=DIRECTION ( 'NONE',  ( 0.000000000000000000, 0.000000000000000000, 1.000000000000000000 ) ) ;
#21263=EDGE_CURVE ( 'NONE', #28771, #26763, #8101, .T. ) ;
#21266=CARTESIAN_POINT ( 'NONE',  ( 141.0000000000000284, -12.00000000000001066, -4.000000000000003553 ) ) ;
#21271=CARTESIAN_POINT ( 'NONE',  ( -4.999999999999886313, -10.50000000000000888, 7.500000000000007105 ) ) ;
#21276=FACE_OUTER_BOUND ( 'NONE', #24862, .T. ) ;
#21277=CARTESIAN_POINT ( 'NONE',  ( 143.6398502691896510, -3.535533905932752852, 3.535533905932725318 ) ) ;
#21278=CARTESIAN_POINT ( 'NONE',  ( 1.000000000000000888, -16.31586670994438037, 6.338163299696072173 ) ) ;
#21279=VECTOR ( 'NONE', #5943, 1000.000000000000000 ) ;
#21280=CARTESIAN_POINT ( 'NONE',  ( 160.4062500000000284, 6.000000000000005329, -2.485281374238556218 ) ) ;
#21286=ORIENTED_EDGE ( 'NONE', *, *, #15779, .T. ) ;
#21287=CARTESIAN_POINT ( 'NONE',  ( 147.2812500000000284, 2.485281374238585972, 6.000000000000005329 ) ) ;
#21297=EDGE_CURVE ( 'NONE', #25911, #12140, #11614, .T. ) ;
#21300=CARTESIAN_POINT ( 'NONE',  ( 154.1101497308104058, 3.535533905932725318, 3.535533905932725318 ) ) ;
#21302=( NAMED_UNIT ( * ) PLANE_ANGLE_UNIT ( ) SI_UNIT ( $, .RADIAN. ) );
#21310=( NAMED_UNIT ( * ) PLANE_ANGLE_UNIT ( ) SI_UNIT ( $, .RADIAN. ) );
#21314=CARTESIAN_POINT ( 'NONE',  ( 157.7961002691896510, 2.071067811865468400, -4.999999999999989342 ) ) ;
#21315=LINE ( 'NONE', #258, #8657 ) ;
#21320=CARTESIAN_POINT ( 'NONE',  ( 160.0000000000000284, -12.64911064067353408, 3.000000000000002665 ) ) ;
#21325=CARTESIAN_POINT ( 'NONE',  ( 0.000000000000000000, -10.00000000000000888, 7.500000000000007105 ) ) ;
#21330=CARTESIAN_POINT ( 'NONE',  ( 125.0000000000000568, -55.00000000000000711, -7.500000000000007105 ) ) ;
#21331=CARTESIAN_POINT ( 'NONE',  ( 151.2187500000000284, 2.485281374238555774, -6.000000000000005329 ) ) ;
#21334=ADVANCED_FACE ( 'NONE', ( #2246 ), #6690, .F. ) ;
#21337=UNCERTAINTY_MEASURE_WITH_UNIT (LENGTH_MEASURE( 1.000000000000000082E-05 ), #21194, 'distance_accuracy_value', 'NONE');
#21341=CARTESIAN_POINT ( 'NONE',  ( 134.5163997308104342, 4.999999999999989342, 2.071067811865468400 ) ) ;
#21343=CARTESIAN_POINT ( 'NONE',  ( 153.5699251345948539, 2.278174593052229469, 5.499999999999796607 ) ) ;
#21344=PRESENTATION_STYLE_ASSIGNMENT (( #5477 ) ) ;
#21351=UNCERTAINTY_MEASURE_WITH_UNIT (LENGTH_MEASURE( 1.000000000000000082E-05 ), #29969, 'distance_accuracy_value', 'NONE');
#21354=CARTESIAN_POINT ( 'NONE',  ( 135.0000000000000284, -9.047800747817511535, -7.999999999998980371 ) ) ;
#21356=EDGE_LOOP ( 'NONE', ( #27649, #6095, #6612, #30061 ) ) ;
#21358=CARTESIAN_POINT ( 'NONE',  ( 8.673617379884035472E-16, -15.50000000000001421, 5.656854249492387687 ) ) ;
#21363=B_SPLINE_CURVE_WITH_KNOTS ( 'NONE', 3,
 ( #26433, #5389, #21994, #6306, #1549, #24747, #3533, #10640, #27036, #3996, #6163, #13271, #25039, #24892, #13415, #6461 ),
 .UNSPECIFIED., .F., .F.,
 ( 4, 2, 2, 2, 2, 2, 2, 4 ),
 ( 0.000000000000000000, 0.001733696408318075163, 0.002600544612477113070, 0.003467392816636151627, 0.004334241020795190184, 0.005201089224954227874, 0.006067937429113266432, 0.006934785633272304989 ),
 .UNSPECIFIED. ) ;
#21371=EDGE_LOOP ( 'NONE', ( #11757, #18590, #7109, #30293 ) ) ;
#21374=CARTESIAN_POINT ( 'NONE',  ( 136.6875000000000284, 4.242640687119269671, 4.242640687119298093 ) ) ;
#21378=FILL_AREA_STYLE ('',( #18943 ) ) ;
#21382=DIRECTION ( 'NONE',  ( 1.000000000000000000, 0.000000000000000000, -0.000000000000000000 ) ) ;
#21384=CARTESIAN_POINT ( 'NONE',  ( -0.5000000000000004441, -10.00000000000000888, 5.000000000000004441 ) ) ;
#21385=CARTESIAN_POINT ( 'NONE',  ( 139.3913997308104342, -2.071067811865468400, 4.999999999999989342 ) ) ;
#21389=STYLED_ITEM ( 'NONE', ( #20994 ), #21334 ) ;
#21400=ORIENTED_EDGE ( 'NONE', *, *, #12507, .T. ) ;
#21404=CARTESIAN_POINT ( 'NONE',  ( 159.0000000000000284, -19.99999999999998934, -4.000000000000003553 ) ) ;
#21405=ADVANCED_FACE ( 'NONE', ( #2825 ), #9759, .F. ) ;
#21406=CARTESIAN_POINT ( 'NONE',  ( 133.6875000000000284, 4.242640687119269671, 4.242640687119298093 ) ) ;
#21409=ORIENTED_EDGE ( 'NONE', *, *, #13768, .F. ) ;
#21413=CARTESIAN_POINT ( 'NONE',  ( 159.1446212341123783, -12.00000000000001243, -4.000000000000004441 ) ) ;
#21416=CARTESIAN_POINT ( 'NONE',  ( -1.000000000000000888, -9.000000000000007105, -4.000000000000003553 ) ) ;
#21423=CARTESIAN_POINT ( 'NONE',  ( 139.8520630996757177, -9.423463366246116024, 7.856467294622035524 ) ) ;
#21428=CARTESIAN_POINT ( 'NONE',  ( 145.0238248654052029, 3.889087296526011706, -3.889087296526011706 ) ) ;
#21432=CARTESIAN_POINT ( 'NONE',  ( 139.5983683982788648, -9.179625746858260271, 7.992216821685455663 ) ) ;
#21434=CARTESIAN_POINT ( 'NONE',  ( 160.6875000000000284, 4.242640687119269671, 4.242640687119298093 ) ) ;
#21435=CARTESIAN_POINT ( 'NONE',  ( 135.0000000000025864, -7.147641677108396152, -8.399623149008458967 ) ) ;
#21436=CARTESIAN_POINT ( 'NONE',  ( 136.0000000000000284, -8.798545334315205579, -8.160000000000000142 ) ) ;
#21440=CARTESIAN_POINT ( 'NONE',  ( 151.5000000000000284, 6.000000000000005329, 0.000000000000000000 ) ) ;
#21452=CARTESIAN_POINT ( 'NONE',  ( 153.3601497308104058, -3.535533905932725318, -3.535533905932725318 ) ) ;
#21454=DIRECTION ( 'NONE',  ( -1.000000000000000000, 0.000000000000000000, 0.000000000000000000 ) ) ;
#21455=LINE ( 'NONE', #2842, #11686 ) ;
#21457=VECTOR ( 'NONE', #9423, 1000.000000000000000 ) ;
#21463=CIRCLE ( 'NONE', #13636, 1.000000000000000888 ) ;
#21469=CARTESIAN_POINT ( 'NONE',  ( 141.8363248654052029, 0.000000000000000000, -5.500000000000005329 ) ) ;
#21471=DIRECTION ( 'NONE',  ( 1.000000000000000000, -0.000000000000000000, -0.000000000000000000 ) ) ;
#21472=CARTESIAN_POINT ( 'NONE',  ( 158.0773502691896510, 5.000000000000004441, 0.000000000000000000 ) ) ;
#21479=DIRECTION ( 'NONE',  ( 6.938893903907222067E-15, -1.000000000000000000, 0.000000000000000000 ) ) ;
#21481=CARTESIAN_POINT ( 'NONE',  ( 159.0000000000000284, -11.07692307692306777, -4.615384615384604317 ) ) ;
#21482=DIRECTION ( 'NONE',  ( -0.000000000000000000, 1.000000000000000000, -0.000000000000000000 ) ) ;
#21485=STYLED_ITEM ( 'NONE', ( #14859 ), #5546 ) ;
#21487=CARTESIAN_POINT ( 'NONE',  ( 145.4062500000000284, 6.000000000000005329, -2.485281374238555774 ) ) ;
#21488=ORIENTED_EDGE ( 'NONE', *, *, #9118, .T. ) ;
#21496=AXIS2_PLACEMENT_3D ( 'NONE', #6501, #6803, #6661 ) ;
#21497=CARTESIAN_POINT ( 'NONE',  ( 134.1413997308104058, 2.071067811865468400, -4.999999999999989342 ) ) ;
#21499=CARTESIAN_POINT ( 'NONE',  ( 0.2148510768240012581, -15.54319609401394331, -8.041199716608099735 ) ) ;
#21513=ORIENTED_EDGE ( 'NONE', *, *, #610, .F. ) ;
#21520=ORIENTED_EDGE ( 'NONE', *, *, #5486, .T. ) ;
#21523=EDGE_LOOP ( 'NONE', ( #14804, #652, #17150, #4428 ) ) ;
#21526=ORIENTED_EDGE ( 'NONE', *, *, #26698, .T. ) ;
#21527=EDGE_LOOP ( 'NONE', ( #19728, #8066, #6388, #27263 ) ) ;
#21528=CARTESIAN_POINT ( 'NONE',  ( 132.9375000000000284, -4.242640687119298093, -4.242640687119298093 ) ) ;
#21529=CARTESIAN_POINT ( 'NONE',  ( 135.0148502691896510, -3.535533905932725318, -3.535533905932725318 ) ) ;
#21530=ORIENTED_EDGE ( 'NONE', *, *, #5580, .F. ) ;
#21534=ORIENTED_EDGE ( 'NONE', *, *, #24317, .F. ) ;
#21538=CARTESIAN_POINT ( 'NONE',  ( 137.7976497308104058, 0.000000000000000000, 5.000000000000004441 ) ) ;
#21549=EDGE_CURVE ( 'NONE', #22218, #6732, #25781, .T. ) ;
#21557=CARTESIAN_POINT ( 'NONE',  ( 132.9375000000000284, -4.242640687119298093, -4.242640687119298093 ) ) ;
#21563=AXIS2_PLACEMENT_3D ( 'NONE', #23500, #20731, #18904 ) ;
#21565=CARTESIAN_POINT ( 'NONE',  ( -9.999999999999980460, -60.00000000000001421, 3.000000000000002665 ) ) ;
#21567=AXIS2_PLACEMENT_3D ( 'NONE', #12639, #19682, #1080 ) ;
#21570=( NAMED_UNIT ( * ) PLANE_ANGLE_UNIT ( ) SI_UNIT ( $, .RADIAN. ) );
#21571=EDGE_CURVE ( 'NONE', #20811, #4004, #22790, .T. ) ;
#21573=EDGE_CURVE ( 'NONE', #20381, #8862, #18951, .T. ) ;
#21577=CARTESIAN_POINT ( 'NONE',  ( 161.0000000000000284, 1.347111479062088799E-15, 11.00000000000000355 ) ) ;
#21581=CARTESIAN_POINT ( 'NONE',  ( 146.6398502691896510, -3.535533905932752852, 3.535533905932725318 ) ) ;
#21582=DIRECTION ( 'NONE',  ( 1.000000000000000000, 6.938893903907222067E-15, 0.000000000000000000 ) ) ;
#21583=CARTESIAN_POINT ( 'NONE',  ( 154.3125000000000284, 4.242640687119298093, -4.242640687119298093 ) ) ;
#21584=CARTESIAN_POINT ( 'NONE',  ( -0.5000000000000004441, -14.50000000000001243, -8.500000000000007105 ) ) ;
#21589=CIRCLE ( 'NONE', #19606, 0.5000000000000004441 ) ;
#21590=CARTESIAN_POINT ( 'NONE',  ( 151.0312500000000568, -2.485281374238555774, -6.000000000000005329 ) ) ;
#21591=CARTESIAN_POINT ( 'NONE',  ( -4.999999999999886313, -10.00000000000000888, 8.000000000000007105 ) ) ;
#21595=EDGE_LOOP ( 'NONE', ( #24831, #29991, #28807, #26839 ) ) ;
#21600=( BOUNDED_CURVE ( )  B_SPLINE_CURVE ( 2, ( #29441, #20097, #1651, #8414, #6109, #15521, #15001, #7909, #14436 ),
 .UNSPECIFIED., .F., .T. ) 
 B_SPLINE_CURVE_WITH_KNOTS ( ( 3, 2, 2, 2, 3 ),
 ( 0.2874999999999998113, 0.2937499999999995670, 0.2999999999999993783, 0.3062499999999991340, 0.3124999999999988898 ),
 .UNSPECIFIED. ) 
 CURVE ( )  GEOMETRIC_REPRESENTATION_ITEM ( )  RATIONAL_B_SPLINE_CURVE ( ( 1.000000000000001998, 0.9238795325112847401, 1.000000000000000000, 0.9238795325112867385, 1.000000000000000000, 0.9238795325112867385, 1.000000000000000000, 0.9238795325113002832, 0.9999999999999864553 ) ) 
 REPRESENTATION_ITEM ( '' )  );
#21603=FACE_OUTER_BOUND ( 'NONE', #5053, .T. ) ;
#21605=COLOUR_RGB ( '', 0.66274510, 0.83137255, 0.94901961) ;
#21607=CARTESIAN_POINT ( 'NONE',  ( 135.4056618780830092, -8.496329914204098444, 8.215405480166593222 ) ) ;
#21612=CARTESIAN_POINT ( 'NONE',  ( 135.0000000000000284, -6.982120021884474781, -8.500000000000007105 ) ) ;
#21619=CARTESIAN_POINT ( 'NONE',  ( 135.1800748654052029, -2.278174593051888408, 5.500000000000135891 ) ) ;
#21620=CARTESIAN_POINT ( 'NONE',  ( 157.0461002691896795, -2.071067811865468400, 4.999999999999989342 ) ) ;
#21621=DIRECTION ( 'NONE',  ( 1.000000000000000000, 0.000000000000000000, 0.000000000000000000 ) ) ;
#21627=EDGE_LOOP ( 'NONE', ( #22711, #5046, #2914, #7367 ) ) ;
#21628=DIRECTION ( 'NONE',  ( 0.000000000000000000, 0.000000000000000000, -1.000000000000000000 ) ) ;
#21633=ORIENTED_EDGE ( 'NONE', *, *, #15885, .F. ) ;
#21634=EDGE_CURVE ( 'NONE', #25526, #11814, #9607, .T. ) ;
#21641=CARTESIAN_POINT ( 'NONE',  ( 133.8601497308104342, -3.535533905932725318, -3.535533905932725318 ) ) ;
#21653=( LENGTH_UNIT ( ) NAMED_UNIT ( * ) SI_UNIT ( .MILLI., .METRE. ) );
#21657=FILL_AREA_STYLE_COLOUR ( '', #17583 ) ;
#21658=FACE_OUTER_BOUND ( 'NONE', #17675, .T. ) ;
#21659=CIRCLE ( 'NONE', #9393, 0.5000000000000004441 ) ;
#21662=CARTESIAN_POINT ( 'NONE',  ( 135.0000000000000284, 0.000000000000000000, 0.000000000000000000 ) ) ;
#21663=DIRECTION ( 'NONE',  ( 1.000000000000000000, 0.000000000000000000, -0.000000000000000000 ) ) ;
#21666=MECHANICAL_DESIGN_GEOMETRIC_PRESENTATION_REPRESENTATION('',(#25574),#14108);
#21674=CARTESIAN_POINT ( 'NONE',  ( 160.6875000000000284, 4.242640687119269671, 4.242640687119298093 ) ) ;
#21676=AXIS2_PLACEMENT_3D ( 'NONE', #18755, #4743, #1987 ) ;
#21679=AXIS2_PLACEMENT_3D ( 'NONE', #11717, #23666, #2743 ) ;
#21680=AXIS2_PLACEMENT_3D ( 'NONE', #7559, #26300, #5254 ) ;
#21682=CARTESIAN_POINT ( 'NONE',  ( 144.0074251345948539, 2.278174593051996322, -5.500000000000026645 ) ) ;
#21685=EDGE_CURVE ( 'NONE', #27377, #2648, #18960, .T. ) ;
#21688=CARTESIAN_POINT ( 'NONE',  ( 140.3288997308104058, 4.999999999999989342, -2.071067811865468400 ) ) ;
#21696=ORIENTED_EDGE ( 'NONE', *, *, #11584, .F. ) ;
#21699=DIRECTION ( 'NONE',  ( 0.000000000000000000, -0.3428396514843867759, 0.9393939393939395588 ) ) ;
#21712=CARTESIAN_POINT ( 'NONE',  ( 116.0000000000000142, 6.735557395310442023E-16, 5.500000000000000000 ) ) ;
#21715=CARTESIAN_POINT ( 'NONE',  ( 140.5000000000000284, -10.99818166789401275, -4.799999999999998934 ) ) ;
#21721=SURFACE_STYLE_FILL_AREA ( #19565 ) ;
#21722=CARTESIAN_POINT ( 'NONE',  ( -10.00000000000000178, -89.00000000000001421, -4.000000000000003553 ) ) ;
#21725=CARTESIAN_POINT ( 'NONE',  ( 139.9385832302453991, -9.134974910517927427, 7.783976842244119787 ) ) ;
#21728=SURFACE_STYLE_FILL_AREA ( #26606 ) ;
#21732=FILL_AREA_STYLE_COLOUR ( '', #11138 ) ;
#21733=CARTESIAN_POINT ( 'NONE',  ( 145.2336002691896795, -4.999999999999989342, 2.071067811865468400 ) ) ;
#21734=CARTESIAN_POINT ( 'NONE',  ( 150.0937500000000284, 6.000000000000005329, 2.485281374238585972 ) ) ;
#21739=ORIENTED_EDGE ( 'NONE', *, *, #11188, .T. ) ;
#21740=CARTESIAN_POINT ( 'NONE',  ( 142.9687500000000000, -2.485281374238585972, 6.000000000000005329 ) ) ;
#21743=UNCERTAINTY_MEASURE_WITH_UNIT (LENGTH_MEASURE( 1.000000000000000082E-05 ), #19254, 'distance_accuracy_value', 'NONE');
#21756=CARTESIAN_POINT ( 'NONE',  ( 135.0029060396470300, -6.966976446535451117, 8.000000000000007105 ) ) ;
#21758=CARTESIAN_POINT ( 'NONE',  ( 160.5074251345948255, 2.278174593052136210, -5.499999999999888978 ) ) ;
#21760=CARTESIAN_POINT ( 'NONE',  ( -4.999999999999990230, -55.00000000000002132, -7.500000000000007105 ) ) ;
#21765=CARTESIAN_POINT ( 'NONE',  ( 155.9136751345948539, 0.000000000000000000, -5.500000000000005329 ) ) ;
#21768=LINE ( 'NONE', #28798, #2133 ) ;
#21771=ORIENTED_EDGE ( 'NONE', *, *, #28023, .T. ) ;
#21777=EDGE_CURVE ( 'NONE', #17671, #14644, #20293, .T. ) ;
#21779=CARTESIAN_POINT ( 'NONE',  ( 145.6875000000000284, 4.242640687119269671, 4.242640687119298093 ) ) ;
#21791=DIRECTION ( 'NONE',  ( -1.000000000000000000, 0.000000000000000000, 0.000000000000000000 ) ) ;
#21792=CARTESIAN_POINT ( 'NONE',  ( 141.2738248654052313, -3.889087296526011706, 3.889087296526011706 ) ) ;
#21796=B_SPLINE_CURVE_WITH_KNOTS ( 'NONE', 3,
 ( #15820, #27419, #6704, #11349, #6386, #29592, #30202, #4083 ),
 .UNSPECIFIED., .F., .F.,
 ( 4, 2, 2, 4 ),
 ( 0.000000000000000000, 0.0002342670595278595010, 0.0003514005892917859177, 0.0004685341190557123343 ),
 .UNSPECIFIED. ) ;
#21802=CARTESIAN_POINT ( 'NONE',  ( 1.000000000000000888, -16.43939393939394833, -5.999693900976793337 ) ) ;
#21803=CARTESIAN_POINT ( 'NONE',  ( 148.9761751345948255, 3.889087296526011706, 3.889087296526011706 ) ) ;
#21805=EDGE_CURVE ( 'NONE', #452, #30157, #28115, .T. ) ;
#21807=CARTESIAN_POINT ( 'NONE',  ( 15.00000000000000000, 0.000000000000000000, -16.50000000000000355 ) ) ;
#21810=DIRECTION ( 'NONE',  ( 0.000000000000000000, 0.000000000000000000, -1.000000000000000000 ) ) ;
#21814=EDGE_CURVE ( 'NONE', #3203, #20658, #21119, .T. ) ;
#21815=ORIENTED_EDGE ( 'NONE', *, *, #27470, .T. ) ;
#21817=CARTESIAN_POINT ( 'NONE',  ( 132.4687500000000284, -2.485281374238585972, 6.000000000000005329 ) ) ;
#21818=CARTESIAN_POINT ( 'NONE',  ( 160.0312500000000284, -2.485281374238555774, -6.000000000000005329 ) ) ;
#21821=CARTESIAN_POINT ( 'NONE',  ( 157.2113248654052313, 5.500000000000005329, 0.000000000000000000 ) ) ;
#21825=CARTESIAN_POINT ( 'NONE',  ( 144.4761751345948255, 3.889087296526011706, 3.889087296526011706 ) ) ;
#21826=ORIENTED_EDGE ( 'NONE', *, *, #436, .F. ) ;
#21829=CARTESIAN_POINT ( 'NONE',  ( -19.99999999999998224, -54.99999999999990763, 5.000000000000004441 ) ) ;
#21830=CARTESIAN_POINT ( 'NONE',  ( 137.1413997308104342, 2.071067811865468400, -4.999999999999989342 ) ) ;
#21831=CARTESIAN_POINT ( 'NONE',  ( 138.0863248654052313, 0.000000000000000000, 5.500000000000005329 ) ) ;
#21833=CARTESIAN_POINT ( 'NONE',  ( -4.999999999999886313, -15.00000000000001421, -7.500000000000007105 ) ) ;
#21834=FACE_OUTER_BOUND ( 'NONE', #4601, .T. ) ;
#21842=CARTESIAN_POINT ( 'NONE',  ( -10.00000000000000178, -19.99999999999998934, 4.000000000000003553 ) ) ;
#21849=ADVANCED_FACE ( 'NONE', ( #3373 ), #10322, .T. ) ;
#21850=DIRECTION ( 'NONE',  ( 0.000000000000000000, 0.000000000000000000, -1.000000000000000000 ) ) ;
#21852=CARTESIAN_POINT ( 'NONE',  ( 140.8531441848278689, -11.85314418482570353, 4.000138456839522405 ) ) ;
#21855=CARTESIAN_POINT ( 'NONE',  ( 160.8911125001014284, -11.51406693544466009, 3.382303552187507112 ) ) ;
#21856=AXIS2_PLACEMENT_3D ( 'NONE', #27869, #23450, #22987 ) ;
#21864=LINE ( 'NONE', #26449, #54 ) ;
#21866=( LENGTH_UNIT ( ) NAMED_UNIT ( * ) SI_UNIT ( .MILLI., .METRE. ) );
#21871=CARTESIAN_POINT ( 'NONE',  ( 140.0000000000000000, -9.910236803014807805, 7.559842130755045631 ) ) ;
#21877=DIRECTION ( 'NONE',  ( 1.000000000000000000, -0.000000000000000000, -0.000000000000000000 ) ) ;
#21879=CARTESIAN_POINT ( 'NONE',  ( 139.0461002691896510, -2.071067811865468400, 4.999999999999989342 ) ) ;
#21880=CARTESIAN_POINT ( 'NONE',  ( 152.0625000000000568, -4.242640687119298093, 4.242640687119298093 ) ) ;
#21887=CARTESIAN_POINT ( 'NONE',  ( 144.1875000000000284, 4.242640687119269671, 4.242640687119298093 ) ) ;
#21897=CIRCLE ( 'NONE', #18983, 12.00000000000000178 ) ;
#21899=COLOUR_RGB ( '', 0.66274510, 0.83137255, 0.94901961) ;
#21900=VERTEX_POINT ( 'NONE', #3079 ) ;
#21902=VECTOR ( 'NONE', #12422, 1000.000000000000000 ) ;
#21904=CYLINDRICAL_SURFACE ( 'NONE', #14273, 1.000000000000000000 ) ;
#21909=EDGE_CURVE ( 'NONE', #2895, #25883, #27118, .T. ) ;
#21917=DIRECTION ( 'NONE',  ( -0.000000000000000000, -0.000000000000000000, -1.000000000000000000 ) ) ;
#21918=( LENGTH_UNIT ( ) NAMED_UNIT ( * ) SI_UNIT ( .MILLI., .METRE. ) );
#21919=EDGE_CURVE ( 'NONE', #6626, #30104, #24671, .T. ) ;
#21921=FILL_AREA_STYLE_COLOUR ( '', #5724 ) ;
#21926=CARTESIAN_POINT ( 'NONE',  ( 147.5625000000000284, -4.242640687119298093, 4.242640687119298093 ) ) ;
#21933=CARTESIAN_POINT ( 'NONE',  ( 146.9136751345948539, 0.000000000000000000, -5.500000000000005329 ) ) ;
#21939=CIRCLE ( 'NONE', #23915, 1.000000000000000000 ) ;
#21942=CARTESIAN_POINT ( 'NONE',  ( 152.9925748654052029, 2.278174593051965235, 5.500000000000058620 ) ) ;
#21944=DIRECTION ( 'NONE',  ( 0.000000000000000000, 0.000000000000000000, 1.000000000000000000 ) ) ;
#21948=CARTESIAN_POINT ( 'NONE',  ( 135.9026099654455493, -8.798545334315235777, 8.160000000000003695 ) ) ;
#21958=ORIENTED_EDGE ( 'NONE', *, *, #6887, .F. ) ;
#21960=( NAMED_UNIT ( * ) SI_UNIT ( $, .STERADIAN. ) SOLID_ANGLE_UNIT ( ) );
#21964=VERTEX_POINT ( 'NONE', #29336 ) ;
#21965=CARTESIAN_POINT ( 'NONE',  ( 134.2648502691896510, 3.535533905932725318, 3.535533905932752852 ) ) ;
#21966=ORIENTED_EDGE ( 'NONE', *, *, #9332, .T. ) ;
#21976=FILL_AREA_STYLE_COLOUR ( '', #14262 ) ;
#21977=CARTESIAN_POINT ( 'NONE',  ( 136.9538997308104058, -2.071067811865468400, -4.999999999999989342 ) ) ;
#21994=CARTESIAN_POINT ( 'NONE',  ( 135.0000000000000284, 5.838252472155780914, -1.149616569750068207 ) ) ;
#21995=CARTESIAN_POINT ( 'NONE',  ( 155.6324251345948255, -5.500000000000012434, -2.278174593052012309 ) ) ;
#21997=SURFACE_STYLE_USAGE ( .BOTH. , #22153 ) ;
#21998=CARTESIAN_POINT ( 'NONE',  ( 141.0863248654052313, 0.000000000000000000, 5.500000000000005329 ) ) ;
#21999=VERTEX_POINT ( 'NONE', #17706 ) ;
#22007=CARTESIAN_POINT ( 'NONE',  ( 157.5788997308104058, -4.999999999999989342, 2.071067811865468400 ) ) ;
#22010=( LENGTH_UNIT ( ) NAMED_UNIT ( * ) SI_UNIT ( .MILLI., .METRE. ) );
#22020=ORIENTED_EDGE ( 'NONE', *, *, #20179, .T. ) ;
#22021=CARTESIAN_POINT ( 'NONE',  ( 142.3273502691896510, -5.000000000000004441, 0.000000000000000000 ) ) ;
#22022=CARTESIAN_POINT ( 'NONE',  ( 152.8125000000000568, 4.242640687119298093, -4.242640687119298093 ) ) ;
#22028=CARTESIAN_POINT ( 'NONE',  ( 141.2812500000000284, 2.485281374238585972, 6.000000000000005329 ) ) ;
#22030=CIRCLE ( 'NONE', #21093, 0.5000000000000004441 ) ;
#22031=( BOUNDED_CURVE ( )  B_SPLINE_CURVE ( 2, ( #10699, #22514, #15147, #11005, #24479, #17922, #27239, #29231, #1601 ),
 .UNSPECIFIED., .F., .F. ) 
 B_SPLINE_CURVE_WITH_KNOTS ( ( 3, 2, 2, 2, 3 ),
 ( 0.4374999999999999445, 0.4437500000000001443, 0.4500000000000003997, 0.4562500000000006550, 0.4625000000000009104 ),
 .UNSPECIFIED. ) 
 CURVE ( )  GEOMETRIC_REPRESENTATION_ITEM ( )  RATIONAL_B_SPLINE_CURVE ( ( 1.000000000000000666, 0.9238795325112860723, 1.000000000000000000, 0.9238795325112867385, 1.000000000000000000, 0.9238795325112867385, 1.000000000000000000, 0.9238795325112759693, 1.000000000000010880 ) ) 
 REPRESENTATION_ITEM ( '' )  );
#22037=ORIENTED_EDGE ( 'NONE', *, *, #27810, .F. ) ;
#22043=SURFACE_SIDE_STYLE ('',( #12707 ) ) ;
#22044=DIRECTION ( 'NONE',  ( 1.000000000000000000, 0.000000000000000000, 0.000000000000000000 ) ) ;
#22045=CARTESIAN_POINT ( 'NONE',  ( 135.0710545211900353, -7.730464060720690256, -8.358520852376209120 ) ) ;
#22046=CARTESIAN_POINT ( 'NONE',  ( 124.9999999999999432, -70.00000000000000000, -7.500000000000007105 ) ) ;
#22049=EDGE_CURVE ( 'NONE', #6232, #20568, #175, .T. ) ;
#22054=AXIS2_PLACEMENT_3D ( 'NONE', #19157, #26627, #28493 ) ;
#22056=CARTESIAN_POINT ( 'NONE',  ( 141.9300748654051745, 2.278174593051702335, -5.500000000000323297 ) ) ;
#22060=CARTESIAN_POINT ( 'NONE',  ( 135.2738248654052313, -3.889087296526011706, 3.889087296526011706 ) ) ;
#22061=CARTESIAN_POINT ( 'NONE',  ( 139.6830278787118402, -9.225297888154202042, -7.967375165638989287 ) ) ;
#22063=CIRCLE ( 'NONE', #26997, 1.000000000000000222 ) ;
#22067=ORIENTED_EDGE ( 'NONE', *, *, #10363, .T. ) ;
#22068=CARTESIAN_POINT ( 'NONE',  ( 161.3437500000000568, -6.000000000000005329, -2.485281374238555774 ) ) ;
#22069=CARTESIAN_POINT ( 'NONE',  ( 140.5000000000000284, -11.45643923738959202, 5.000000000000004441 ) ) ;
#22073=ORIENTED_EDGE ( 'NONE', *, *, #9983, .T. ) ;
#22077=AXIS2_PLACEMENT_3D ( 'NONE', #4236, #25425, #17957 ) ;
#22081=VECTOR ( 'NONE', #16864, 1000.000000000000000 ) ;
#22087=EDGE_CURVE ( 'NONE', #9038, #4270, #21768, .T. ) ;
#22090=CARTESIAN_POINT ( 'NONE',  ( 155.8050748654052313, 5.500000000000012434, 2.278174593052012309 ) ) ;
#22095=CARTESIAN_POINT ( 'NONE',  ( -0.6046674458933997132, -9.395332554106689216, 4.067501169440991049 ) ) ;
#22099=CARTESIAN_POINT ( 'NONE',  ( 135.2583738898383103, -8.263074927440506201, 8.258625120961028188 ) ) ;
#22101=LINE ( 'NONE', #1178, #15330 ) ;
#22102=CARTESIAN_POINT ( 'NONE',  ( 135.0000000000000284, -8.500000000000007105, 8.000000000000007105 ) ) ;
#22114=EDGE_LOOP ( 'NONE', ( #2165, #27473, #12969, #27633 ) ) ;
#22116=CARTESIAN_POINT ( 'NONE',  ( 132.5773502691896510, 5.000000000000004441, 0.000000000000000000 ) ) ;
#22118=EDGE_CURVE ( 'NONE', #3951, #11992, #28504, .T. ) ;
#22119=VERTEX_POINT ( 'NONE', #14716 ) ;
#22126=CARTESIAN_POINT ( 'NONE',  ( 1.000000000000000888, -16.43939393939395188, -5.999693900976774685 ) ) ;
#22127=DIRECTION ( 'NONE',  ( 1.000000000000000000, 0.000000000000000000, 0.000000000000000000 ) ) ;
#22128=FACE_OUTER_BOUND ( 'NONE', #5063, .T. ) ;
#22129=AXIS2_PLACEMENT_3D ( 'NONE', #17779, #5443, #3292 ) ;
#22130=CARTESIAN_POINT ( 'NONE',  ( 135.0000000000000284, -9.047800747817552391, 7.500000000000007105 ) ) ;
#22131=CARTESIAN_POINT ( 'NONE',  ( 0.9563234411482145481, -15.26191353904648551, -8.566444784294999337 ) ) ;
#22134=DIRECTION ( 'NONE',  ( 0.000000000000000000, 0.000000000000000000, -1.000000000000000000 ) ) ;
#22148=CIRCLE ( 'NONE', #1518, 0.5000000000000004441 ) ;
#22149=FILL_AREA_STYLE ('',( #15095 ) ) ;
#22150=DIRECTION ( 'NONE',  ( 1.000000000000000000, 0.000000000000000000, 0.000000000000000000 ) ) ;
#22152=AXIS2_PLACEMENT_3D ( 'NONE', #29292, #17211, #15373 ) ;
#22153=SURFACE_SIDE_STYLE ('',( #3384 ) ) ;
#22154=CARTESIAN_POINT ( 'NONE',  ( 140.3637585460053572, -11.68187927300244411, 4.222310544175132740 ) ) ;
#22155=ADVANCED_FACE ( 'NONE', ( #3004 ), #10470, .F. ) ;
#22158=CARTESIAN_POINT ( 'NONE',  ( 159.5094690746824142, -11.10052039921582079, 4.558404387674897862 ) ) ;
#22164=CARTESIAN_POINT ( 'NONE',  ( 152.8913997308104626, -2.071067811865468400, 4.999999999999989342 ) ) ;
#22169=CARTESIAN_POINT ( 'NONE',  ( 135.4369124609227129, -8.875665394635735339, 8.012677223695028772 ) ) ;
#22172=DIRECTION ( 'NONE',  ( -0.000000000000000000, -0.000000000000000000, -1.000000000000000000 ) ) ;
#22176=SURFACE_SIDE_STYLE ('',( #5268 ) ) ;
#22178=CARTESIAN_POINT ( 'NONE',  ( 153.4687500000000853, -2.485281374238585972, 6.000000000000005329 ) ) ;
#22180=AXIS2_PLACEMENT_3D ( 'NONE', #29211, #1582, #8173 ) ;
#22185=CARTESIAN_POINT ( 'NONE',  ( 145.5937500000000284, 6.000000000000005329, 2.485281374238585972 ) ) ;
#22186=CARTESIAN_POINT ( 'NONE',  ( 161.3871073408037375, -5.626013716664558295, -1.762305681933894475 ) ) ;
#22192=ORIENTED_EDGE ( 'NONE', *, *, #6044, .F. ) ;
#22199=FACE_OUTER_BOUND ( 'NONE', #8779, .T. ) ;
#22200=CARTESIAN_POINT ( 'NONE',  ( 135.9026387045187221, -8.798545334315203803, -8.160000000000000142 ) ) ;
#22201=DIRECTION ( 'NONE',  ( -1.000000000000000000, 0.000000000000000000, 0.000000000000000000 ) ) ;
#22205=CARTESIAN_POINT ( 'NONE',  ( 134.9999999999999432, 5.815044816414753015, 1.151864612277130551 ) ) ;
#22208=DIRECTION ( 'NONE',  ( 0.000000000000000000, -1.000000000000000000, 0.000000000000000000 ) ) ;
#22211=CARTESIAN_POINT ( 'NONE',  ( 152.5461002691896795, -2.071067811865468400, 4.999999999999989342 ) ) ;
#22214=EDGE_CURVE ( 'NONE', #3609, #25966, #27101, .T. ) ;
#22218=VERTEX_POINT ( 'NONE', #7180 ) ;
#22219=CARTESIAN_POINT ( 'NONE',  ( 160.5937500000000284, 6.000000000000005329, 2.485281374238585972 ) ) ;
#22224=EDGE_CURVE ( 'NONE', #22958, #15258, #22229, .T. ) ;
#22227=CARTESIAN_POINT ( 'NONE',  ( -14.99999999999999289, -54.99999999999990763, 7.500000000000007105 ) ) ;
#22229=CIRCLE ( 'NONE', #20761, 12.50000000000000178 ) ;
#22235=VERTEX_POINT ( 'NONE', #21320 ) ;
#22237=CARTESIAN_POINT ( 'NONE',  ( 116.0000000000000142, 0.000000000000000000, -5.500000000000000000 ) ) ;
#22247=LINE ( 'NONE', #8242, #21279 ) ;
#22249=FACE_OUTER_BOUND ( 'NONE', #27272, .T. ) ;
#22250=( NAMED_UNIT ( * ) SI_UNIT ( $, .STERADIAN. ) SOLID_ANGLE_UNIT ( ) );
#22251=CARTESIAN_POINT ( 'NONE',  ( 130.0000000000000284, -60.00000000000001421, 4.000000000000003553 ) ) ;
#22256=CARTESIAN_POINT ( 'NONE',  ( 143.3363248654052029, 0.000000000000000000, -5.500000000000005329 ) ) ;
#22259=CARTESIAN_POINT ( 'NONE',  ( 135.5000000000000000, -9.047800747817552391, 7.500000000000007105 ) ) ;
#22260=CIRCLE ( 'NONE', #19796, 14.49999999999999822 ) ;
#22266=VERTEX_POINT ( 'NONE', #22369 ) ;
#22267=CARTESIAN_POINT ( 'NONE',  ( 155.0625000000000284, -4.242640687119298093, 4.242640687119298093 ) ) ;
#22268=B_SPLINE_CURVE_WITH_KNOTS ( 'NONE', 3,
 ( #19115, #12366, #7420, #21715 ),
 .UNSPECIFIED., .F., .F.,
 ( 4, 4 ),
 ( 0.000000000000000000, 0.0002043583609089599416 ),
 .UNSPECIFIED. ) ;
#22270=VERTEX_POINT ( 'NONE', #10869 ) ;
#22279=( LENGTH_UNIT ( ) NAMED_UNIT ( * ) SI_UNIT ( .MILLI., .METRE. ) );
#22281=CARTESIAN_POINT ( 'NONE',  ( 139.7738248654052313, -3.889087296526011706, 3.889087296526011706 ) ) ;
#22287=CARTESIAN_POINT ( 'NONE',  ( 1.000000000000000888, -15.50000000000001421, 5.656854249492387687 ) ) ;
#22291=ORIENTED_EDGE ( 'NONE', *, *, #7847, .F. ) ;
#22294=CARTESIAN_POINT ( 'NONE',  ( 160.1175748654052029, 5.500000000000012434, -2.278174593052012309 ) ) ;
#22302=CARTESIAN_POINT ( 'NONE',  ( 116.0000000000000142, 0.000000000000000000, -5.500000000000000000 ) ) ;
#22305=VECTOR ( 'NONE', #28941, 1000.000000000000000 ) ;
#22308=CARTESIAN_POINT ( 'NONE',  ( 160.2036198215142520, -11.22298632203329483, 4.248469099170785412 ) ) ;
#22313=( BOUNDED_CURVE ( )  B_SPLINE_CURVE ( 2, ( #28098, #14336, #23673, #14615, #307, #5052, #14762, #19079, #1639 ),
 .UNSPECIFIED., .F., .T. ) 
 B_SPLINE_CURVE_WITH_KNOTS ( ( 3, 2, 2, 2, 3 ),
 ( 0.8124999999999993339, 0.8187499999999995337, 0.8249999999999997335, 0.8312500000000000444, 0.8375000000000002442 ),
 .UNSPECIFIED. ) 
 CURVE ( )  GEOMETRIC_REPRESENTATION_ITEM ( )  RATIONAL_B_SPLINE_CURVE ( ( 1.000000000000008216, 0.9238795325112786339, 1.000000000000000000, 0.9238795325112867385, 1.000000000000000000, 0.9238795325112867385, 1.000000000000000000, 0.9238795325112840739, 1.000000000000002665 ) ) 
 REPRESENTATION_ITEM ( '' )  );
#22315=CARTESIAN_POINT ( 'NONE',  ( 149.4226497308104058, 5.000000000000004441, 0.000000000000000000 ) ) ;
#22316=CARTESIAN_POINT ( 'NONE',  ( -4.999999999999990230, -14.50000000000001243, -8.000000000000007105 ) ) ;
#22319=DIRECTION ( 'NONE',  ( 0.000000000000000000, 0.000000000000000000, -1.000000000000000000 ) ) ;
#22324=EDGE_LOOP ( 'NONE', ( #27911, #30375, #29693, #10324 ) ) ;
#22331=CARTESIAN_POINT ( 'NONE',  ( 148.2187500000000284, 2.485281374238556218, -6.000000000000005329 ) ) ;
#22336=VERTEX_POINT ( 'NONE', #12572 ) ;
#22337=CARTESIAN_POINT ( 'NONE',  ( 143.6250000000000284, 0.000000000000000000, -6.000000000000005329 ) ) ;
#22340=VECTOR ( 'NONE', #14250, 1000.000000000000000 ) ;
#22350=LINE ( 'NONE', #27237, #27512 ) ;
#22351=EDGE_CURVE ( 'NONE', #13456, #8510, #21256, .T. ) ;
#22359=UNCERTAINTY_MEASURE_WITH_UNIT (LENGTH_MEASURE( 1.000000000000000082E-05 ), #2079, 'distance_accuracy_value', 'NONE');
#22365=CARTESIAN_POINT ( 'NONE',  ( 154.4211002691896510, -4.999999999999989342, -2.071067811865468400 ) ) ;
#22368=CARTESIAN_POINT ( 'NONE',  ( 144.5550748654052029, -5.500000000000012434, -2.278174593052012309 ) ) ;
#22369=CARTESIAN_POINT ( 'NONE',  ( 0.000000000000000000, -9.500000000000008882, -5.000000000000004441 ) ) ;
#22372=VERTEX_POINT ( 'NONE', #26948 ) ;
#22385=EDGE_CURVE ( 'NONE', #12702, #22602, #24655, .T. ) ;
#22390=DIRECTION ( 'NONE',  ( -0.000000000000000000, -0.000000000000000000, -1.000000000000000000 ) ) ;
#22395=PRESENTATION_STYLE_ASSIGNMENT (( #29896 ) ) ;
#22397=CARTESIAN_POINT ( 'NONE',  ( -0.4963810631259263917, -9.251809468437068418, 4.126213593628771825 ) ) ;
#22403=EDGE_CURVE ( 'NONE', #19367, #12929, #15950, .T. ) ;
#22406=CARTESIAN_POINT ( 'NONE',  ( 135.0000000000000284, -8.789428240781155921, 7.941267209061672716 ) ) ;
#22420=CARTESIAN_POINT ( 'NONE',  ( 159.0937500000000284, 6.000000000000005329, 2.485281374238585972 ) ) ;
#22424=CARTESIAN_POINT ( 'NONE',  ( 161.1037658773653050, -2.857005778783127844E-13, 5.603765877365280090 ) ) ;
#22426=CARTESIAN_POINT ( 'NONE',  ( 116.0000000000000142, 0.000000000000000000, 0.000000000000000000 ) ) ;
#22429=CARTESIAN_POINT ( 'NONE',  ( 159.3361461291012517, -11.35074521425119620, 3.948316470164734415 ) ) ;
#22434=CARTESIAN_POINT ( 'NONE',  ( 140.5835741348633690, -11.79178706743166494, 4.000000000000005329 ) ) ;
#22441=CARTESIAN_POINT ( 'NONE',  ( 0.7669223171414760731, -15.58766199952932396, 7.954545454545463912 ) ) ;
#22443=DIRECTION ( 'NONE',  ( -0.000000000000000000, -0.000000000000000000, -1.000000000000000000 ) ) ;
#22449=ORIENTED_EDGE ( 'NONE', *, *, #27396, .T. ) ;
#22455=AXIS2_PLACEMENT_3D ( 'NONE', #16909, #587, #9974 ) ;
#22463=CARTESIAN_POINT ( 'NONE',  ( 143.2500000000000568, -6.000000000000005329, 0.000000000000000000 ) ) ;
#22471=CARTESIAN_POINT ( 'NONE',  ( 135.8344003793655190, -8.798545317545935163, -8.160000018081550621 ) ) ;
#22472=CARTESIAN_POINT ( 'NONE',  ( 152.3288997308104058, 4.999999999999989342, -2.071067811865468400 ) ) ;
#22475=DIRECTION ( 'NONE',  ( 0.000000000000000000, 1.000000000000000000, -0.000000000000000000 ) ) ;
#22479=EDGE_CURVE ( 'NONE', #18033, #27766, #20881, .T. ) ;
#22484=STYLED_ITEM ( 'NONE', ( #19356 ), #3263 ) ;
#22485=CARTESIAN_POINT ( 'NONE',  ( 116.0000000000000142, 0.000000000000000000, 0.000000000000000000 ) ) ;
#22486=ORIENTED_EDGE ( 'NONE', *, *, #13379, .T. ) ;
#22488=CARTESIAN_POINT ( 'NONE',  ( -4.999999999999990230, -24.99999999999999289, 4.000000000000003553 ) ) ;
#22490=ORIENTED_EDGE ( 'NONE', *, *, #4699, .F. ) ;
#22492=CARTESIAN_POINT ( 'NONE',  ( 148.3125000000000284, 4.242640687119298093, -4.242640687119298093 ) ) ;
#22496=ORIENTED_EDGE ( 'NONE', *, *, #6846, .F. ) ;
#22497=CARTESIAN_POINT ( 'NONE',  ( 138.3750000000000284, 0.000000000000000000, 6.000000000000005329 ) ) ;
#22498=CARTESIAN_POINT ( 'NONE',  ( 161.3624454948340485, -5.811493806601979450, -0.8339435799521033310 ) ) ;
#22501=( BOUNDED_CURVE ( )  B_SPLINE_CURVE ( 2, ( #3291, #14431, #17165, #12717, #12125, #7464, #5294, #22056, #21469 ),
 .UNSPECIFIED., .F., .T. ) 
 B_SPLINE_CURVE_WITH_KNOTS ( ( 3, 2, 2, 2, 3 ),
 ( 0.6375000000000001776, 0.6437500000000004885, 0.6500000000000006883, 0.6562500000000008882, 0.6625000000000010880 ),
 .UNSPECIFIED. ) 
 CURVE ( )  GEOMETRIC_REPRESENTATION_ITEM ( )  RATIONAL_B_SPLINE_CURVE ( ( 0.9999999999999973355, 0.9238795325112894030, 1.000000000000000000, 0.9238795325112867385, 1.000000000000000000, 0.9238795325112867385, 1.000000000000000000, 0.9238795325112731938, 1.000000000000013545 ) ) 
 REPRESENTATION_ITEM ( '' )  );
#22507=EDGE_CURVE ( 'NONE', #20198, #24855, #16606, .T. ) ;
#22508=ADVANCED_FACE ( 'NONE', ( #29870 ), #6528, .F. ) ;
#22510=ORIENTED_EDGE ( 'NONE', *, *, #5378, .F. ) ;
#22511=CIRCLE ( 'NONE', #26407, 16.00000000000000000 ) ;
#22514=CARTESIAN_POINT ( 'NONE',  ( 148.4925748654052313, 2.278174593051996322, 5.500000000000026645 ) ) ;
#22525=LINE ( 'NONE', #6222, #29519 ) ;
#22526=CARTESIAN_POINT ( 'NONE',  ( 161.0438449402356866, -5.397155697456622825, -1.336872040267217177 ) ) ;
#22531=ORIENTED_EDGE ( 'NONE', *, *, #7373, .F. ) ;
#22541=ORIENTED_EDGE ( 'NONE', *, *, #22677, .T. ) ;
#22543=( LENGTH_UNIT ( ) NAMED_UNIT ( * ) SI_UNIT ( .MILLI., .METRE. ) );
#22547=ORIENTED_EDGE ( 'NONE', *, *, #14228, .T. ) ;
#22550=AXIS2_PLACEMENT_3D ( 'NONE', #20422, #3969, #6431 ) ;
#22551=CARTESIAN_POINT ( 'NONE',  ( 146.7261751345948539, -3.889087296526011706, -3.889087296526011706 ) ) ;
#22555=SURFACE_STYLE_FILL_AREA ( #29745 ) ;
#22556=CARTESIAN_POINT ( 'NONE',  ( -0.6927266194436426661, -9.614546761112704232, 4.200333198739607532 ) ) ;
#22560=SURFACE_STYLE_FILL_AREA ( #10753 ) ;
#22562=DIRECTION ( 'NONE',  ( -0.000000000000000000, -0.000000000000000000, -1.000000000000000000 ) ) ;
#22569=DIRECTION ( 'NONE',  ( 0.000000000000000000, 0.000000000000000000, -1.000000000000000000 ) ) ;
#22573=LINE ( 'NONE', #6410, #2359 ) ;
#22576=AXIS2_PLACEMENT_3D ( 'NONE', #8765, #15405, #27463 ) ;
#22579=CARTESIAN_POINT ( 'NONE',  ( 154.2187500000000284, 2.485281374238555774, -6.000000000000005329 ) ) ;
#22587=DIRECTION ( 'NONE',  ( -0.000000000000000000, -0.000000000000000000, -1.000000000000000000 ) ) ;
#22591=CARTESIAN_POINT ( 'NONE',  ( 159.8945522408903344, -11.49011212213293831, -3.498496789343953139 ) ) ;
#22602=VERTEX_POINT ( 'NONE', #11593 ) ;
#22604=AXIS2_PLACEMENT_3D ( 'NONE', #11088, #1690, #15874 ) ;
#22607=CARTESIAN_POINT ( 'NONE',  ( 140.7336002691896795, -4.999999999999989342, 2.071067811865468400 ) ) ;
#22608=ORIENTED_EDGE ( 'NONE', *, *, #3574, .F. ) ;
#22616=VERTEX_POINT ( 'NONE', #2343 ) ;
#22617=DIRECTION ( 'NONE',  ( -1.000000000000000000, -0.000000000000000000, -0.000000000000000000 ) ) ;
#22618=CARTESIAN_POINT ( 'NONE',  ( 141.1875000000000284, 4.242640687119269671, 4.242640687119298093 ) ) ;
#22619=COLOUR_RGB ( '', 0.08235294, 0.09019608, 0.10196078) ;
#22626=( NAMED_UNIT ( * ) PLANE_ANGLE_UNIT ( ) SI_UNIT ( $, .RADIAN. ) );
#22627=DIRECTION ( 'NONE',  ( -0.000000000000000000, 0.000000000000000000, 1.000000000000000000 ) ) ;
#22629=CARTESIAN_POINT ( 'NONE',  ( 151.1101497308104058, 3.535533905932725318, 3.535533905932725318 ) ) ;
#22634=EDGE_LOOP ( 'NONE', ( #22486, #20232, #27285, #26682 ) ) ;
#22637=CARTESIAN_POINT ( 'NONE',  ( 1.000000000000000888, 0.000000000000000000, 0.000000000000000000 ) ) ;
#22640=ORIENTED_EDGE ( 'NONE', *, *, #27092, .T. ) ;
#22642=CARTESIAN_POINT ( 'NONE',  ( 148.5000000000000284, 6.000000000000005329, 0.000000000000000000 ) ) ;
#22643=CARTESIAN_POINT ( 'NONE',  ( -4.999999999999886313, -9.000000000000007105, 4.000000000000003553 ) ) ;
#22644=CIRCLE ( 'NONE', #2024, 14.49999999999998579 ) ;
#22645=EDGE_CURVE ( 'NONE', #9814, #8182, #3568, .T. ) ;
#22646=CARTESIAN_POINT ( 'NONE',  ( 140.0769230769231228, -11.53846153846155254, -4.615384615384604317 ) ) ;
#22648=CARTESIAN_POINT ( 'NONE',  ( 139.5937500000000284, 6.000000000000005329, 2.485281374238585972 ) ) ;
#22649=CARTESIAN_POINT ( 'NONE',  ( 161.1633582548628567, -2.175497436150891417, 5.238395570785098876 ) ) ;
#22651=EDGE_CURVE ( 'NONE', #20198, #22270, #18795, .T. ) ;
#22654=ORIENTED_EDGE ( 'NONE', *, *, #6677, .F. ) ;
#22664=CARTESIAN_POINT ( 'NONE',  ( 0.000000000000000000, -14.14213562373095634, -8.500000000000007105 ) ) ;
#22665=AXIS2_PLACEMENT_3D ( 'NONE', #26306, #9748, #23868 ) ;
#22670=DIRECTION ( 'NONE',  ( 1.000000000000000000, -0.000000000000000000, -0.000000000000000000 ) ) ;
#22671=CARTESIAN_POINT ( 'NONE',  ( 154.1398502691896510, -3.535533905932752852, 3.535533905932725318 ) ) ;
#22675=CARTESIAN_POINT ( 'NONE',  ( 140.7917870674316987, -11.58357413486331566, -4.000000000000005329 ) ) ;
#22676=AXIS2_PLACEMENT_3D ( 'NONE', #4394, #4089, #27886 ) ;
#22677=EDGE_CURVE ( 'NONE', #20342, #16115, #22779, .T. ) ;
#22684=CARTESIAN_POINT ( 'NONE',  ( 156.4687500000000284, -2.485281374238585972, 6.000000000000005329 ) ) ;
#22685=DIRECTION ( 'NONE',  ( -0.000000000000000000, -0.4000000000000005773, -0.9165151389911678770 ) ) ;
#22688=EDGE_LOOP ( 'NONE', ( #19001, #22724, #17185, #17534 ) ) ;
#22689=EDGE_LOOP ( 'NONE', ( #16901, #12301, #9544 ) ) ;
#22695=CARTESIAN_POINT ( 'NONE',  ( 139.7945697293052660, -8.829120115006070080, -8.127272355818778493 ) ) ;
#22699=B_SPLINE_CURVE_WITH_KNOTS ( 'NONE', 3,
 ( #12676, #3708, #22169, #15439, #8323, #1103, #10501, #19854, #10977, #27210, #5554, #8163 ),
 .UNSPECIFIED., .F., .F.,
 ( 4, 2, 2, 2, 2, 4 ),
 ( 0.000000000000000000, 0.0002753300403215867896, 0.0005506600806431735792, 0.001101320161286347158, 0.001651980241929520629, 0.002202640322572694317 ),
 .UNSPECIFIED. ) ;
#22700=SURFACE_SIDE_STYLE ('',( #30207 ) ) ;
#22707=CARTESIAN_POINT ( 'NONE',  ( 145.5863248654052313, 0.000000000000000000, 5.500000000000005329 ) ) ;
#22711=ORIENTED_EDGE ( 'NONE', *, *, #18246, .F. ) ;
#22714=DIRECTION ( 'NONE',  ( 1.000000000000000000, -0.000000000000000000, -0.000000000000000000 ) ) ;
#22719=CARTESIAN_POINT ( 'NONE',  ( 135.6566535407617948, -9.123793365789319765, 8.000000000000007105 ) ) ;
#22720=ORIENTED_EDGE ( 'NONE', *, *, #3779, .F. ) ;
#22723=EDGE_LOOP ( 'NONE', ( #13720, #28808, #25595, #23191 ) ) ;
#22724=ORIENTED_EDGE ( 'NONE', *, *, #12067, .F. ) ;
#22725=CARTESIAN_POINT ( 'NONE',  ( 157.2187500000000284, 2.485281374238555774, -6.000000000000005329 ) ) ;
#22730=CARTESIAN_POINT ( 'NONE',  ( 151.3199251345948255, -2.278174593051950136, -5.500000000000074607 ) ) ;
#22734=CARTESIAN_POINT ( 'NONE',  ( 159.6227035152770668, -12.16574911538731740, 3.793091317978431576 ) ) ;
#22739=CARTESIAN_POINT ( 'NONE',  ( 159.5364582854214746, -11.09853219182770090, -4.564322074144446795 ) ) ;
#22740=DIRECTION ( 'NONE',  ( -0.000000000000000000, -0.000000000000000000, -1.000000000000000000 ) ) ;
#22749=FACE_OUTER_BOUND ( 'NONE', #717, .T. ) ;
#22756=CARTESIAN_POINT ( 'NONE',  ( 140.2648502691896795, 3.535533905932725318, 3.535533905932752852 ) ) ;
#22757=EDGE_CURVE ( 'NONE', #17555, #27766, #18492, .T. ) ;
#22758=VERTEX_POINT ( 'NONE', #4480 ) ;
#22765=CARTESIAN_POINT ( 'NONE',  ( 139.2187500000000000, 2.485281374238555774, -6.000000000000005329 ) ) ;
#22767=EDGE_LOOP ( 'NONE', ( #7184, #6949 ) ) ;
#22774=CARTESIAN_POINT ( 'NONE',  ( 135.1084928141376054, -8.790281914029968391, -8.000000000000007105 ) ) ;
#22776=CARTESIAN_POINT ( 'NONE',  ( 149.6101497308104058, 3.535533905932725318, 3.535533905932725318 ) ) ;
#22779=LINE ( 'NONE', #1720, #7485 ) ;
#22783=CARTESIAN_POINT ( 'NONE',  ( 137.6324251345948255, -5.500000000000012434, -2.278174593052012309 ) ) ;
#22790=LINE ( 'NONE', #25217, #1739 ) ;
#22795=CARTESIAN_POINT ( 'NONE',  ( 144.1875000000000284, 4.242640687119269671, 4.242640687119298093 ) ) ;
#22799=CARTESIAN_POINT ( 'NONE',  ( 136.0312500000000000, -2.485281374238555774, -6.000000000000005329 ) ) ;
#22817=FACE_OUTER_BOUND ( 'NONE', #6775, .T. ) ;
#22820=EDGE_CURVE ( 'NONE', #11247, #6328, #19534, .T. ) ;
#22821=CARTESIAN_POINT ( 'NONE',  ( 148.8898502691896510, 3.535533905932725318, -3.535533905932725318 ) ) ;
#22826=AXIS2_PLACEMENT_3D ( 'NONE', #13997, #6725, #29909 ) ;
#22830=VERTEX_POINT ( 'NONE', #5221 ) ;
#22831=CARTESIAN_POINT ( 'NONE',  ( 155.7187500000000568, 2.485281374238555774, -6.000000000000005329 ) ) ;
#22835=EDGE_LOOP ( 'NONE', ( #5041, #24776, #3611, #20489 ) ) ;
#22837=ORIENTED_EDGE ( 'NONE', *, *, #3467, .F. ) ;
#22838=ORIENTED_EDGE ( 'NONE', *, *, #14124, .T. ) ;
#22840=CARTESIAN_POINT ( 'NONE',  ( 116.0000000000000142, 0.000000000000000000, -5.500000000000000000 ) ) ;
#22844=DIRECTION ( 'NONE',  ( -1.000000000000000000, -0.000000000000000000, -0.000000000000000000 ) ) ;
#22851=CARTESIAN_POINT ( 'NONE',  ( 159.0000000000000284, -11.31370849898477537, 4.000000000000003553 ) ) ;
#22861=CARTESIAN_POINT ( 'NONE',  ( 159.6711002691896510, 4.999999999999989342, 2.071067811865468400 ) ) ;
#22862=CARTESIAN_POINT ( 'NONE',  ( -0.05509383827833347347, -14.57570334281945001, 8.269883983291466123 ) ) ;
#22863=ORIENTED_EDGE ( 'NONE', *, *, #601, .T. ) ;
#22868=ORIENTED_EDGE ( 'NONE', *, *, #20256, .F. ) ;
#22869=PRESENTATION_STYLE_ASSIGNMENT (( #25450 ) ) ;
#22870=VECTOR ( 'NONE', #22172, 1000.000000000000000 ) ;
#22875=CARTESIAN_POINT ( 'NONE',  ( 157.3125000000000284, 4.242640687119298093, -4.242640687119298093 ) ) ;
#22879=ORIENTED_EDGE ( 'NONE', *, *, #5279, .F. ) ;
#22883=CARTESIAN_POINT ( 'NONE',  ( 160.9483822453071014, -11.55409466406504748, 3.248948683749017796 ) ) ;
#22884=( NAMED_UNIT ( * ) SI_UNIT ( $, .STERADIAN. ) SOLID_ANGLE_UNIT ( ) );
#22888=CARTESIAN_POINT ( 'NONE',  ( 140.0769230769231228, -11.53846153846155254, 4.615384615384604317 ) ) ;
#22889=AXIS2_PLACEMENT_3D ( 'NONE', #20045, #24328, #20349 ) ;
#22890=EDGE_CURVE ( 'NONE', #25655, #12427, #15074, .T. ) ;
#22891=CARTESIAN_POINT ( 'NONE',  ( 159.7995982923682732, -12.30064632830203664, -3.603981859628974771 ) ) ;
#22893=FACE_OUTER_BOUND ( 'NONE', #23343, .T. ) ;
#22896=DIRECTION ( 'NONE',  ( 6.938893903907221278E-15, -1.000000000000000000, 0.000000000000000000 ) ) ;
#22900=( GEOMETRIC_REPRESENTATION_CONTEXT ( 3 ) GLOBAL_UNCERTAINTY_ASSIGNED_CONTEXT ( ( #14288 ) ) GLOBAL_UNIT_ASSIGNED_CONTEXT ( ( #29826, #4483, #16061 ) ) REPRESENTATION_CONTEXT ( 'NONE', 'WORKASPACE' ) );
#22904=CYLINDRICAL_SURFACE ( 'NONE', #15320, 0.5000000000000004441 ) ;
#22905=CARTESIAN_POINT ( 'NONE',  ( 140.4523502691896510, 0.000000000000000000, 5.000000000000004441 ) ) ;
#22906=EDGE_LOOP ( 'NONE', ( #8388, #4868, #26108, #10136 ) ) ;
#22915=ORIENTED_EDGE ( 'NONE', *, *, #20112, .F. ) ;
#22918=CARTESIAN_POINT ( 'NONE',  ( 143.5312500000000284, -2.485281374238555774, -6.000000000000005329 ) ) ;
#22920=SURFACE_STYLE_USAGE ( .BOTH. , #973 ) ;
#22922=DIRECTION ( 'NONE',  ( 0.000000000000000000, 0.000000000000000000, 1.000000000000000000 ) ) ;
#22924=CARTESIAN_POINT ( 'NONE',  ( 136.5863248654052313, 0.000000000000000000, 5.500000000000005329 ) ) ;
#22925=CIRCLE ( 'NONE', #27805, 0.5000000000000004441 ) ;
#22929=CARTESIAN_POINT ( 'NONE',  ( 135.0583403565074150, -7.808325495656168513, -8.343593232213100563 ) ) ;
#22930=CARTESIAN_POINT ( 'NONE',  ( 145.1101497308104058, 3.535533905932725318, 3.535533905932725318 ) ) ;
#22934=CARTESIAN_POINT ( 'NONE',  ( -15.49999999999999289, -24.99999999999999289, 7.500000000000007105 ) ) ;
#22945=DIRECTION ( 'NONE',  ( 0.000000000000000000, 0.000000000000000000, 1.000000000000000000 ) ) ;
#22948=CARTESIAN_POINT ( 'NONE',  ( 147.6562500000000568, -6.000000000000005329, 2.485281374238556218 ) ) ;
#22949=CARTESIAN_POINT ( 'NONE',  ( 159.9005546240083788, -12.40839718913323431, -3.439547090519799788 ) ) ;
#22951=MECHANICAL_DESIGN_GEOMETRIC_PRESENTATION_REPRESENTATION('',(#27832),#24897);
#22952=( BOUNDED_SURFACE ( )  B_SPLINE_SURFACE ( 3, 2, ( 
 ( #25805, #12317, #28682 ),
 ( #23520, #28089, #7505 ),
 ( #2602, #11876, #16477 ),
 ( #21212, #17064, #9984 ),
 ( #26393, #19360, #16919 ),
 ( #21358, #28243, #7217 ) ),
 .UNSPECIFIED., .F., .F., .F. ) 
 B_SPLINE_SURFACE_WITH_KNOTS ( ( 4, 2, 4 ),
 ( 3, 3 ),
 ( 0.000000000000000000, 0.001011980645342317126, 0.002023961290684634252 ),
 ( 0.000000000000000000, 1.000000000000000000 ),
 .UNSPECIFIED. ) 
 GEOMETRIC_REPRESENTATION_ITEM ( )  RATIONAL_B_SPLINE_SURFACE ( (
 ( 1.000000000000000000, 0.8593225670956829987, 1.000000000000000000),
 ( 1.000000000000000000, 0.8348814976564934431, 1.000000000000000000),
 ( 1.000000000000000000, 0.8097437468337547184, 1.000000000000000000),
 ( 1.000000000000000000, 0.7587734595484167954, 1.000000000000000000),
 ( 1.000000000000000000, 0.7329355451685689582, 1.000000000000000000),
 ( 1.000000000000000000, 0.7071067811865475727, 1.000000000000000000) ) ) 
 REPRESENTATION_ITEM ( '' )  SURFACE ( )  );
#22953=CARTESIAN_POINT ( 'NONE',  ( 140.8125000000000284, 4.242640687119298093, -4.242640687119298093 ) ) ;
#22956=ADVANCED_FACE ( 'NONE', ( #3517 ), #5523, .T. ) ;
#22958=VERTEX_POINT ( 'NONE', #24725 ) ;
#22965=CARTESIAN_POINT ( 'NONE',  ( 140.1363996827915059, -11.13639968279144732, -4.472640761300552548 ) ) ;
#22968=VECTOR ( 'NONE', #26303, 1000.000000000000000 ) ;
#22969=VECTOR ( 'NONE', #5908, 1000.000000000000000 ) ;
#22971=TOROIDAL_SURFACE ( 'NONE', #9732, 11.00000000000000355, 1.000000000000000000 ) ;
#22977=DIRECTION ( 'NONE',  ( -1.040834085586083310E-14, -1.000000000000000000, 0.000000000000000000 ) ) ;
#22980=CARTESIAN_POINT ( 'NONE',  ( 148.9836002691896795, 4.999999999999989342, -2.071067811865468400 ) ) ;
#22987=DIRECTION ( 'NONE',  ( -1.000000000000000000, 0.000000000000000000, 0.000000000000000000 ) ) ;
#22989=CARTESIAN_POINT ( 'NONE',  ( 153.4687500000000853, -2.485281374238585972, 6.000000000000005329 ) ) ;
#22990=CARTESIAN_POINT ( 'NONE',  ( -0.5000000000000004441, -10.00000000000000888, -5.000000000000004441 ) ) ;
#22994=ORIENTED_EDGE ( 'NONE', *, *, #1648, .F. ) ;
#22999=ADVANCED_FACE ( 'NONE', ( #13101 ), #11675, .T. ) ;
#23002=B_SPLINE_CURVE_WITH_KNOTS ( 'NONE', 3,
 ( #20771, #8307, #25190, #24752, #13274, #15891, #29655, #4000, #13419, #27040, #1858, #27347 ),
 .UNSPECIFIED., .F., .F.,
 ( 4, 2, 2, 2, 2, 4 ),
 ( 0.000000000000000000, 0.0002134524463634672269, 0.0004269048927269344538, 0.0008538097854538677150, 0.001280714678180800868, 0.001707619570907734346 ),
 .UNSPECIFIED. ) ;
#23006=( NAMED_UNIT ( * ) SI_UNIT ( $, .STERADIAN. ) SOLID_ANGLE_UNIT ( ) );
#23008=CARTESIAN_POINT ( 'NONE',  ( 139.6491219074057710, -8.798545334315207356, 8.159999999999998366 ) ) ;
#23012=PRESENTATION_STYLE_ASSIGNMENT (( #23478 ) ) ;
#23015=CARTESIAN_POINT ( 'NONE',  ( 0.2066684337268677174, -15.46624955645880561, 8.188921300829465011 ) ) ;
#23021=CARTESIAN_POINT ( 'NONE',  ( 157.6949251345948539, 5.500000000000012434, -2.278174593052012309 ) ) ;
#23025=EDGE_CURVE ( 'NONE', #12881, #12934, #3686, .T. ) ;
#23030=ORIENTED_EDGE ( 'NONE', *, *, #6659, .F. ) ;
#23031=CARTESIAN_POINT ( 'NONE',  ( 148.5000000000000284, 6.000000000000005329, 0.000000000000000000 ) ) ;
#23035=ADVANCED_FACE ( 'NONE', ( #1833 ), #23049, .T. ) ;
#23038=ORIENTED_EDGE ( 'NONE', *, *, #24396, .F. ) ;
#23042=( NAMED_UNIT ( * ) PLANE_ANGLE_UNIT ( ) SI_UNIT ( $, .RADIAN. ) );
#23045=CARTESIAN_POINT ( 'NONE',  ( 0.7669223171414829565, -15.58766199952930620, -7.954545454545462135 ) ) ;
#23049=CYLINDRICAL_SURFACE ( 'NONE', #13429, 0.5000000000000004441 ) ;
#23059=DIRECTION ( 'NONE',  ( -1.000000000000000000, -1.067522139062651904E-16, 0.000000000000000000 ) ) ;
#23062=CIRCLE ( 'NONE', #4897, 6.499999999999977796 ) ;
#23063=LINE ( 'NONE', #7066, #13631 ) ;
#23064=DIRECTION ( 'NONE',  ( 0.000000000000000000, 0.000000000000000000, -1.000000000000000000 ) ) ;
#23065=CARTESIAN_POINT ( 'NONE',  ( 136.5148502691896510, -3.535533905932725318, -3.535533905932725318 ) ) ;
#23069=CARTESIAN_POINT ( 'NONE',  ( 151.1175748654052313, 5.500000000000012434, -2.278174593052012309 ) ) ;
#23074=EDGE_CURVE ( 'NONE', #23261, #7272, #11237, .T. ) ;
#23078=CARTESIAN_POINT ( 'NONE',  ( 138.5699251345948255, 2.278174593052352925, 5.499999999999671374 ) ) ;
#23079=CARTESIAN_POINT ( 'NONE',  ( 137.7187500000000284, 2.485281374238555774, -6.000000000000005329 ) ) ;
#23081=FACE_OUTER_BOUND ( 'NONE', #1238, .T. ) ;
#23085=DIRECTION ( 'NONE',  ( 0.000000000000000000, 0.000000000000000000, -1.000000000000000000 ) ) ;
#23088=CARTESIAN_POINT ( 'NONE',  ( 135.2991173618539165, -8.337648098108042305, -8.244751738008236686 ) ) ;
#23089=CARTESIAN_POINT ( 'NONE',  ( 145.0163997308104058, 4.999999999999989342, 2.071067811865468400 ) ) ;
#23092=CARTESIAN_POINT ( 'NONE',  ( 144.0863248654052313, 0.000000000000000000, 5.500000000000005329 ) ) ;
#23099=CARTESIAN_POINT ( 'NONE',  ( 116.0000000000000142, 0.000000000000000000, 0.000000000000000000 ) ) ;
#23102=CARTESIAN_POINT ( 'NONE',  ( 162.0000000000000284, 0.000000000000000000, 0.000000000000000000 ) ) ;
#23107=CARTESIAN_POINT ( 'NONE',  ( 140.8125000000000284, 4.242640687119298093, -4.242640687119298093 ) ) ;
#23108=STYLED_ITEM ( 'NONE', ( #20579 ), #27917 ) ;
#23110=ADVANCED_FACE ( 'NONE', ( #22893 ), #27923, .F. ) ;
#23111=CARTESIAN_POINT ( 'NONE',  ( 139.8750000000000284, 0.000000000000000000, 6.000000000000005329 ) ) ;
#23114=TOROIDAL_SURFACE ( 'NONE', #26514, 16.50000000000000355, 1.000000000000000000 ) ;
#23117=VERTEX_POINT ( 'NONE', #13708 ) ;
#23120=CARTESIAN_POINT ( 'NONE',  ( 155.1636751345948255, 0.000000000000000000, 5.500000000000005329 ) ) ;
#23122=DIRECTION ( 'NONE',  ( 1.000000000000000000, 0.000000000000000000, -0.000000000000000000 ) ) ;
#23123=AXIS2_PLACEMENT_3D ( 'NONE', #15907, #22475, #12982 ) ;
#23124=CARTESIAN_POINT ( 'NONE',  ( 136.0000000000000284, -9.165151389911669000, 8.500000000000007105 ) ) ;
#23130=COLOUR_RGB ( '', 0.66274510, 0.83137255, 0.94901961) ;
#23132=CARTESIAN_POINT ( 'NONE',  ( 155.1488248654052029, -3.889087296526011706, -3.889087296526011706 ) ) ;
#23138=CARTESIAN_POINT ( 'NONE',  ( 160.7738248654052029, -3.889087296526011706, 3.889087296526011706 ) ) ;
#23139=CARTESIAN_POINT ( 'NONE',  ( 138.6636751345948255, 0.000000000000000000, 5.500000000000005329 ) ) ;
#23140=MECHANICAL_DESIGN_GEOMETRIC_PRESENTATION_REPRESENTATION('',(#15297),#13848);
#23141=CARTESIAN_POINT ( 'NONE',  ( 157.1250000000000284, 0.000000000000000000, -6.000000000000005329 ) ) ;
#23146=FILL_AREA_STYLE ('',( #4374 ) ) ;
#23147=EDGE_CURVE ( 'NONE', #3410, #4566, #24973, .T. ) ;
#23149=CARTESIAN_POINT ( 'NONE',  ( 158.0625000000000284, -4.242640687119298093, 4.242640687119298093 ) ) ;
#23152=CIRCLE ( 'NONE', #9897, 14.49999999999999822 ) ;
#23154=ORIENTED_EDGE ( 'NONE', *, *, #9843, .F. ) ;
#23156=CIRCLE ( 'NONE', #3484, 1.000000000000000000 ) ;
#23160=CARTESIAN_POINT ( 'NONE',  ( -0.4142135623730956451, -9.292893218813460976, -4.000000000000004441 ) ) ;
#23167=CARTESIAN_POINT ( 'NONE',  ( -0.5000000000000004441, -10.50000000000000888, 7.500000000000007105 ) ) ;
#23176=CARTESIAN_POINT ( 'NONE',  ( 0.1950436299885377478, -15.42103240523036334, 8.274747089234001152 ) ) ;
#23183=DIRECTION ( 'NONE',  ( 0.000000000000000000, 1.000000000000000000, 0.000000000000000000 ) ) ;
#23188=ORIENTED_EDGE ( 'NONE', *, *, #7096, .T. ) ;
#23189=DIRECTION ( 'NONE',  ( 0.3589790793088772358, -0.3589790793088664111, -0.8615497903412833169 ) ) ;
#23190=CARTESIAN_POINT ( 'NONE',  ( 151.1250000000000284, 0.000000000000000000, -6.000000000000005329 ) ) ;
#23191=ORIENTED_EDGE ( 'NONE', *, *, #1289, .F. ) ;
#23195=ORIENTED_EDGE ( 'NONE', *, *, #6322, .F. ) ;
#23198=CARTESIAN_POINT ( 'NONE',  ( 161.0000000000000284, -11.67610212985248275, 2.769230769230770939 ) ) ;
#23199=( NAMED_UNIT ( * ) PLANE_ANGLE_UNIT ( ) SI_UNIT ( $, .RADIAN. ) );
#23200=ORIENTED_EDGE ( 'NONE', *, *, #14847, .T. ) ;
#23203=CARTESIAN_POINT ( 'NONE',  ( 152.9136751345948539, 0.000000000000000000, -5.500000000000005329 ) ) ;
#23210=CARTESIAN_POINT ( 'NONE',  ( -0.1262135825162392921, -9.436893208741910399, -4.496381089953947807 ) ) ;
#23212=DIRECTION ( 'NONE',  ( -0.000000000000000000, -1.000000000000000000, -0.000000000000000000 ) ) ;
#23215=CARTESIAN_POINT ( 'NONE',  ( 135.0000000000000284, -7.637914190097514933, -8.088422893840236938 ) ) ;
#23219=DIRECTION ( 'NONE',  ( -0.000000000000000000, -0.000000000000000000, -1.000000000000000000 ) ) ;
#23222=ORIENTED_EDGE ( 'NONE', *, *, #28211, .T. ) ;
#23224=CARTESIAN_POINT ( 'NONE',  ( 151.3988248654052313, 3.889087296526011706, 3.889087296526011706 ) ) ;
#23233=DIRECTION ( 'NONE',  ( -1.000000000000000000, 0.000000000000000000, 0.000000000000000000 ) ) ;
#23234=CARTESIAN_POINT ( 'NONE',  ( 137.6250000000000284, 0.000000000000000000, -6.000000000000005329 ) ) ;
#23237=CARTESIAN_POINT ( 'NONE',  ( -4.999999999999886313, -10.00000000000000888, 5.000000000000004441 ) ) ;
#23242=VECTOR ( 'NONE', #28644, 1000.000000000000000 ) ;
#23243=CARTESIAN_POINT ( 'NONE',  ( 141.1726497308104342, -5.000000000000004441, 0.000000000000000000 ) ) ;
#23246=CARTESIAN_POINT ( 'NONE',  ( 135.0000000000000284, -11.07692307692306777, -4.615384615384604317 ) ) ;
#23247=TOROIDAL_SURFACE ( 'NONE', #9989, 16.50000000000000355, 1.000000000000000000 ) ;
#23255=FACE_OUTER_BOUND ( 'NONE', #29457, .T. ) ;
#23257=( NAMED_UNIT ( * ) SI_UNIT ( $, .STERADIAN. ) SOLID_ANGLE_UNIT ( ) );
#23260=DIRECTION ( 'NONE',  ( 0.000000000000000000, 0.000000000000000000, -1.000000000000000000 ) ) ;
#23261=VERTEX_POINT ( 'NONE', #18256 ) ;
#23263=CARTESIAN_POINT ( 'NONE',  ( 137.7187500000000284, 2.485281374238556218, -6.000000000000005329 ) ) ;
#23265=CARTESIAN_POINT ( 'NONE',  ( 138.7425748654052313, -2.278174593052352925, -5.499999999999671374 ) ) ;
#23266=CARTESIAN_POINT ( 'NONE',  ( 133.4062500000000568, 6.000000000000005329, -2.485281374238555774 ) ) ;
#23268=AXIS2_PLACEMENT_3D ( 'NONE', #19542, #12055, #185 ) ;
#23270=ORIENTED_EDGE ( 'NONE', *, *, #30014, .T. ) ;
#23273=( BOUNDED_CURVE ( )  B_SPLINE_CURVE ( 2, ( #9969, #12596, #19347, #7640, #24081, #12449, #21792, #17648, #8236 ),
 .UNSPECIFIED., .F., .F. ) 
 B_SPLINE_CURVE_WITH_KNOTS ( ( 3, 2, 2, 2, 3 ),
 ( 0.6625000000000010880, 0.6687500000000008438, 0.6750000000000007105, 0.6812500000000004663, 0.6875000000000002220 ),
 .UNSPECIFIED. ) 
 CURVE ( )  GEOMETRIC_REPRESENTATION_ITEM ( )  RATIONAL_B_SPLINE_CURVE ( ( 0.9999999999999864553, 0.9238795325113002832, 1.000000000000000000, 0.9238795325112867385, 1.000000000000000000, 0.9238795325112867385, 1.000000000000000000, 0.9238795325112840739, 1.000000000000002665 ) ) 
 REPRESENTATION_ITEM ( '' )  );
#23278=CARTESIAN_POINT ( 'NONE',  ( -4.999999999999990230, -55.00000000000002132, -8.000000000000007105 ) ) ;
#23285=EDGE_CURVE ( 'NONE', #10891, #8542, #21070, .T. ) ;
#23287=CARTESIAN_POINT ( 'NONE',  ( 140.0676280679787169, -9.491795069345080549, -7.344273253287639136 ) ) ;
#23292=DIRECTION ( 'NONE',  ( -0.000000000000000000, -0.000000000000000000, -1.000000000000000000 ) ) ;
#23295=DIRECTION ( 'NONE',  ( -1.000000000000000000, 3.469446951953694061E-16, 0.000000000000000000 ) ) ;
#23296=CARTESIAN_POINT ( 'NONE',  ( 159.2812500000000284, 2.485281374238585972, 6.000000000000005329 ) ) ;
#23299=CARTESIAN_POINT ( 'NONE',  ( 138.7574251345947971, -2.278174593051671692, 5.500000000000352607 ) ) ;
#23300=DIRECTION ( 'NONE',  ( 0.000000000000000000, 0.000000000000000000, 1.000000000000000000 ) ) ;
#23304=CARTESIAN_POINT ( 'NONE',  ( 158.2500000000000284, -6.000000000000005329, 0.000000000000000000 ) ) ;
#23305=CYLINDRICAL_SURFACE ( 'NONE', #24379, 0.5000000000000004441 ) ;
#23314=ORIENTED_EDGE ( 'NONE', *, *, #12182, .F. ) ;
#23315=CARTESIAN_POINT ( 'NONE',  ( 1.000000000000000888, 0.000000000000000000, 0.000000000000000000 ) ) ;
#23326=CARTESIAN_POINT ( 'NONE',  ( 146.3363248654052029, 0.000000000000000000, -5.500000000000005329 ) ) ;
#23328=DIRECTION ( 'NONE',  ( -0.000000000000000000, 0.2307692307692307543, -0.9730085108210398959 ) ) ;
#23329=SURFACE_STYLE_USAGE ( .BOTH. , #4405 ) ;
#23339=CARTESIAN_POINT ( 'NONE',  ( 0.000000000000000000, -15.50000000000001421, -8.000000000000007105 ) ) ;
#23343=EDGE_LOOP ( 'NONE', ( #1622, #12321, #10303, #1771 ) ) ;
#23346=CARTESIAN_POINT ( 'NONE',  ( 150.7500000000000284, -6.000000000000005329, 0.000000000000000000 ) ) ;
#23348=TOROIDAL_SURFACE ( 'NONE', #6153, 28.99999999999999645, 1.000000000000000000 ) ;
#23349=EDGE_CURVE ( 'NONE', #18727, #5920, #21455, .T. ) ;
#23354=CARTESIAN_POINT ( 'NONE',  ( -0.5000000000000004441, -9.500000000000008882, 7.500000000000007105 ) ) ;
#23358=CARTESIAN_POINT ( 'NONE',  ( 153.6636751345948255, 0.000000000000000000, 5.500000000000005329 ) ) ;
#23364=CARTESIAN_POINT ( 'NONE',  ( 116.0000000000000142, 0.000000000000000000, 0.000000000000000000 ) ) ;
#23365=CARTESIAN_POINT ( 'NONE',  ( 160.8919244128742605, -11.51465293479089524, -3.380337924145041750 ) ) ;
#23367=CARTESIAN_POINT ( 'NONE',  ( -1.000000000000000888, 9.000000000000007105, 5.000000000000004441 ) ) ;
#23378=FILL_AREA_STYLE ('',( #14040 ) ) ;
#23383=CARTESIAN_POINT ( 'NONE',  ( 133.2187500000000568, 2.485281374238555774, -6.000000000000005329 ) ) ;
#23387=DIRECTION ( 'NONE',  ( -1.000000000000000000, 0.000000000000000000, 0.000000000000000000 ) ) ;
#23390=EDGE_CURVE ( 'NONE', #9852, #7029, #6233, .T. ) ;
#23393=CARTESIAN_POINT ( 'NONE',  ( 146.5163997308104058, 4.999999999999989342, 2.071067811865468400 ) ) ;
#23398=CARTESIAN_POINT ( 'NONE',  ( 156.2886751345948255, 5.500000000000005329, 0.000000000000000000 ) ) ;
#23402=CARTESIAN_POINT ( 'NONE',  ( -4.999999999999886313, -15.00000000000001421, 7.500000000000007105 ) ) ;
#23404=COLOUR_RGB ( '', 0.31764706, 0.68627451, 0.89019608) ;
#23408=( BOUNDED_CURVE ( )  B_SPLINE_CURVE ( 2, ( #3250, #17131, #507, #9903, #14821, #950, #24164, #3106, #24303 ),
 .UNSPECIFIED., .F., .T. ) 
 B_SPLINE_CURVE_WITH_KNOTS ( ( 3, 2, 2, 2, 3 ),
 ( 0.2374999999999997391, 0.2437499999999995226, 0.2499999999999992784, 0.2562499999999990896, 0.2624999999999988454 ),
 .UNSPECIFIED. ) 
 CURVE ( )  GEOMETRIC_REPRESENTATION_ITEM ( )  RATIONAL_B_SPLINE_CURVE ( ( 1.000000000000003775, 0.9238795325112830747, 1.000000000000000000, 0.9238795325112867385, 1.000000000000000000, 0.9238795325112867385, 1.000000000000000000, 0.9238795325113002832, 0.9999999999999864553 ) ) 
 REPRESENTATION_ITEM ( '' )  );
#23411=CARTESIAN_POINT ( 'NONE',  ( 140.2500000000000284, -6.000000000000005329, 0.000000000000000000 ) ) ;
#23415=CARTESIAN_POINT ( 'NONE',  ( 132.7500000000000284, -6.000000000000005329, 0.000000000000000000 ) ) ;
#23416=FACE_OUTER_BOUND ( 'NONE', #8078, .T. ) ;
#23424=FACE_OUTER_BOUND ( 'NONE', #21006, .T. ) ;
#23443=DIRECTION ( 'NONE',  ( 1.000000000000000000, -0.000000000000000000, -0.000000000000000000 ) ) ;
#23445=CARTESIAN_POINT ( 'NONE',  ( 156.2812500000000284, 2.485281374238585972, 6.000000000000005329 ) ) ;
#23450=DIRECTION ( 'NONE',  ( 0.000000000000000000, 0.000000000000000000, -1.000000000000000000 ) ) ;
#23452=CARTESIAN_POINT ( 'NONE',  ( 150.1875000000000284, 4.242640687119269671, 4.242640687119298093 ) ) ;
#23454=VECTOR ( 'NONE', #18986, 1000.000000000000000 ) ;
#23458=EDGE_LOOP ( 'NONE', ( #25428, #2874, #327, #25150 ) ) ;
#23460=ADVANCED_FACE ( 'NONE', ( #22199 ), #15629, .F. ) ;
#23464=CIRCLE ( 'NONE', #9706, 12.00000000000000178 ) ;
#23467=CARTESIAN_POINT ( 'NONE',  ( 157.7663997308104626, -4.999999999999989342, -2.071067811865468400 ) ) ;
#23470=CARTESIAN_POINT ( 'NONE',  ( 135.7516005668334742, -9.165151352139671914, 8.000000000000007105 ) ) ;
#23478=SURFACE_STYLE_USAGE ( .BOTH. , #9026 ) ;
#23482=CARTESIAN_POINT ( 'NONE',  ( 135.0000000000000284, -7.344328791152317848, 8.346722065162424542 ) ) ;
#23483=ORIENTED_EDGE ( 'NONE', *, *, #1400, .F. ) ;
#23488=ORIENTED_EDGE ( 'NONE', *, *, #10064, .T. ) ;
#23493=CARTESIAN_POINT ( 'NONE',  ( 150.0000000000000284, 6.000000000000005329, 0.000000000000000000 ) ) ;
#23494=VERTEX_POINT ( 'NONE', #13176 ) ;
#23500=CARTESIAN_POINT ( 'NONE',  ( -4.999999999999990230, -55.00000000000002132, 7.500000000000007105 ) ) ;
#23504=CARTESIAN_POINT ( 'NONE',  ( 0.7522227795206197776, -15.54366488976627636, -8.040203489970597417 ) ) ;
#23505=COLOUR_RGB ( '', 0.08235294, 0.09019608, 0.10196078) ;
#23511=CARTESIAN_POINT ( 'NONE',  ( -0.7382520721438933231, -9.130873963928037185, -4.026027341348664912 ) ) ;
#23515=CARTESIAN_POINT ( 'NONE',  ( 134.9999999999992895, -7.177887245073663713, -8.449849189508016778 ) ) ;
#23519=EDGE_CURVE ( 'NONE', #30356, #11342, #22031, .T. ) ;
#23520=CARTESIAN_POINT ( 'NONE',  ( -0.04607149862261590567, -15.28219869613047521, 7.206732114352344176 ) ) ;
#23521=DIRECTION ( 'NONE',  ( -1.000000000000000000, -1.067522139062651411E-16, 0.000000000000000000 ) ) ;
#23525=FACE_OUTER_BOUND ( 'NONE', #20399, .T. ) ;
#23526=EDGE_CURVE ( 'NONE', #25268, #23117, #28258, .T. ) ;
#23528=ORIENTED_EDGE ( 'NONE', *, *, #9149, .T. ) ;
#23530=CARTESIAN_POINT ( 'NONE',  ( -9.999999999999793943, 10.00000000000000888, 3.000000000000002665 ) ) ;
#23531=CARTESIAN_POINT ( 'NONE',  ( 138.6562500000000568, -6.000000000000005329, 2.485281374238555774 ) ) ;
#23532=ORIENTED_EDGE ( 'NONE', *, *, #26434, .T. ) ;
#23536=PRESENTATION_STYLE_ASSIGNMENT (( #18631 ) ) ;
#23540=CARTESIAN_POINT ( 'NONE',  ( 143.8913997308104058, -2.071067811865468400, 4.999999999999989342 ) ) ;
#23542=DIRECTION ( 'NONE',  ( -0.000000000000000000, -0.000000000000000000, 1.000000000000000000 ) ) ;
#23547=CIRCLE ( 'NONE', #24971, 1.000000000000000888 ) ;
#23549=LINE ( 'NONE', #7252, #1395 ) ;
#23550=CARTESIAN_POINT ( 'NONE',  ( 140.9136751345948539, 0.000000000000000000, -5.500000000000005329 ) ) ;
#23556=CARTESIAN_POINT ( 'NONE',  ( 141.1875000000000284, 4.242640687119269671, 4.242640687119298093 ) ) ;
#23559=EDGE_CURVE ( 'NONE', #4026, #10268, #25820, .T. ) ;
#23560=CARTESIAN_POINT ( 'NONE',  ( 135.2812500000000284, 2.485281374238585972, 6.000000000000005329 ) ) ;
#23565=ORIENTED_EDGE ( 'NONE', *, *, #20069, .T. ) ;
#23570=LINE ( 'NONE', #16827, #1433 ) ;
#23576=( BOUNDED_CURVE ( )  B_SPLINE_CURVE ( 2, ( #11246, #20756, #9067, #14030, #13719, #151, #7061, #25325, #16474 ),
 .UNSPECIFIED., .F., .T. ) 
 B_SPLINE_CURVE_WITH_KNOTS ( ( 3, 2, 2, 2, 3 ),
 ( 0.2374999999999997391, 0.2437499999999999944, 0.2500000000000002220, 0.2562500000000004774, 0.2625000000000007327 ),
 .UNSPECIFIED. ) 
 CURVE ( )  GEOMETRIC_REPRESENTATION_ITEM ( )  RATIONAL_B_SPLINE_CURVE ( ( 1.000000000000003109, 0.9238795325112837409, 1.000000000000000000, 0.9238795325112867385, 1.000000000000000000, 0.9238795325112867385, 1.000000000000000000, 0.9238795325112779677, 1.000000000000008882 ) ) 
 REPRESENTATION_ITEM ( '' )  );
#23581=ADVANCED_FACE ( 'NONE', ( #27387 ), #8358, .T. ) ;
#23585=CIRCLE ( 'NONE', #9350, 30.00000000000000000 ) ;
#23586=DIRECTION ( 'NONE',  ( 1.000000000000000000, 0.000000000000000000, 0.000000000000000000 ) ) ;
#23587=CARTESIAN_POINT ( 'NONE',  ( 143.1711002691896795, 4.999999999999989342, 2.071067811865468400 ) ) ;
#23589=CARTESIAN_POINT ( 'NONE',  ( 158.5312500000000284, -2.485281374238556218, -6.000000000000005329 ) ) ;
#23593=DIRECTION ( 'NONE',  ( -0.000000000000000000, -0.000000000000000000, -1.000000000000000000 ) ) ;
#23598=CARTESIAN_POINT ( 'NONE',  ( 148.8750000000000284, 0.000000000000000000, 6.000000000000005329 ) ) ;
#23599=DIRECTION ( 'NONE',  ( 1.000000000000000000, 9.251858538542971828E-16, 0.000000000000000000 ) ) ;
#23601=B_SPLINE_CURVE_WITH_KNOTS ( 'NONE', 3,
 ( #5397, #10493, #3236, #26885, #21855, #12815, #12973, #24438, #22308, #29349, #10647, #5845, #22158, #14948, #24148, #802 ),
 .UNSPECIFIED., .F., .F.,
 ( 4, 2, 2, 2, 2, 2, 2, 4 ),
 ( 0.000000000000000000, 0.0003858708990758222723, 0.0007717417981516445447, 0.001543483596303289089, 0.001929354495379140798, 0.002315225394454992723, 0.002701096293530844215, 0.003086967192606696140 ),
 .UNSPECIFIED. ) ;
#23602=CARTESIAN_POINT ( 'NONE',  ( 140.0769230769231228, -11.53846153846155254, 4.615384615384604317 ) ) ;
#23607=TOROIDAL_SURFACE ( 'NONE', #24065, 28.99999999999999645, 1.000000000000000000 ) ;
#23613=CARTESIAN_POINT ( 'NONE',  ( 156.7351497308104058, 3.535533905932725318, -3.535533905932725318 ) ) ;
#23615=VECTOR ( 'NONE', #18643, 1000.000000000000000 ) ;
#23622=CYLINDRICAL_SURFACE ( 'NONE', #1007, 1.000000000000000888 ) ;
#23627=CARTESIAN_POINT ( 'NONE',  ( 156.8586002691896510, 2.071067811865468400, 4.999999999999989342 ) ) ;
#23631=DIRECTION ( 'NONE',  ( -1.000000000000000000, 0.000000000000000000, 0.000000000000000000 ) ) ;
#23634=ORIENTED_EDGE ( 'NONE', *, *, #28272, .F. ) ;
#23638=CIRCLE ( 'NONE', #21680, 0.5000000000000004441 ) ;
#23639=EDGE_LOOP ( 'NONE', ( #20962, #20368, #10440, #27517 ) ) ;
#23642=CARTESIAN_POINT ( 'NONE',  ( 151.3125000000000568, 4.242640687119298093, -4.242640687119298093 ) ) ;
#23643=ORIENTED_EDGE ( 'NONE', *, *, #15265, .T. ) ;
#23647=ORIENTED_EDGE ( 'NONE', *, *, #12743, .F. ) ;
#23651=CARTESIAN_POINT ( 'NONE',  ( 133.3913997308104058, -2.071067811865468400, 4.999999999999989342 ) ) ;
#23654=CARTESIAN_POINT ( 'NONE',  ( 153.1011751345948824, 3.889087296526011706, -3.889087296526011706 ) ) ;
#23658=CARTESIAN_POINT ( 'NONE',  ( 136.0000000000000284, -9.165151389911669000, 8.000000000000007105 ) ) ;
#23659=CARTESIAN_POINT ( 'NONE',  ( 140.0000000000000284, -54.99999999999990763, 5.000000000000004441 ) ) ;
#23660=CARTESIAN_POINT ( 'NONE',  ( 160.5767363903362082, -11.34513390049722936, -3.911391104096503479 ) ) ;
#23661=EDGE_CURVE ( 'NONE', #452, #19300, #16387, .T. ) ;
#23664=AXIS2_PLACEMENT_3D ( 'NONE', #15231, #24564, #3515 ) ;
#23666=DIRECTION ( 'NONE',  ( 0.000000000000000000, 0.000000000000000000, 1.000000000000000000 ) ) ;
#23670=( LENGTH_UNIT ( ) NAMED_UNIT ( * ) SI_UNIT ( .MILLI., .METRE. ) );
#23672=DIRECTION ( 'NONE',  ( -0.000000000000000000, -0.000000000000000000, -1.000000000000000000 ) ) ;
#23673=CARTESIAN_POINT ( 'NONE',  ( 156.8511751345948539, -3.889087296526011706, 3.889087296526011706 ) ) ;
#23675=CARTESIAN_POINT ( 'NONE',  ( 140.8988248654052029, 3.889087296526011706, 3.889087296526011706 ) ) ;
#23676=ORIENTED_EDGE ( 'NONE', *, *, #21777, .F. ) ;
#23677=ORIENTED_EDGE ( 'NONE', *, *, #1013, .T. ) ;
#23679=CARTESIAN_POINT ( 'NONE',  ( 138.1875000000000284, 4.242640687119269671, 4.242640687119298093 ) ) ;
#23681=SURFACE_STYLE_USAGE ( .BOTH. , #14343 ) ;
#23689=CARTESIAN_POINT ( 'NONE',  ( 137.2351497308104058, 3.535533905932725318, -3.535533905932725318 ) ) ;
#23691=CARTESIAN_POINT ( 'NONE',  ( 139.5000000000000000, -24.99999999999999289, -8.000000000000007105 ) ) ;
#23700=VERTEX_POINT ( 'NONE', #18374 ) ;
#23706=CARTESIAN_POINT ( 'NONE',  ( 139.9687500000000284, -2.485281374238585972, 6.000000000000005329 ) ) ;
#23708=CARTESIAN_POINT ( 'NONE',  ( 138.0863248654052313, 0.000000000000000000, 5.500000000000005329 ) ) ;
#23709=CARTESIAN_POINT ( 'NONE',  ( 159.3601497308104058, -3.535533905932725318, -3.535533905932725318 ) ) ;
#23711=ORIENTED_EDGE ( 'NONE', *, *, #25651, .F. ) ;
#23712=DIRECTION ( 'NONE',  ( 1.000000000000000000, -0.000000000000000000, -0.000000000000000000 ) ) ;
#23713=EDGE_CURVE ( 'NONE', #12427, #12660, #17506, .T. ) ;
#23719=DIRECTION ( 'NONE',  ( 1.000000000000000000, -0.000000000000000000, 0.000000000000000000 ) ) ;
#23721=CARTESIAN_POINT ( 'NONE',  ( 140.6451377260904678, -11.29027545218211515, -4.288736938852192537 ) ) ;
#23722=CARTESIAN_POINT ( 'NONE',  ( 116.0000000000000142, 6.735557395310442023E-16, 5.500000000000000000 ) ) ;
#23724=EDGE_CURVE ( 'NONE', #30382, #25961, #21897, .T. ) ;
#23727=PLANE ( 'NONE',  #22665 ) ;
#23735=CARTESIAN_POINT ( 'NONE',  ( 145.4211002691896510, -4.999999999999989342, -2.071067811865468400 ) ) ;
#23738=CARTESIAN_POINT ( 'NONE',  ( 158.9062500000000284, 6.000000000000005329, -2.485281374238556218 ) ) ;
#23739=CARTESIAN_POINT ( 'NONE',  ( 135.0000000000000284, -6.982120021884474781, -8.500000000000007105 ) ) ;
#23741=SURFACE_STYLE_FILL_AREA ( #4676 ) ;
#23746=CARTESIAN_POINT ( 'NONE',  ( 150.2812500000000284, 2.485281374238585972, 6.000000000000005329 ) ) ;
#23750=ORIENTED_EDGE ( 'NONE', *, *, #16432, .F. ) ;
#23756=CARTESIAN_POINT ( 'NONE',  ( 156.2663997308104342, -4.999999999999989342, -2.071067811865468400 ) ) ;
#23757=CYLINDRICAL_SURFACE ( 'NONE', #25513, 9.999999999999980460 ) ;
#23759=FILL_AREA_STYLE ('',( #19596 ) ) ;
#23770=UNCERTAINTY_MEASURE_WITH_UNIT (LENGTH_MEASURE( 1.000000000000000082E-05 ), #25367, 'distance_accuracy_value', 'NONE');
#23780=CARTESIAN_POINT ( 'NONE',  ( 145.8750000000000284, 0.000000000000000000, 6.000000000000005329 ) ) ;
#23785=UNCERTAINTY_MEASURE_WITH_UNIT (LENGTH_MEASURE( 1.000000000000000082E-05 ), #23670, 'distance_accuracy_value', 'NONE');
#23789=CARTESIAN_POINT ( 'NONE',  ( 132.6413997308104342, 2.071067811865468400, -4.999999999999989342 ) ) ;
#23791=EDGE_CURVE ( 'NONE', #12642, #20769, #3307, .T. ) ;
#23796=DIRECTION ( 'NONE',  ( 1.000000000000000000, 0.000000000000000000, -0.000000000000000000 ) ) ;
#23799=DIRECTION ( 'NONE',  ( 0.000000000000000000, 0.000000000000000000, -1.000000000000000000 ) ) ;
#23801=CARTESIAN_POINT ( 'NONE',  ( 136.0000000000000284, -8.798545334315205579, 8.160000000000000142 ) ) ;
#23810=VERTEX_POINT ( 'NONE', #18218 ) ;
#23811=AXIS2_PLACEMENT_3D ( 'NONE', #27393, #11161, #22977 ) ;
#23820=CARTESIAN_POINT ( 'NONE',  ( 133.8898502691896510, 3.535533905932725318, -3.535533905932725318 ) ) ;
#23821=ADVANCED_FACE ( 'NONE', ( #18675 ), #16784, .F. ) ;
#23823=EDGE_CURVE ( 'NONE', #8771, #1653, #14665, .T. ) ;
#23824=ORIENTED_EDGE ( 'NONE', *, *, #22385, .T. ) ;
#23826=SURFACE_STYLE_USAGE ( .BOTH. , #12485 ) ;
#23834=CARTESIAN_POINT ( 'NONE',  ( 140.6101497308104058, 3.535533905932725318, 3.535533905932725318 ) ) ;
#23838=AXIS2_PLACEMENT_3D ( 'NONE', #25108, #3909, #24955 ) ;
#23839=DIRECTION ( 'NONE',  ( 1.387778780781444256E-14, 1.000000000000000000, -0.000000000000000000 ) ) ;
#23845=( BOUNDED_CURVE ( )  B_SPLINE_CURVE ( 2, ( #7848, #19991, #26723, #5687, #24586, #21995, #29343, #28883, #29183 ),
 .UNSPECIFIED., .F., .T. ) 
 B_SPLINE_CURVE_WITH_KNOTS ( ( 3, 2, 2, 2, 3 ),
 ( 0.7624999999999992895, 0.7687499999999996003, 0.7749999999999998002, 0.7812500000000000000, 0.7875000000000001998 ),
 .UNSPECIFIED. ) 
 CURVE ( )  GEOMETRIC_REPRESENTATION_ITEM ( )  RATIONAL_B_SPLINE_CURVE ( ( 1.000000000000008216, 0.9238795325112786339, 1.000000000000000000, 0.9238795325112867385, 1.000000000000000000, 0.9238795325112867385, 1.000000000000000000, 0.9238795325112840739, 1.000000000000002665 ) ) 
 REPRESENTATION_ITEM ( '' )  );
#23846=ORIENTED_EDGE ( 'NONE', *, *, #5928, .T. ) ;
#23849=VECTOR ( 'NONE', #1163, 1000.000000000000000 ) ;
#23851=CARTESIAN_POINT ( 'NONE',  ( 133.2187500000000568, 2.485281374238555774, -6.000000000000005329 ) ) ;
#23853=AXIS2_PLACEMENT_3D ( 'NONE', #20794, #30141, #2349 ) ;
#23856=ORIENTED_EDGE ( 'NONE', *, *, #23880, .T. ) ;
#23857=ORIENTED_EDGE ( 'NONE', *, *, #21685, .F. ) ;
#23861=DIRECTION ( 'NONE',  ( 0.000000000000000000, 0.000000000000000000, -1.000000000000000000 ) ) ;
#23868=DIRECTION ( 'NONE',  ( 1.000000000000000000, -3.469446951953694061E-16, 0.000000000000000000 ) ) ;
#23871=CARTESIAN_POINT ( 'NONE',  ( 15.00000000000000000, 0.000000000000000000, 0.000000000000000000 ) ) ;
#23874=CARTESIAN_POINT ( 'NONE',  ( 15.00000000000000000, 0.000000000000000000, 0.000000000000000000 ) ) ;
#23875=CARTESIAN_POINT ( 'NONE',  ( 143.5461002691896510, -2.071067811865468400, 4.999999999999989342 ) ) ;
#23876=CARTESIAN_POINT ( 'NONE',  ( 0.7669223171414760731, -15.58766199952932396, 7.954545454545463912 ) ) ;
#23877=CARTESIAN_POINT ( 'NONE',  ( 152.1562500000000284, -6.000000000000005329, 2.485281374238556218 ) ) ;
#23880=EDGE_CURVE ( 'NONE', #5354, #28619, #17913, .T. ) ;
#23881=AXIS2_PLACEMENT_3D ( 'NONE', #4025, #6494, #22945 ) ;
#23884=CARTESIAN_POINT ( 'NONE',  ( 151.9687500000000568, -2.485281374238585972, 6.000000000000005329 ) ) ;
#23886=TOROIDAL_SURFACE ( 'NONE', #14589, 2.000000000000000000, 1.000000000000000000 ) ;
#23887=UNCERTAINTY_MEASURE_WITH_UNIT (LENGTH_MEASURE( 1.000000000000000082E-05 ), #3816, 'distance_accuracy_value', 'NONE');
#23889=ADVANCED_FACE ( 'NONE', ( #14388 ), #10198, .F. ) ;
#23901=CARTESIAN_POINT ( 'NONE',  ( 140.0707155294784911, -11.09459640813488690, 4.575173035329051174 ) ) ;
#23902=AXIS2_PLACEMENT_3D ( 'NONE', #7300, #21138, #23300 ) ;
#23903=AXIS2_PLACEMENT_3D ( 'NONE', #6451, #23521, #16182 ) ;
#23905=CARTESIAN_POINT ( 'NONE',  ( 143.6175748654052597, 5.500000000000012434, -2.278174593052012309 ) ) ;
#23908=CARTESIAN_POINT ( 'NONE',  ( 148.7738248654052597, -3.889087296526011706, 3.889087296526011706 ) ) ;
#23910=DIRECTION ( 'NONE',  ( 0.000000000000000000, 0.000000000000000000, -1.000000000000000000 ) ) ;
#23913=CARTESIAN_POINT ( 'NONE',  ( 157.5148502691896510, -3.535533905932725318, -3.535533905932725318 ) ) ;
#23915=AXIS2_PLACEMENT_3D ( 'NONE', #29996, #27982, #1737 ) ;
#23926=COLOUR_RGB ( '', 0.40784314, 0.44705882, 0.49803922) ;
#23927=EDGE_CURVE ( 'NONE', #6918, #17372, #9729, .T. ) ;
#23936=ORIENTED_EDGE ( 'NONE', *, *, #22351, .F. ) ;
#23941=CARTESIAN_POINT ( 'NONE',  ( 134.3288997308104058, 4.999999999999989342, -2.071067811865468400 ) ) ;
#23945=CARTESIAN_POINT ( 'NONE',  ( 124.9999999999999432, -69.50000000000000000, -7.500000000000007105 ) ) ;
#23946=FILL_AREA_STYLE ('',( #25936 ) ) ;
#23956=DIRECTION ( 'NONE',  ( 0.000000000000000000, 0.000000000000000000, -1.000000000000000000 ) ) ;
#23960=ADVANCED_FACE ( 'NONE', ( #10976 ), #1414, .F. ) ;
#23964=DIRECTION ( 'NONE',  ( 1.000000000000000000, 0.000000000000000000, 0.000000000000000000 ) ) ;
#23970=CARTESIAN_POINT ( 'NONE',  ( 132.6562500000000284, -6.000000000000005329, 2.485281374238555774 ) ) ;
#23971=CARTESIAN_POINT ( 'NONE',  ( 160.8750000000000568, 0.000000000000000000, 6.000000000000005329 ) ) ;
#23972=ORIENTED_EDGE ( 'NONE', *, *, #26161, .F. ) ;
#23978=CARTESIAN_POINT ( 'NONE',  ( 135.2663997308104342, -4.999999999999989342, -2.071067811865468400 ) ) ;
#23979=FACE_OUTER_BOUND ( 'NONE', #2213, .T. ) ;
#23984=CARTESIAN_POINT ( 'NONE',  ( 0.9568781502952149465, -15.26121788209296959, -8.567725837855926230 ) ) ;
#23989=ADVANCED_FACE ( 'NONE', ( #26894 ), #15438, .F. ) ;
#23990=VECTOR ( 'NONE', #2162, 1000.000000000000000 ) ;
#23993=CARTESIAN_POINT ( 'NONE',  ( 136.1250000000000284, 0.000000000000000000, -6.000000000000005329 ) ) ;
#23995=DIRECTION ( 'NONE',  ( 1.000000000000000000, 0.000000000000000000, 0.000000000000000000 ) ) ;
#23998=CARTESIAN_POINT ( 'NONE',  ( -1.000000000000000888, 11.00000000000001066, 4.000000000000003553 ) ) ;
#24000=ORIENTED_EDGE ( 'NONE', *, *, #4595, .T. ) ;
#24004=CARTESIAN_POINT ( 'NONE',  ( 159.2870157019986550, -12.02748541700689522, -3.967488760539278125 ) ) ;
#24010=DIRECTION ( 'NONE',  ( -1.000000000000000000, -0.000000000000000000, -0.000000000000000000 ) ) ;
#24011=CARTESIAN_POINT ( 'NONE',  ( 140.8038234968595646, -11.90191174842906108, -4.000000000000003553 ) ) ;
#24015=CARTESIAN_POINT ( 'NONE',  ( 139.8373098077242105, -9.046954833815613384, 7.886428923425581772 ) ) ;
#24020=( NAMED_UNIT ( * ) SI_UNIT ( $, .STERADIAN. ) SOLID_ANGLE_UNIT ( ) );
#24021=CARTESIAN_POINT ( 'NONE',  ( 147.1086002691896510, -2.071067811865468400, -4.999999999999989342 ) ) ;
#24022=CARTESIAN_POINT ( 'NONE',  ( 150.4687500000000284, -2.485281374238585972, 6.000000000000005329 ) ) ;
#24028=CIRCLE ( 'NONE', #16231, 0.5000000000000004441 ) ;
#24029=CARTESIAN_POINT ( 'NONE',  ( 152.4375000000000284, -4.242640687119298093, -4.242640687119298093 ) ) ;
#24030=VECTOR ( 'NONE', #13752, 1000.000000000000000 ) ;
#24039=ORIENTED_EDGE ( 'NONE', *, *, #25044, .F. ) ;
#24041=EDGE_CURVE ( 'NONE', #9495, #12642, #13748, .T. ) ;
#24065=AXIS2_PLACEMENT_3D ( 'NONE', #24556, #10455, #27010 ) ;
#24072=ORIENTED_EDGE ( 'NONE', *, *, #26161, .T. ) ;
#24076=CARTESIAN_POINT ( 'NONE',  ( 131.9851497308104058, -3.535533905932725318, 3.535533905932725318 ) ) ;
#24079=EDGE_LOOP ( 'NONE', ( #26059, #28927, #12776, #6550 ) ) ;
#24081=CARTESIAN_POINT ( 'NONE',  ( 141.4613248654052597, -5.500000000000005329, 0.000000000000000000 ) ) ;
#24086=DIRECTION ( 'NONE',  ( 0.000000000000000000, 0.000000000000000000, -1.000000000000000000 ) ) ;
#24087=DIRECTION ( 'NONE',  ( 1.000000000000000000, -0.000000000000000000, -0.000000000000000000 ) ) ;
#24092=DIRECTION ( 'NONE',  ( 0.000000000000000000, 0.000000000000000000, -1.000000000000000000 ) ) ;
#24097=DIRECTION ( 'NONE',  ( -0.000000000000000000, -0.000000000000000000, -1.000000000000000000 ) ) ;
#24098=FACE_OUTER_BOUND ( 'NONE', #11463, .T. ) ;
#24101=CARTESIAN_POINT ( 'NONE',  ( 0.000000000000000000, -9.500000000000008882, -7.500000000000007105 ) ) ;
#24103=ORIENTED_EDGE ( 'NONE', *, *, #1051, .T. ) ;
#24106=ORIENTED_EDGE ( 'NONE', *, *, #29806, .F. ) ;
#24108=CARTESIAN_POINT ( 'NONE',  ( 135.6711002691896795, 4.999999999999989342, 2.071067811865468400 ) ) ;
#24109=STYLED_ITEM ( 'NONE', ( #21344 ), #29379 ) ;
#24110=CARTESIAN_POINT ( 'NONE',  ( 157.3050748654052029, 5.500000000000012434, 2.278174593052012309 ) ) ;
#24120=CARTESIAN_POINT ( 'NONE',  ( 135.6413997308104058, 2.071067811865468400, -4.999999999999989342 ) ) ;
#24122=CARTESIAN_POINT ( 'NONE',  ( 15.00000000000000000, 0.000000000000000000, 17.50000000000000355 ) ) ;
#24124=VECTOR ( 'NONE', #1910, 1000.000000000000000 ) ;
#24129=ADVANCED_FACE ( 'NONE', ( #14060 ), #22971, .T. ) ;
#24131=PRESENTATION_STYLE_ASSIGNMENT (( #8132 ) ) ;
#24133=VECTOR ( 'NONE', #5933, 1000.000000000000000 ) ;
#24135=B_SPLINE_CURVE_WITH_KNOTS ( 'NONE', 3,
 ( #24378, #10894, #6099, #1025, #12904, #24682 ),
 .UNSPECIFIED., .F., .F.,
 ( 4, 2, 4 ),
 ( 0.000000000000000000, 0.001072522389057928034, 0.002145044778115856067 ),
 .UNSPECIFIED. ) ;
#24140=CARTESIAN_POINT ( 'NONE',  ( 158.9136751345948539, 0.000000000000000000, -5.500000000000005329 ) ) ;
#24141=DIRECTION ( 'NONE',  ( 0.000000000000000000, 1.776356839400250465E-15, 1.000000000000000000 ) ) ;
#24143=CARTESIAN_POINT ( 'NONE',  ( -19.99999999999998224, -54.99999999999990763, 8.000000000000007105 ) ) ;
#24147=EDGE_LOOP ( 'NONE', ( #8099, #26873, #10186, #2980 ) ) ;
#24148=CARTESIAN_POINT ( 'NONE',  ( 159.1298473403915068, -11.07692307692306777, 4.615384615384606093 ) ) ;
#24151=CARTESIAN_POINT ( 'NONE',  ( 140.1636751345948255, 0.000000000000000000, 5.500000000000005329 ) ) ;
#24158=CARTESIAN_POINT ( 'NONE',  ( 140.4088296780374776, -11.40882967803863934, -4.170790813163522515 ) ) ;
#24162=CARTESIAN_POINT ( 'NONE',  ( 139.6504835472090349, -9.198789620363742259, 7.981988490022517979 ) ) ;
#24164=CARTESIAN_POINT ( 'NONE',  ( 139.9761751345948539, 3.889087296526011706, 3.889087296526011706 ) ) ;
#24165=PRESENTATION_STYLE_ASSIGNMENT (( #12532 ) ) ;
#24169=DIRECTION ( 'NONE',  ( 0.000000000000000000, 0.000000000000000000, 1.000000000000000000 ) ) ;
#24171=CARTESIAN_POINT ( 'NONE',  ( 146.2648502691896510, 3.535533905932725318, 3.535533905932752852 ) ) ;
#24172=CARTESIAN_POINT ( 'NONE',  ( 151.5937500000000284, 6.000000000000005329, 2.485281374238585972 ) ) ;
#24173=DIRECTION ( 'NONE',  ( -7.155734338404322954E-15, 0.000000000000000000, 1.000000000000000000 ) ) ;
#24177=CARTESIAN_POINT ( 'NONE',  ( 142.5937500000000568, 6.000000000000005329, 2.485281374238585972 ) ) ;
#24179=DIRECTION ( 'NONE',  ( -6.938893903907250071E-16, 0.6000000000000006439, -0.7999999999999997113 ) ) ;
#24191=CARTESIAN_POINT ( 'NONE',  ( 140.0769230769231228, -11.53846153846155254, 4.615384615384630074 ) ) ;
#24195=CARTESIAN_POINT ( 'NONE',  ( -1.000000000000000888, -19.99999999999998934, 4.000000000000003553 ) ) ;
#24202=DIRECTION ( 'NONE',  ( 1.000000000000000000, 0.000000000000000000, 0.000000000000000000 ) ) ;
#24204=ORIENTED_EDGE ( 'NONE', *, *, #3831, .T. ) ;
#24205=CARTESIAN_POINT ( 'NONE',  ( 160.7812500000000568, 2.485281374238585972, 6.000000000000005329 ) ) ;
#24210=CARTESIAN_POINT ( 'NONE',  ( 147.0000000000000284, 6.000000000000005329, 0.000000000000000000 ) ) ;
#24211=ORIENTED_EDGE ( 'NONE', *, *, #7025, .F. ) ;
#24219=CARTESIAN_POINT ( 'NONE',  ( 135.0000000000000000, -7.391412244009264221, 8.245343090279524390 ) ) ;
#24223=CARTESIAN_POINT ( 'NONE',  ( -0.04562205425674302484, -14.49999999999998046, -8.291335958003948292 ) ) ;
#24225=CARTESIAN_POINT ( 'NONE',  ( -9.999999999999980460, -60.00000000000001421, 4.000000000000003553 ) ) ;
#24232=( NAMED_UNIT ( * ) SI_UNIT ( $, .STERADIAN. ) SOLID_ANGLE_UNIT ( ) );
#24234=DIRECTION ( 'NONE',  ( 1.000000000000000000, 0.000000000000000000, 0.000000000000000000 ) ) ;
#24235=ORIENTED_EDGE ( 'NONE', *, *, #4133, .F. ) ;
#24244=DIRECTION ( 'NONE',  ( 1.000000000000000000, 0.000000000000000000, 0.000000000000000000 ) ) ;
#24245=ORIENTED_EDGE ( 'NONE', *, *, #8784, .F. ) ;
#24246=CARTESIAN_POINT ( 'NONE',  ( -4.999999999999990230, -24.99999999999999289, 7.500000000000007105 ) ) ;
#24247=ORIENTED_EDGE ( 'NONE', *, *, #28701, .T. ) ;
#24249=CARTESIAN_POINT ( 'NONE',  ( 161.8125000000000284, 4.242640687119298093, -4.242640687119298093 ) ) ;
#24250=ORIENTED_EDGE ( 'NONE', *, *, #11726, .T. ) ;
#24259=CARTESIAN_POINT ( 'NONE',  ( 138.9226497308104342, 5.000000000000004441, 0.000000000000000000 ) ) ;
#24266=CARTESIAN_POINT ( 'NONE',  ( 116.0000000000000142, 0.000000000000000000, 0.000000000000000000 ) ) ;
#24273=CARTESIAN_POINT ( 'NONE',  ( 153.8363248654052029, 0.000000000000000000, -5.500000000000005329 ) ) ;
#24277=CARTESIAN_POINT ( 'NONE',  ( 135.7500000000000284, -6.000000000000005329, 0.000000000000000000 ) ) ;
#24279=EDGE_CURVE ( 'NONE', #13349, #7272, #7569, .T. ) ;
#24285=CARTESIAN_POINT ( 'NONE',  ( 140.6818792730027781, -11.36375854600488644, 4.222310544175423175 ) ) ;
#24286=ADVANCED_FACE ( 'NONE', ( #21834 ), #732, .F. ) ;
#24292=CARTESIAN_POINT ( 'NONE',  ( 159.5699251345948255, 2.278174593052136210, 5.499999999999888978 ) ) ;
#24293=CARTESIAN_POINT ( 'NONE',  ( 135.0000000000000284, 0.000000000000000000, 0.000000000000000000 ) ) ;
#24295=CARTESIAN_POINT ( 'NONE',  ( 153.1726497308104058, -5.000000000000004441, 0.000000000000000000 ) ) ;
#24298=( NAMED_UNIT ( * ) SI_UNIT ( $, .STERADIAN. ) SOLID_ANGLE_UNIT ( ) );
#24300=AXIS2_PLACEMENT_3D ( 'NONE', #25454, #23189, #4111 ) ;
#24303=CARTESIAN_POINT ( 'NONE',  ( 140.1636751345948255, 0.000000000000000000, 5.500000000000005329 ) ) ;
#24306=DIRECTION ( 'NONE',  ( 0.000000000000000000, 0.000000000000000000, -1.000000000000000000 ) ) ;
#24307=ORIENTED_EDGE ( 'NONE', *, *, #18246, .T. ) ;
#24308=CARTESIAN_POINT ( 'NONE',  ( 140.1711002691896795, 4.999999999999989342, 2.071067811865468400 ) ) ;
#24309=CARTESIAN_POINT ( 'NONE',  ( 149.9062500000000568, 6.000000000000005329, -2.485281374238556218 ) ) ;
#24310=DIRECTION ( 'NONE',  ( -0.000000000000000000, -1.000000000000000000, -0.000000000000000000 ) ) ;
#24314=ORIENTED_EDGE ( 'NONE', *, *, #8081, .T. ) ;
#24315=CARTESIAN_POINT ( 'NONE',  ( 142.5000000000000568, 6.000000000000005329, 0.000000000000000000 ) ) ;
#24317=EDGE_CURVE ( 'NONE', #20296, #19034, #24472, .T. ) ;
#24318=CARTESIAN_POINT ( 'NONE',  ( 116.0000000000000142, 6.735557395310442023E-16, 5.500000000000000000 ) ) ;
#24327=CARTESIAN_POINT ( 'NONE',  ( -4.999999999999990230, -55.00000000000002132, 5.000000000000004441 ) ) ;
#24328=DIRECTION ( 'NONE',  ( 0.000000000000000000, 0.000000000000000000, 1.000000000000000000 ) ) ;
#24338=CYLINDRICAL_SURFACE ( 'NONE', #22129, 0.5000000000000004441 ) ;
#24340=CARTESIAN_POINT ( 'NONE',  ( 152.9211002691896795, -4.999999999999989342, -2.071067811865468400 ) ) ;
#24342=CARTESIAN_POINT ( 'NONE',  ( 161.4590559403349630, -3.334791428567227989, -4.957026983497794248 ) ) ;
#24343=AXIS2_PLACEMENT_3D ( 'NONE', #22934, #4016, #13433 ) ;
#24348=DIRECTION ( 'NONE',  ( 1.000000000000000000, 0.000000000000000000, -0.000000000000000000 ) ) ;
#24351=ADVANCED_FACE ( 'NONE', ( #7601 ), #17936, .T. ) ;
#24352=ORIENTED_EDGE ( 'NONE', *, *, #26398, .F. ) ;
#24353=FILL_AREA_STYLE ('',( #21921 ) ) ;
#24354=DIRECTION ( 'NONE',  ( 0.000000000000000000, 0.9165151389911677660, -0.4000000000000004663 ) ) ;
#24355=CARTESIAN_POINT ( 'NONE',  ( 146.0699251345948255, 2.278174593052290753, 5.499999999999732658 ) ) ;
#24361=CARTESIAN_POINT ( 'NONE',  ( 146.3437500000000568, -6.000000000000005329, -2.485281374238555774 ) ) ;
#24364=AXIS2_PLACEMENT_3D ( 'NONE', #11295, #11133, #27373 ) ;
#24367=ORIENTED_EDGE ( 'NONE', *, *, #25187, .T. ) ;
#24371=VECTOR ( 'NONE', #10488, 1000.000000000000000 ) ;
#24374=ORIENTED_EDGE ( 'NONE', *, *, #9466, .F. ) ;
#24378=CARTESIAN_POINT ( 'NONE',  ( 1.000000000000000888, -16.43939393939394833, -5.999693900976793337 ) ) ;
#24379=AXIS2_PLACEMENT_3D ( 'NONE', #11498, #30035, #27713 ) ;
#24384=CARTESIAN_POINT ( 'NONE',  ( 155.0550748654052313, -5.500000000000012434, -2.278174593052012309 ) ) ;
#24387=FACE_OUTER_BOUND ( 'NONE', #21356, .T. ) ;
#24394=CARTESIAN_POINT ( 'NONE',  ( -4.999999999999886313, -15.00000000000001421, 8.000000000000007105 ) ) ;
#24395=MECHANICAL_DESIGN_GEOMETRIC_PRESENTATION_REPRESENTATION('',(#29812),#8733);
#24396=EDGE_CURVE ( 'NONE', #25843, #9799, #14851, .T. ) ;
#24403=CIRCLE ( 'NONE', #26837, 0.5000000000000006661 ) ;
#24404=ORIENTED_EDGE ( 'NONE', *, *, #30362, .F. ) ;
#24405=CARTESIAN_POINT ( 'NONE',  ( 161.0625000000000284, -4.242640687119298093, 4.242640687119298093 ) ) ;
#24408=CARTESIAN_POINT ( 'NONE',  ( -39.00000000000000000, -20.00000000000021316, -3.000000000000002665 ) ) ;
#24411=VECTOR ( 'NONE', #20520, 1000.000000000000000 ) ;
#24413=CARTESIAN_POINT ( 'NONE',  ( -4.999999999999990230, -55.00000000000002132, 8.000000000000007105 ) ) ;
#24415=CARTESIAN_POINT ( 'NONE',  ( 134.7976497308104058, 0.000000000000000000, 5.000000000000004441 ) ) ;
#24419=SURFACE_STYLE_FILL_AREA ( #7982 ) ;
#24423=FILL_AREA_STYLE_COLOUR ( '', #3375 ) ;
#24426=CARTESIAN_POINT ( 'NONE',  ( 153.4613248654052029, -5.500000000000005329, 0.000000000000000000 ) ) ;
#24427=DIRECTION ( 'NONE',  ( 0.000000000000000000, 0.000000000000000000, 1.000000000000000000 ) ) ;
#24431=CARTESIAN_POINT ( 'NONE',  ( 135.9375000000000568, -4.242640687119298093, -4.242640687119298093 ) ) ;
#24438=CARTESIAN_POINT ( 'NONE',  ( 160.3057606286754435, -11.25150511129604780, 4.172711468660709855 ) ) ;
#24444=CARTESIAN_POINT ( 'NONE',  ( 155.7976497308104342, 0.000000000000000000, 5.000000000000004441 ) ) ;
#24453=ADVANCED_FACE ( 'NONE', ( #3140 ), #26221, .T. ) ;
#24455=CYLINDRICAL_SURFACE ( 'NONE', #10165, 1.000000000000000888 ) ;
#24457=CARTESIAN_POINT ( 'NONE',  ( 151.3125000000000568, 4.242640687119298093, -4.242640687119298093 ) ) ;
#24462=ORIENTED_EDGE ( 'NONE', *, *, #977, .F. ) ;
#24463=CARTESIAN_POINT ( 'NONE',  ( 146.2500000000000568, -6.000000000000005329, 0.000000000000000000 ) ) ;
#24464=CARTESIAN_POINT ( 'NONE',  ( 161.2222053800996093, -4.042477648134306101, 4.062297615371217141 ) ) ;
#24466=COLOUR_RGB ( '', 0.72549020, 0.75294118, 0.79215686) ;
#24469=ORIENTED_EDGE ( 'NONE', *, *, #11942, .F. ) ;
#24472=B_SPLINE_CURVE_WITH_KNOTS ( 'NONE', 3,
 ( #8128, #19677, #1076, #10466, #24570, #3519, #12949, #29326, #10389, #28630, #19741, #17616, #2995, #5441, #22205, #17317, #10539, #842 ),
 .UNSPECIFIED., .F., .F.,
 ( 4, 2, 2, 2, 2, 2, 2, 2, 4 ),
 ( 0.006357437601277660111, 0.007224154817333453514, 0.008090872033389246917, 0.008957589249445039453, 0.009824306465500833724, 0.01069102368155662626, 0.01155774089761241880, 0.01242445811366821307, 0.01329117532972400560 ),
 .UNSPECIFIED. ) ;
#24475=ORIENTED_EDGE ( 'NONE', *, *, #19654, .F. ) ;
#24479=CARTESIAN_POINT ( 'NONE',  ( 148.2113248654052313, 5.500000000000005329, 0.000000000000000000 ) ) ;
#24488=CARTESIAN_POINT ( 'NONE',  ( 140.3363248654052029, 0.000000000000000000, -5.500000000000005329 ) ) ;
#24491=CIRCLE ( 'NONE', #12294, 30.00000000000000000 ) ;
#24492=CARTESIAN_POINT ( 'NONE',  ( 152.0773502691896510, 5.000000000000004441, 0.000000000000000000 ) ) ;
#24493=CARTESIAN_POINT ( 'NONE',  ( 150.6636751345948255, 0.000000000000000000, 5.500000000000005329 ) ) ;
#24494=CARTESIAN_POINT ( 'NONE',  ( 139.5985279861999686, -9.179712423653196396, -7.992169671736488290 ) ) ;
#24495=AXIS2_PLACEMENT_3D ( 'NONE', #18009, #1838, #6289 ) ;
#24499=CARTESIAN_POINT ( 'NONE',  ( 150.6488248654052029, -3.889087296526011706, -3.889087296526011706 ) ) ;
#24511=ORIENTED_EDGE ( 'NONE', *, *, #12480, .F. ) ;
#24513=TOROIDAL_SURFACE ( 'NONE', #29917, 15.99999999999999289, 1.000000000000000000 ) ;
#24514=CARTESIAN_POINT ( 'NONE',  ( 135.0000000000000284, -6.982120021884474781, 8.500000000000007105 ) ) ;
#24516=EDGE_CURVE ( 'NONE', #3348, #10268, #10242, .T. ) ;
#24532=CARTESIAN_POINT ( 'NONE',  ( 135.0000000000000284, -9.047800747817580813, -7.500000000000007105 ) ) ;
#24541=ORIENTED_EDGE ( 'NONE', *, *, #1092, .T. ) ;
#24543=CARTESIAN_POINT ( 'NONE',  ( 139.1175748654052029, 5.500000000000012434, -2.278174593052012309 ) ) ;
#24550=CARTESIAN_POINT ( 'NONE',  ( 155.1562500000000284, -6.000000000000005329, 2.485281374238555774 ) ) ;
#24552=ORIENTED_EDGE ( 'NONE', *, *, #23724, .T. ) ;
#24556=CARTESIAN_POINT ( 'NONE',  ( -10.00000000000000178, -19.99999999999998934, -3.000000000000002665 ) ) ;
#24557=AXIS2_PLACEMENT_3D ( 'NONE', #9927, #1130, #5735 ) ;
#24562=EDGE_CURVE ( 'NONE', #26257, #14826, #27379, .T. ) ;
#24563=( GEOMETRIC_REPRESENTATION_CONTEXT ( 3 ) GLOBAL_UNCERTAINTY_ASSIGNED_CONTEXT ( ( #19896 ) ) GLOBAL_UNIT_ASSIGNED_CONTEXT ( ( #13024, #13187, #3754 ) ) REPRESENTATION_CONTEXT ( 'NONE', 'WORKASPACE' ) );
#24564=DIRECTION ( 'NONE',  ( 0.000000000000000000, 0.000000000000000000, 1.000000000000000000 ) ) ;
#24566=DIRECTION ( 'NONE',  ( -0.000000000000000000, -0.000000000000000000, -1.000000000000000000 ) ) ;
#24569=CARTESIAN_POINT ( 'NONE',  ( 161.0000000000000284, -11.67610212985248452, 2.769230769230773603 ) ) ;
#24570=CARTESIAN_POINT ( 'NONE',  ( 135.0000000000000284, 3.276830707260631304, 4.562445581355718538 ) ) ;
#24571=FACE_OUTER_BOUND ( 'NONE', #6124, .T. ) ;
#24575=EDGE_LOOP ( 'NONE', ( #2294, #13166, #8105, #20612 ) ) ;
#24581=ORIENTED_EDGE ( 'NONE', *, *, #13835, .T. ) ;
#24586=CARTESIAN_POINT ( 'NONE',  ( 155.5386751345948539, -5.500000000000005329, 0.000000000000000000 ) ) ;
#24588=CARTESIAN_POINT ( 'NONE',  ( 141.0000000000000284, -12.00000000000001066, 4.000000000000003553 ) ) ;
#24592=CARTESIAN_POINT ( 'NONE',  ( 136.5863248654052313, 0.000000000000000000, 5.500000000000005329 ) ) ;
#24599=CARTESIAN_POINT ( 'NONE',  ( 151.9538997308104058, -2.071067811865468400, -4.999999999999989342 ) ) ;
#24612=ORIENTED_EDGE ( 'NONE', *, *, #20191, .F. ) ;
#24613=CARTESIAN_POINT ( 'NONE',  ( 144.0000000000000284, 6.000000000000005329, 0.000000000000000000 ) ) ;
#24614=CARTESIAN_POINT ( 'NONE',  ( 141.7574251345948255, -2.278174593051702335, 5.500000000000323297 ) ) ;
#24620=CARTESIAN_POINT ( 'NONE',  ( 146.9062500000000284, 6.000000000000005329, -2.485281374238555774 ) ) ;
#24621=CARTESIAN_POINT ( 'NONE',  ( 143.0550748654052313, -5.500000000000012434, -2.278174593052012309 ) ) ;
#24622=EDGE_CURVE ( 'NONE', #9799, #2895, #25238, .T. ) ;
#24632=EDGE_CURVE ( 'NONE', #5384, #19330, #4851, .T. ) ;
#24639=DIRECTION ( 'NONE',  ( 1.000000000000000000, -0.000000000000000000, -0.000000000000000000 ) ) ;
#24651=CARTESIAN_POINT ( 'NONE',  ( 154.7023502691896510, 0.000000000000000000, -5.000000000000004441 ) ) ;
#24655=LINE ( 'NONE', #3602, #6018 ) ;
#24660=( NAMED_UNIT ( * ) PLANE_ANGLE_UNIT ( ) SI_UNIT ( $, .RADIAN. ) );
#24671=CIRCLE ( 'NONE', #25674, 1.000000000000000888 ) ;
#24673=ORIENTED_EDGE ( 'NONE', *, *, #15664, .F. ) ;
#24675=CARTESIAN_POINT ( 'NONE',  ( 135.0000000000000284, -8.656813570721347162, 7.548387214344470131 ) ) ;
#24679=LINE ( 'NONE', #3620, #12290 ) ;
#24682=CARTESIAN_POINT ( 'NONE',  ( 0.7669223171414829565, -15.58766199952932396, -7.954545454545463912 ) ) ;
#24687=CARTESIAN_POINT ( 'NONE',  ( -0.02602735246118784845, -9.486986323769393437, 4.738252045315884509 ) ) ;
#24697=CARTESIAN_POINT ( 'NONE',  ( -0.5000000000000004441, -10.50000000000000888, 8.000000000000007105 ) ) ;
#24699=ORIENTED_EDGE ( 'NONE', *, *, #20383, .T. ) ;
#24708=CARTESIAN_POINT ( 'NONE',  ( 155.3437500000000284, -6.000000000000005329, -2.485281374238555774 ) ) ;
#24710=EDGE_CURVE ( 'NONE', #15017, #13841, #24755, .T. ) ;
#24715=( NAMED_UNIT ( * ) PLANE_ANGLE_UNIT ( ) SI_UNIT ( $, .RADIAN. ) );
#24725=CARTESIAN_POINT ( 'NONE',  ( 140.0000000000000284, -11.45643923738959202, 5.000000000000004441 ) ) ;
#24738=CARTESIAN_POINT ( 'NONE',  ( 160.2113248654052313, 5.500000000000005329, 0.000000000000000000 ) ) ;
#24741=DIRECTION ( 'NONE',  ( 0.000000000000000000, 1.000000000000000000, 0.000000000000000000 ) ) ;
#24744=( NAMED_UNIT ( * ) SI_UNIT ( $, .STERADIAN. ) SOLID_ANGLE_UNIT ( ) );
#24747=CARTESIAN_POINT ( 'NONE',  ( 135.0000000000000568, 5.117427953996132040, -2.736531087928903094 ) ) ;
#24752=CARTESIAN_POINT ( 'NONE',  ( 159.2804190760031702, -12.03105614890318265, 3.962454373193818657 ) ) ;
#24753=AXIS2_PLACEMENT_3D ( 'NONE', #782, #27175, #29019 ) ;
#24754=CARTESIAN_POINT ( 'NONE',  ( 143.6250000000000284, 0.000000000000000000, -6.000000000000005329 ) ) ;
#24755=CIRCLE ( 'NONE', #10052, 0.5000000000000004441 ) ;
#24758=CARTESIAN_POINT ( 'NONE',  ( 159.1949251345948255, 5.500000000000012434, -2.278174593052012309 ) ) ;
#24762=CARTESIAN_POINT ( 'NONE',  ( 136.0000000000000284, -9.165151389911695645, -8.000000000000007105 ) ) ;
#24763=CARTESIAN_POINT ( 'NONE',  ( 150.7351497308104342, 3.535533905932725318, -3.535533905932725318 ) ) ;
#24772=APPLICATION_CONTEXT ( 'automotive_design' ) ;
#24776=ORIENTED_EDGE ( 'NONE', *, *, #3639, .T. ) ;
#24778=CARTESIAN_POINT ( 'NONE',  ( 147.0000000000000284, 6.000000000000005329, 0.000000000000000000 ) ) ;
#24780=SURFACE_STYLE_USAGE ( .BOTH. , #15923 ) ;
#24783=CARTESIAN_POINT ( 'NONE',  ( 143.4375000000000284, -4.242640687119298093, -4.242640687119298093 ) ) ;
#24784=CARTESIAN_POINT ( 'NONE',  ( 161.1372372713044570, -1.259261447730557926, 5.503929387713502486 ) ) ;
#24786=AXIS2_PLACEMENT_3D ( 'NONE', #19471, #10099, #21479 ) ;
#24790=ORIENTED_EDGE ( 'NONE', *, *, #13655, .F. ) ;
#24794=PRESENTATION_STYLE_ASSIGNMENT (( #7896 ) ) ;
#24796=CARTESIAN_POINT ( 'NONE',  ( 136.0000000000000284, -8.798545334315205579, -8.160000000000000142 ) ) ;
#24799=CARTESIAN_POINT ( 'NONE',  ( 136.8675748654052313, -5.500000000000012434, 2.278174593052012309 ) ) ;
#24802=UNCERTAINTY_MEASURE_WITH_UNIT (LENGTH_MEASURE( 1.000000000000000082E-05 ), #30165, 'distance_accuracy_value', 'NONE');
#24809=CARTESIAN_POINT ( 'NONE',  ( 161.5000000000000853, -2.984449860524901688, -5.205099329504969674 ) ) ;
#24810=CARTESIAN_POINT ( 'NONE',  ( 135.3824251345948539, 5.500000000000012434, 2.278174593052012309 ) ) ;
#24816=EDGE_CURVE ( 'NONE', #2367, #15417, #15041, .T. ) ;
#24817=EDGE_LOOP ( 'NONE', ( #10572, #10448, #15378, #16491 ) ) ;
#24818=CARTESIAN_POINT ( 'NONE',  ( 0.000000000000000000, -15.50000000000001421, 5.656854249492387687 ) ) ;
#24824=COLOUR_RGB ( '', 0.09019608, 0.27058824, 0.51372549) ;
#24831=ORIENTED_EDGE ( 'NONE', *, *, #14220, .F. ) ;
#24832=CARTESIAN_POINT ( 'NONE',  ( 0.000000000000000000, 11.00000000000001066, -3.000000000000002665 ) ) ;
#24836=STYLED_ITEM ( 'NONE', ( #3211 ), #13558 ) ;
#24838=CARTESIAN_POINT ( 'NONE',  ( -0.7382520721438935452, -9.130873963928037185, 4.026027341348664912 ) ) ;
#24839=EDGE_CURVE ( 'NONE', #25384, #26506, #10994, .T. ) ;
#24844=VERTEX_POINT ( 'NONE', #17284 ) ;
#24848=ADVANCED_FACE ( 'NONE', ( #26744 ), #2814, .F. ) ;
#24855=VERTEX_POINT ( 'NONE', #26258 ) ;
#24857=VERTEX_POINT ( 'NONE', #613 ) ;
#24858=CARTESIAN_POINT ( 'NONE',  ( 154.5000000000000284, 6.000000000000005329, 0.000000000000000000 ) ) ;
#24859=( BOUNDED_SURFACE ( )  B_SPLINE_SURFACE ( 3, 2, ( 
 ( #2107, #13978, #4846 ),
 ( #23470, #14274, #2408 ),
 ( #11820, #14423, #96 ),
 ( #19455, #19597, #21607 ),
 ( #540, #14991, #3283 ),
 ( #29084, #3429, #17459 ),
 ( #12861, #12412, #26773 ),
 ( #28626, #21756, #2844 ) ),
 .UNSPECIFIED., .F., .F., .F. ) 
 B_SPLINE_SURFACE_WITH_KNOTS ( ( 4, 2, 2, 4 ),
 ( 3, 3 ),
 ( 0.006483209092139505421, 0.007220185479624316449, 0.007957161867109126610, 0.009431114642078748667 ),
 ( 0.000000000000000000, 1.000000000000000000 ),
 .UNSPECIFIED. ) 
 GEOMETRIC_REPRESENTATION_ITEM ( )  RATIONAL_B_SPLINE_SURFACE ( (
 ( 1.000000000000000000, 0.9165151389911680990, 1.000000000000000000),
 ( 1.000000000000000000, 0.9165811099393400552, 1.000000000000000000),
 ( 1.000000000000000000, 0.9096513889650220674, 1.000000000000000000),
 ( 1.000000000000000000, 0.8858533194329228921, 1.000000000000000000),
 ( 1.000000000000000000, 0.8692663461314428242, 1.000000000000000000),
 ( 1.000000000000000000, 0.8111162787391891227, 1.000000000000000000),
 ( 1.000000000000000000, 0.7613968795875392104, 1.000000000000000000),
 ( 1.000000000000000000, 0.7050799574999858654, 1.000000000000000000) ) ) 
 REPRESENTATION_ITEM ( '' )  SURFACE ( )  );
#24862=EDGE_LOOP ( 'NONE', ( #8823, #29727, #16375, #20559 ) ) ;
#24863=DIRECTION ( 'NONE',  ( 0.000000000000000000, 0.000000000000000000, 1.000000000000000000 ) ) ;
#24866=CARTESIAN_POINT ( 'NONE',  ( 159.8041075121309120, -12.29865543435749942, 3.608411551111435411 ) ) ;
#24868=ORIENTED_EDGE ( 'NONE', *, *, #14919, .T. ) ;
#24872=CARTESIAN_POINT ( 'NONE',  ( 139.8675748654052597, -5.500000000000012434, 2.278174593052012309 ) ) ;
#24879=EDGE_CURVE ( 'NONE', #23261, #27080, #4436, .T. ) ;
#24880=DIRECTION ( 'NONE',  ( 0.000000000000000000, 0.000000000000000000, 1.000000000000000000 ) ) ;
#24886=EDGE_CURVE ( 'NONE', #4566, #5384, #27990, .T. ) ;
#24887=CARTESIAN_POINT ( 'NONE',  ( 141.2023502691896510, 0.000000000000000000, -5.000000000000004441 ) ) ;
#24892=CARTESIAN_POINT ( 'NONE',  ( 135.0000000000000284, 2.497680721013432859, -4.958406755811053834 ) ) ;
#24894=ORIENTED_EDGE ( 'NONE', *, *, #7882, .F. ) ;
#24895=CARTESIAN_POINT ( 'NONE',  ( 138.6636751345948255, 0.000000000000000000, 5.500000000000005329 ) ) ;
#24896=CARTESIAN_POINT ( 'NONE',  ( 142.8750000000000284, 0.000000000000000000, 6.000000000000005329 ) ) ;
#24897=( GEOMETRIC_REPRESENTATION_CONTEXT ( 3 ) GLOBAL_UNCERTAINTY_ASSIGNED_CONTEXT ( ( #28476 ) ) GLOBAL_UNIT_ASSIGNED_CONTEXT ( ( #14760, #19655, #21960 ) ) REPRESENTATION_CONTEXT ( 'NONE', 'WORKASPACE' ) );
#24901=FILL_AREA_STYLE_COLOUR ( '', #826 ) ;
#24904=CARTESIAN_POINT ( 'NONE',  ( 1.000000000000000888, 0.000000000000000000, 0.000000000000000000 ) ) ;
#24906=CARTESIAN_POINT ( 'NONE',  ( 147.3601497308104058, -3.535533905932725318, -3.535533905932725318 ) ) ;
#24909=CARTESIAN_POINT ( 'NONE',  ( 136.0000000000000284, 1.469576158976823947E-15, 12.00000000000000178 ) ) ;
#24911=ADVANCED_FACE ( 'NONE', ( #20274 ), #7266, .T. ) ;
#24916=VERTEX_POINT ( 'NONE', #3960 ) ;
#24920=ORIENTED_EDGE ( 'NONE', *, *, #29730, .T. ) ;
#24922=CARTESIAN_POINT ( 'NONE',  ( 143.5312500000000284, -2.485281374238556218, -6.000000000000005329 ) ) ;
#24927=CARTESIAN_POINT ( 'NONE',  ( 135.7500000000000284, -6.000000000000005329, 0.000000000000000000 ) ) ;
#24928=CARTESIAN_POINT ( 'NONE',  ( 142.7738248654052313, -3.889087296526011706, 3.889087296526011706 ) ) ;
#24940=FACE_OUTER_BOUND ( 'NONE', #2394, .T. ) ;
#24945=CARTESIAN_POINT ( 'NONE',  ( -4.999999999999990230, -24.99999999999999289, 8.000000000000007105 ) ) ;
#24949=CARTESIAN_POINT ( 'NONE',  ( 154.7961002691896795, 2.071067811865468400, -4.999999999999989342 ) ) ;
#24955=DIRECTION ( 'NONE',  ( 0.000000000000000000, 0.000000000000000000, -1.000000000000000000 ) ) ;
#24956=ORIENTED_EDGE ( 'NONE', *, *, #11907, .T. ) ;
#24957=AXIS2_PLACEMENT_3D ( 'NONE', #3042, #593, #9979 ) ;
#24958=CARTESIAN_POINT ( 'NONE',  ( 154.5000000000000284, 6.000000000000005329, 0.000000000000000000 ) ) ;
#24962=EDGE_CURVE ( 'NONE', #691, #19810, #17444, .T. ) ;
#24968=PRESENTATION_STYLE_ASSIGNMENT (( #20693 ) ) ;
#24971=AXIS2_PLACEMENT_3D ( 'NONE', #20414, #3811, #6131 ) ;
#24972=ORIENTED_EDGE ( 'NONE', *, *, #6044, .T. ) ;
#24973=( BOUNDED_CURVE ( )  B_SPLINE_CURVE ( 2, ( #30243, #30397, #16321, #20743, #16169, #18147, #14017, #8761, #20897 ),
 .UNSPECIFIED., .F., .F. ) 
 B_SPLINE_CURVE_WITH_KNOTS ( ( 3, 2, 2, 2, 3 ),
 ( 0.1125000000000005579, 0.1187500000000003275, 0.1250000000000001110, 0.1312499999999998945, 0.1374999999999996780 ),
 .UNSPECIFIED. ) 
 CURVE ( )  GEOMETRIC_REPRESENTATION_ITEM ( )  RATIONAL_B_SPLINE_CURVE ( ( 0.9999999999999932276, 0.9238795325112935108, 1.000000000000000000, 0.9238795325112867385, 1.000000000000000000, 0.9238795325112867385, 1.000000000000000000, 0.9238795325112908463, 0.9999999999999958922 ) ) 
 REPRESENTATION_ITEM ( '' )  );
#24976=CARTESIAN_POINT ( 'NONE',  ( 146.2574251345948539, -2.278174593051733421, 5.500000000000292211 ) ) ;
#24981=CARTESIAN_POINT ( 'NONE',  ( 160.4136751345948824, 0.000000000000000000, -5.500000000000005329 ) ) ;
#24995=CIRCLE ( 'NONE', #22054, 16.00000000000000000 ) ;
#25000=MECHANICAL_DESIGN_GEOMETRIC_PRESENTATION_REPRESENTATION('',(#26946),#17674);
#25002=CARTESIAN_POINT ( 'NONE',  ( 157.9687500000000284, -2.485281374238585972, 6.000000000000005329 ) ) ;
#25006=VERTEX_POINT ( 'NONE', #22424 ) ;
#25012=ORIENTED_EDGE ( 'NONE', *, *, #18288, .T. ) ;
#25014=EDGE_CURVE ( 'NONE', #18697, #25268, #8902, .T. ) ;
#25016=DIRECTION ( 'NONE',  ( 1.000000000000000000, 0.000000000000000000, 0.000000000000000000 ) ) ;
#25022=DIRECTION ( 'NONE',  ( 0.000000000000000000, 0.000000000000000000, -1.000000000000000000 ) ) ;
#25026=AXIS2_PLACEMENT_3D ( 'NONE', #22426, #5658, #5971 ) ;
#25029=ORIENTED_EDGE ( 'NONE', *, *, #1254, .T. ) ;
#25031=CARTESIAN_POINT ( 'NONE',  ( 159.9300748654052029, 2.278174593051865315, -5.500000000000158984 ) ) ;
#25033=CARTESIAN_POINT ( 'NONE',  ( 137.6398502691896510, -3.535533905932752852, 3.535533905932725318 ) ) ;
#25039=CARTESIAN_POINT ( 'NONE',  ( 135.0000000000000000, 3.024630907472011465, -4.708032601928953120 ) ) ;
#25041=ORIENTED_EDGE ( 'NONE', *, *, #20670, .T. ) ;
#25043=CARTESIAN_POINT ( 'NONE',  ( 139.4062500000000284, 6.000000000000005329, -2.485281374238555774 ) ) ;
#25044=EDGE_CURVE ( 'NONE', #15395, #3348, #18133, .T. ) ;
#25051=EDGE_CURVE ( 'NONE', #30382, #9852, #23547, .T. ) ;
#25052=DIRECTION ( 'NONE',  ( 1.000000000000000000, 0.000000000000000000, 0.000000000000000000 ) ) ;
#25056=CARTESIAN_POINT ( 'NONE',  ( 151.7663997308104342, -4.999999999999989342, -2.071067811865468400 ) ) ;
#25057=DIRECTION ( 'NONE',  ( 1.000000000000000000, 0.000000000000000000, 0.000000000000000000 ) ) ;
#25064=ORIENTED_EDGE ( 'NONE', *, *, #4604, .T. ) ;
#25068=FACE_OUTER_BOUND ( 'NONE', #22634, .T. ) ;
#25069=EDGE_LOOP ( 'NONE', ( #24352, #19656, #16636, #15852 ) ) ;
#25071=CARTESIAN_POINT ( 'NONE',  ( 144.3750000000000284, 0.000000000000000000, 6.000000000000005329 ) ) ;
#25076=CARTESIAN_POINT ( 'NONE',  ( 137.7187500000000284, 2.485281374238555774, -6.000000000000005329 ) ) ;
#25085=AXIS2_PLACEMENT_3D ( 'NONE', #18910, #15866, #30396 ) ;
#25087=EDGE_CURVE ( 'NONE', #8567, #18033, #30389, .T. ) ;
#25088=VERTEX_POINT ( 'NONE', #4584 ) ;
#25094=CARTESIAN_POINT ( 'NONE',  ( -9.999999999999772626, -89.00000000000001421, 4.000000000000003553 ) ) ;
#25096=CIRCLE ( 'NONE', #9427, 1.000000000000000000 ) ;
#25099=DIRECTION ( 'NONE',  ( 1.000000000000000000, 0.000000000000000000, 0.000000000000000000 ) ) ;
#25101=CARTESIAN_POINT ( 'NONE',  ( 135.0000000000000284, -6.982120021884474781, 8.500000000000007105 ) ) ;
#25102=CARTESIAN_POINT ( 'NONE',  ( 148.3273502691896510, -5.000000000000004441, 0.000000000000000000 ) ) ;
#25107=LINE ( 'NONE', #8695, #24411 ) ;
#25108=CARTESIAN_POINT ( 'NONE',  ( 139.5000000000000000, -24.99999999999999289, 7.500000000000007105 ) ) ;
#25110=CARTESIAN_POINT ( 'NONE',  ( 158.4375000000000284, -4.242640687119298093, -4.242640687119298093 ) ) ;
#25113=EDGE_CURVE ( 'NONE', #605, #6232, #28396, .T. ) ;
#25114=ORIENTED_EDGE ( 'NONE', *, *, #24622, .F. ) ;
#25118=CARTESIAN_POINT ( 'NONE',  ( 0.000000000000000000, -9.500000000000008882, -5.000000000000004441 ) ) ;
#25119=CARTESIAN_POINT ( 'NONE',  ( 139.5000000000000284, -8.798545334315205579, -8.160000000000000142 ) ) ;
#25122=PRESENTATION_STYLE_ASSIGNMENT (( #17537 ) ) ;
#25125=DIRECTION ( 'NONE',  ( 1.000000000000000000, 0.000000000000000000, 0.000000000000000000 ) ) ;
#25128=FILL_AREA_STYLE_COLOUR ( '', #9812 ) ;
#25133=CARTESIAN_POINT ( 'NONE',  ( 162.5773502691896510, 5.000000000000004441, 0.000000000000000000 ) ) ;
#25135=CARTESIAN_POINT ( 'NONE',  ( 0.7667987217272868028, -15.49901228270247877, 8.125944816629214529 ) ) ;
#25140=LINE ( 'NONE', #13527, #6126 ) ;
#25142=B_SPLINE_CURVE_WITH_KNOTS ( 'NONE', 3,
 ( #14328, #14182, #9377, #9829, #12169, #2460 ),
 .UNSPECIFIED., .F., .F.,
 ( 4, 2, 4 ),
 ( 0.000000000000000000, 0.0009337058470447063543, 0.001867411694089412709 ),
 .UNSPECIFIED. ) ;
#25145=CARTESIAN_POINT ( 'NONE',  ( 140.5000000000000284, -10.99818166789401275, 4.799999999999998934 ) ) ;
#25146=ORIENTED_EDGE ( 'NONE', *, *, #9858, .F. ) ;
#25149=VECTOR ( 'NONE', #1618, 1000.000000000000000 ) ;
#25150=ORIENTED_EDGE ( 'NONE', *, *, #3388, .F. ) ;
#25151=CARTESIAN_POINT ( 'NONE',  ( 158.3437500000000568, -6.000000000000005329, -2.485281374238555774 ) ) ;
#25156=CARTESIAN_POINT ( 'NONE',  ( 0.000000000000000000, 10.00000000000000888, -3.000000000000002665 ) ) ;
#25161=CARTESIAN_POINT ( 'NONE',  ( 140.2370868712064862, -11.61854343560322533, 4.230991509104584658 ) ) ;
#25163=CARTESIAN_POINT ( 'NONE',  ( 159.0000000000000284, -11.07692307692307843, -4.615384615384617639 ) ) ;
#25174=AXIS2_PLACEMENT_3D ( 'NONE', #28530, #7499, #16911 ) ;
#25175=VERTEX_POINT ( 'NONE', #4734 ) ;
#25176=CARTESIAN_POINT ( 'NONE',  ( 135.6636751345948255, 0.000000000000000000, 5.500000000000005329 ) ) ;
#25177=ADVANCED_FACE ( 'NONE', ( #27912 ), #30236, .F. ) ;
#25180=CARTESIAN_POINT ( 'NONE',  ( 139.3273502691896510, -5.000000000000004441, 0.000000000000000000 ) ) ;
#25181=VERTEX_POINT ( 'NONE', #7197 ) ;
#25187=EDGE_CURVE ( 'NONE', #29595, #8771, #4372, .T. ) ;
#25188=DIRECTION ( 'NONE',  ( 0.000000000000000000, 0.000000000000000000, 1.000000000000000000 ) ) ;
#25190=CARTESIAN_POINT ( 'NONE',  ( 159.1428483359083828, -12.00649502811498515, 3.992243735981535480 ) ) ;
#25191=CARTESIAN_POINT ( 'NONE',  ( 143.8125000000000284, 4.242640687119298093, -4.242640687119298093 ) ) ;
#25193=ORIENTED_EDGE ( 'NONE', *, *, #20736, .T. ) ;
#25198=SURFACE_STYLE_FILL_AREA ( #9089 ) ;
#25199=CARTESIAN_POINT ( 'NONE',  ( 135.7574251345947971, -2.278174593051640162, 5.500000000000382805 ) ) ;
#25201=CARTESIAN_POINT ( 'NONE',  ( 135.6737246954143643, -8.728829995092375782, -8.172675940895006264 ) ) ;
#25202=CARTESIAN_POINT ( 'NONE',  ( 148.4851497308104342, -3.535533905932725318, 3.535533905932725318 ) ) ;
#25206=DIRECTION ( 'NONE',  ( 0.000000000000000000, 1.000000000000000000, 0.000000000000000000 ) ) ;
#25214=EDGE_CURVE ( 'NONE', #8542, #3410, #26634, .T. ) ;
#25217=CARTESIAN_POINT ( 'NONE',  ( -15.49999999999999289, -25.00000000000007816, 8.000000000000007105 ) ) ;
#25221=CARTESIAN_POINT ( 'NONE',  ( 148.8750000000000284, 0.000000000000000000, 6.000000000000005329 ) ) ;
#25222=CARTESIAN_POINT ( 'NONE',  ( 160.0053871411751913, -11.56467308583480147, -3.224818504556521415 ) ) ;
#25224=CARTESIAN_POINT ( 'NONE',  ( 137.2500000000000284, -6.000000000000005329, 0.000000000000000000 ) ) ;
#25235=CARTESIAN_POINT ( 'NONE',  ( 139.6518077262924180, -8.798545368671454980, 8.159999962955303943 ) ) ;
#25236=CIRCLE ( 'NONE', #5638, 16.50000000000000355 ) ;
#25238=LINE ( 'NONE', #4210, #15471 ) ;
#25245=CARTESIAN_POINT ( 'NONE',  ( 148.6086002691896510, -2.071067811865468400, -4.999999999999989342 ) ) ;
#25247=CARTESIAN_POINT ( 'NONE',  ( 135.5000000000000284, -9.047800747817580813, -8.000000000000007105 ) ) ;
#25252=CARTESIAN_POINT ( 'NONE',  ( 0.000000000000000000, 0.000000000000000000, 0.000000000000000000 ) ) ;
#25253=VERTEX_POINT ( 'NONE', #10415 ) ;
#25254=CARTESIAN_POINT ( 'NONE',  ( 153.7500000000000284, -6.000000000000005329, 0.000000000000000000 ) ) ;
#25263=DIRECTION ( 'NONE',  ( 0.000000000000000000, 0.000000000000000000, -1.000000000000000000 ) ) ;
#25265=AXIS2_PLACEMENT_3D ( 'NONE', #9108, #18503, #6331 ) ;
#25268=VERTEX_POINT ( 'NONE', #19483 ) ;
#25270=( LENGTH_UNIT ( ) NAMED_UNIT ( * ) SI_UNIT ( .MILLI., .METRE. ) );
#25271=CARTESIAN_POINT ( 'NONE',  ( 140.0466131354633887, -8.931230826727917460, 8.014915759236114212 ) ) ;
#25277=DIRECTION ( 'NONE',  ( 1.000000000000000000, -0.000000000000000000, -0.000000000000000000 ) ) ;
#25281=CARTESIAN_POINT ( 'NONE',  ( 134.9999999981442045, -7.162237350910601208, 8.424967526247618466 ) ) ;
#25284=AXIS2_PLACEMENT_3D ( 'NONE', #11664, #22844, #8551 ) ;
#25286=DIRECTION ( 'NONE',  ( 0.000000000000000000, 0.000000000000000000, -1.000000000000000000 ) ) ;
#25297=CARTESIAN_POINT ( 'NONE',  ( -14.99999999999999289, -54.99999999999990763, -7.500000000000007105 ) ) ;
#25300=CARTESIAN_POINT ( 'NONE',  ( 150.5625000000000568, -4.242640687119298093, 4.242640687119298093 ) ) ;
#25301=EDGE_LOOP ( 'NONE', ( #4375, #772, #18096, #21958 ) ) ;
#25306=CARTESIAN_POINT ( 'NONE',  ( 150.9449251345948539, -5.500000000000012434, 2.278174593052012309 ) ) ;
#25309=CARTESIAN_POINT ( 'NONE',  ( 159.1716635061148679, -11.33697504938031919, 3.989315678507943552 ) ) ;
#25325=CARTESIAN_POINT ( 'NONE',  ( 153.9300748654051745, 2.278174593051810692, -5.500000000000211386 ) ) ;
#25326=ORIENTED_EDGE ( 'NONE', *, *, #28784, .T. ) ;
#25328=CARTESIAN_POINT ( 'NONE',  ( 143.1636751345948255, 0.000000000000000000, 5.500000000000005329 ) ) ;
#25329=STYLED_ITEM ( 'NONE', ( #7727 ), #3859 ) ;
#25330=CARTESIAN_POINT ( 'NONE',  ( 136.4211002691896510, -4.999999999999989342, -2.071067811865468400 ) ) ;
#25331=EDGE_LOOP ( 'NONE', ( #27877, #1856, #4032, #6470 ) ) ;
#25333=CARTESIAN_POINT ( 'NONE',  ( 151.3050748654052313, 5.500000000000012434, 2.278174593052012309 ) ) ;
#25337=( BOUNDED_SURFACE ( )  B_SPLINE_SURFACE ( 3, 2, ( 
 ( #11402, #4445, #30400 ),
 ( #30098, #29939, #4594 ),
 ( #9367, #27777, #146 ),
 ( #23210, #20748, #9063 ),
 ( #4747, #16468, #6753 ),
 ( #25797, #14173, #13713 ),
 ( #4294, #25478, #2156 ),
 ( #23511, #11865, #11558 ),
 ( #2307, #21205, #9527 ),
 ( #1840, #27465, #20903 ) ),
 .UNSPECIFIED., .F., .F., .T. ) 
 B_SPLINE_SURFACE_WITH_KNOTS ( ( 4, 2, 2, 2, 4 ),
 ( 3, 3 ),
 ( 3.141592653589793116, 3.534291735288517255, 3.926990816987241395, 4.319689898685965090, 4.712388980384689674 ),
 ( 0.000000000000000000, 1.000000000000000000 ),
 .UNSPECIFIED. ) 
 GEOMETRIC_REPRESENTATION_ITEM ( )  RATIONAL_B_SPLINE_SURFACE ( (
 ( 1.000000000000000000, 0.7071067811865475727, 1.000000000000000000),
 ( 1.000000000000000000, 0.7066757001360287616, 1.000000000000000000),
 ( 1.000000000000000000, 0.7265518147277496563, 1.000000000000000000),
 ( 1.000000000000000000, 0.7876784249694541717, 1.000000000000000000),
 ( 1.000000000000000000, 0.8282379786091766949, 1.000000000000000000),
 ( 1.000000000000000000, 0.9038128289597016085, 1.000000000000000000),
 ( 1.000000000000000000, 0.9386556746367812343, 1.000000000000000000),
 ( 1.000000000000000000, 0.9867291651255319929, 1.000000000000000000),
 ( 1.000000000000000000, 1.000158598892035622, 1.000000000000000000),
 ( 1.000000000000000000, 1.000000000000000000, 1.000000000000000000) ) ) 
 REPRESENTATION_ITEM ( '' )  SURFACE ( )  );
#25340=ORIENTED_EDGE ( 'NONE', *, *, #9149, .F. ) ;
#25341=ORIENTED_EDGE ( 'NONE', *, *, #20324, .F. ) ;
#25342=CARTESIAN_POINT ( 'NONE',  ( 142.2187500000000284, 2.485281374238555774, -6.000000000000005329 ) ) ;
#25347=DIRECTION ( 'NONE',  ( -0.000000000000000000, -0.000000000000000000, -1.000000000000000000 ) ) ;
#25352=VECTOR ( 'NONE', #6583, 1000.000000000000000 ) ;
#25355=CARTESIAN_POINT ( 'NONE',  ( 141.6413997308104058, 2.071067811865468400, -4.999999999999989342 ) ) ;
#25359=PLANE ( 'NONE',  #26785 ) ;
#25364=CIRCLE ( 'NONE', #9716, 1.000000000000001554 ) ;
#25367=( LENGTH_UNIT ( ) NAMED_UNIT ( * ) SI_UNIT ( .MILLI., .METRE. ) );
#25375=TOROIDAL_SURFACE ( 'NONE', #355, 13.00000000000000178, 1.000000000000000000 ) ;
#25376=CARTESIAN_POINT ( 'NONE',  ( 139.3125000000000284, 4.242640687119298093, -4.242640687119298093 ) ) ;
#25378=DIRECTION ( 'NONE',  ( 1.000000000000000000, -0.000000000000000000, -0.000000000000000000 ) ) ;
#25379=VECTOR ( 'NONE', #10443, 1000.000000000000000 ) ;
#25380=CARTESIAN_POINT ( 'NONE',  ( 139.2187500000000000, 2.485281374238555774, -6.000000000000005329 ) ) ;
#25382=ORIENTED_EDGE ( 'NONE', *, *, #5471, .F. ) ;
#25384=VERTEX_POINT ( 'NONE', #20080 ) ;
#25386=ORIENTED_EDGE ( 'NONE', *, *, #3016, .T. ) ;
#25394=EDGE_CURVE ( 'NONE', #12934, #14826, #10289, .T. ) ;
#25398=CARTESIAN_POINT ( 'NONE',  ( 139.5000000000000000, -9.165151389911695645, 8.000000000000007105 ) ) ;
#25401=CARTESIAN_POINT ( 'NONE',  ( -0.2003331987396294867, -9.399833400630225100, 4.385453238887281557 ) ) ;
#25403=SURFACE_STYLE_USAGE ( .BOTH. , #6679 ) ;
#25405=CARTESIAN_POINT ( 'NONE',  ( 147.2961002691896510, 2.071067811865468400, -4.999999999999989342 ) ) ;
#25408=CARTESIAN_POINT ( 'NONE',  ( 157.6875000000000284, 4.242640687119269671, 4.242640687119298093 ) ) ;
#25413=CARTESIAN_POINT ( 'NONE',  ( 130.0000000000000284, -60.00000000000001421, -3.000000000000002665 ) ) ;
#25414=ORIENTED_EDGE ( 'NONE', *, *, #12706, .F. ) ;
#25415=CARTESIAN_POINT ( 'NONE',  ( 154.2187500000000284, 2.485281374238555774, -6.000000000000005329 ) ) ;
#25421=EDGE_CURVE ( 'NONE', #17415, #765, #22030, .T. ) ;
#25424=ORIENTED_EDGE ( 'NONE', *, *, #23285, .F. ) ;
#25425=DIRECTION ( 'NONE',  ( -1.000000000000000000, 0.000000000000000000, 0.000000000000000000 ) ) ;
#25426=LINE ( 'NONE', #6851, #17480 ) ;
#25428=ORIENTED_EDGE ( 'NONE', *, *, #18645, .F. ) ;
#25438=( NAMED_UNIT ( * ) SI_UNIT ( $, .STERADIAN. ) SOLID_ANGLE_UNIT ( ) );
#25441=CARTESIAN_POINT ( 'NONE',  ( 160.9836002691896226, 4.999999999999989342, -2.071067811865468400 ) ) ;
#25442=CARTESIAN_POINT ( 'NONE',  ( 0.7911096625681925953, -15.46436038730320206, 8.191759848737534710 ) ) ;
#25443=ORIENTED_EDGE ( 'NONE', *, *, #10810, .T. ) ;
#25450=SURFACE_STYLE_USAGE ( .BOTH. , #4262 ) ;
#25454=CARTESIAN_POINT ( 'NONE',  ( 140.5384615384615756, -11.53846153846155254, 4.807692307692318145 ) ) ;
#25455=ORIENTED_EDGE ( 'NONE', *, *, #977, .T. ) ;
#25456=CARTESIAN_POINT ( 'NONE',  ( 149.0625000000000284, -4.242640687119298093, 4.242640687119298093 ) ) ;
#25460=COLOUR_RGB ( '', 0.08235294, 0.09019608, 0.10196078) ;
#25468=CARTESIAN_POINT ( 'NONE',  ( 160.0292075518898116, -11.64910390351806946, 2.883065298126458398 ) ) ;
#25478=CARTESIAN_POINT ( 'NONE',  ( -0.6046674458933889440, -9.395332554106687439, -4.067501169440991049 ) ) ;
#25482=CARTESIAN_POINT ( 'NONE',  ( 135.4072480194323020, -8.806439873276080021, -8.023362806821699778 ) ) ;
#25484=ORIENTED_EDGE ( 'NONE', *, *, #362, .T. ) ;
#25490=AXIS2_PLACEMENT_3D ( 'NONE', #30178, #18535, #27861 ) ;
#25502=CARTESIAN_POINT ( 'NONE',  ( 137.3437500000000568, -6.000000000000005329, -2.485281374238555774 ) ) ;
#25504=ADVANCED_FACE ( 'NONE', ( #29734 ), #3616, .T. ) ;
#25506=FACE_OUTER_BOUND ( 'NONE', #26333, .T. ) ;
#25508=STYLED_ITEM ( 'NONE', ( #3813 ), #27288 ) ;
#25510=DIRECTION ( 'NONE',  ( -1.000000000000000000, 0.000000000000000000, 0.000000000000000000 ) ) ;
#25512=CARTESIAN_POINT ( 'NONE',  ( 135.4056618780774386, -8.496329914198520683, -8.215405480166896979 ) ) ;
#25513=AXIS2_PLACEMENT_3D ( 'NONE', #8910, #11550, #21454 ) ;
#25514=CARTESIAN_POINT ( 'NONE',  ( 146.7976497308104058, 0.000000000000000000, 5.000000000000004441 ) ) ;
#25518=CARTESIAN_POINT ( 'NONE',  ( 156.1949251345949108, 5.500000000000012434, -2.278174593052012309 ) ) ;
#25523=PRODUCT_DEFINITION_CONTEXT ( 'detailed design', #4179, 'design' ) ;
#25525=FILL_AREA_STYLE ('',( #21657 ) ) ;
#25526=VERTEX_POINT ( 'NONE', #28295 ) ;
#25532=ORIENTED_EDGE ( 'NONE', *, *, #3158, .F. ) ;
#25534=CARTESIAN_POINT ( 'NONE',  ( 142.9687500000000284, -2.485281374238585972, 6.000000000000005329 ) ) ;
#25535=CARTESIAN_POINT ( 'NONE',  ( 160.0000000000000284, -12.58710442076092484, -3.130720585662490674 ) ) ;
#25539=CARTESIAN_POINT ( 'NONE',  ( 142.9761751345948255, 3.889087296526011706, 3.889087296526011706 ) ) ;
#25541=CARTESIAN_POINT ( 'NONE',  ( 134.2500000000000284, -6.000000000000005329, 0.000000000000000000 ) ) ;
#25544=EDGE_CURVE ( 'NONE', #10998, #6626, #5829, .T. ) ;
#25545=AXIS2_PLACEMENT_3D ( 'NONE', #23124, #27689, #5258 ) ;
#25551=CARTESIAN_POINT ( 'NONE',  ( 155.0699251345948255, 2.278174593052198382, 5.499999999999826805 ) ) ;
#25553=CARTESIAN_POINT ( 'NONE',  ( 140.2902754521815041, -11.64513772609104159, -4.288736938852963476 ) ) ;
#25564=CIRCLE ( 'NONE', #20189, 1.000000000000000000 ) ;
#25569=CARTESIAN_POINT ( 'NONE',  ( 149.8273502691896510, -5.000000000000004441, 0.000000000000000000 ) ) ;
#25574=STYLED_ITEM ( 'NONE', ( #10500 ), #23989 ) ;
#25575=CARTESIAN_POINT ( 'NONE',  ( 159.9375000000000284, -4.242640687119298093, -4.242640687119298093 ) ) ;
#25581=SURFACE_STYLE_FILL_AREA ( #23146 ) ;
#25582=ORIENTED_EDGE ( 'NONE', *, *, #29874, .F. ) ;
#25583=CARTESIAN_POINT ( 'NONE',  ( 156.9375000000000284, -4.242640687119298093, -4.242640687119298093 ) ) ;
#25585=VECTOR ( 'NONE', #10783, 1000.000000000000000 ) ;
#25588=ORIENTED_EDGE ( 'NONE', *, *, #22890, .F. ) ;
#25589=EDGE_CURVE ( 'NONE', #691, #25181, #23570, .T. ) ;
#25595=ORIENTED_EDGE ( 'NONE', *, *, #21814, .F. ) ;
#25605=AXIS2_PLACEMENT_3D ( 'NONE', #13989, #23328, #9334 ) ;
#25611=CARTESIAN_POINT ( 'NONE',  ( 160.1398502691896510, -3.535533905932752852, 3.535533905932725318 ) ) ;
#25612=FACE_OUTER_BOUND ( 'NONE', #16046, .T. ) ;
#25613=ORIENTED_EDGE ( 'NONE', *, *, #1359, .T. ) ;
#25616=EDGE_CURVE ( 'NONE', #5051, #30356, #28590, .T. ) ;
#25619=CARTESIAN_POINT ( 'NONE',  ( 129.9999999999998010, -90.00000000000001421, 3.000000000000002665 ) ) ;
#25621=CARTESIAN_POINT ( 'NONE',  ( -19.99999999999998224, -54.99999999999990763, -7.500000000000007105 ) ) ;
#25625=ORIENTED_EDGE ( 'NONE', *, *, #22479, .F. ) ;
#25626=ADVANCED_FACE ( 'NONE', ( #23424 ), #16679, .T. ) ;
#25628=EDGE_CURVE ( 'NONE', #14042, #8327, #11306, .T. ) ;
#25630=CARTESIAN_POINT ( 'NONE',  ( 151.5937500000000284, 6.000000000000005329, 2.485281374238585972 ) ) ;
#25640=CARTESIAN_POINT ( 'NONE',  ( 140.0000000000000284, -8.500000000000007105, 8.000000000000007105 ) ) ;
#25644=LINE ( 'NONE', #20590, #29801 ) ;
#25651=EDGE_CURVE ( 'NONE', #27766, #11375, #22268, .T. ) ;
#25654=VECTOR ( 'NONE', #25832, 1000.000000000000000 ) ;
#25655=VERTEX_POINT ( 'NONE', #200 ) ;
#25661=MECHANICAL_DESIGN_GEOMETRIC_PRESENTATION_REPRESENTATION('',(#28575),#16855);
#25666=CARTESIAN_POINT ( 'NONE',  ( 136.0312500000000000, -2.485281374238555774, -6.000000000000005329 ) ) ;
#25674=AXIS2_PLACEMENT_3D ( 'NONE', #4714, #16141, #25286 ) ;
#25675=CARTESIAN_POINT ( 'NONE',  ( 142.3913997308104058, -2.071067811865468400, 4.999999999999989342 ) ) ;
#25682=DIRECTION ( 'NONE',  ( 0.000000000000000000, 0.000000000000000000, 1.000000000000000000 ) ) ;
#25683=CARTESIAN_POINT ( 'NONE',  ( 0.000000000000000000, -9.500000000000008882, 5.000000000000004441 ) ) ;
#25688=EDGE_CURVE ( 'NONE', #10874, #2429, #1405, .T. ) ;
#25692=CARTESIAN_POINT ( 'NONE',  ( 141.6562500000000284, -6.000000000000005329, 2.485281374238556218 ) ) ;
#25695=CARTESIAN_POINT ( 'NONE',  ( 134.1562500000000568, -6.000000000000005329, 2.485281374238555774 ) ) ;
#25696=FACE_OUTER_BOUND ( 'NONE', #9952, .T. ) ;
#25699=ORIENTED_EDGE ( 'NONE', *, *, #29732, .F. ) ;
#25703=CARTESIAN_POINT ( 'NONE',  ( 160.0000000000000284, -12.64911064067353408, -3.000000000000002665 ) ) ;
#25706=CARTESIAN_POINT ( 'NONE',  ( 154.8824251345948255, 5.500000000000012434, 2.278174593052012309 ) ) ;
#25708=CARTESIAN_POINT ( 'NONE',  ( 0.000000000000000000, 9.000000000000007105, -5.000000000000004441 ) ) ;
#25717=AXIS2_PLACEMENT_3D ( 'NONE', #5790, #26681, #1922 ) ;
#25719=CARTESIAN_POINT ( 'NONE',  ( 154.5863248654052313, 0.000000000000000000, 5.500000000000005329 ) ) ;
#25724=SURFACE_STYLE_FILL_AREA ( #2383 ) ;
#25725=CARTESIAN_POINT ( 'NONE',  ( 149.5461002691896510, -2.071067811865468400, 4.999999999999989342 ) ) ;
#25728=CARTESIAN_POINT ( 'NONE',  ( 156.0937500000000284, 6.000000000000005329, 2.485281374238585972 ) ) ;
#25735=CARTESIAN_POINT ( 'NONE',  ( 148.6875000000000284, 4.242640687119269671, 4.242640687119298093 ) ) ;
#25741=EDGE_LOOP ( 'NONE', ( #12694, #16613, #13200, #30117 ) ) ;
#25746=CARTESIAN_POINT ( 'NONE',  ( 154.7663997308104342, -4.999999999999989342, -2.071067811865468400 ) ) ;
#25753=LINE ( 'NONE', #22851, #3689 ) ;
#25756=CIRCLE ( 'NONE', #19874, 1.000000000000000888 ) ;
#25759=CARTESIAN_POINT ( 'NONE',  ( 144.6636751345948255, 0.000000000000000000, 5.500000000000005329 ) ) ;
#25762=CARTESIAN_POINT ( 'NONE',  ( 116.0000000000000142, 0.000000000000000000, 0.000000000000000000 ) ) ;
#25763=CARTESIAN_POINT ( 'NONE',  ( 160.4211002691896510, -4.999999999999989342, -2.071067811865468400 ) ) ;
#25764=CARTESIAN_POINT ( 'NONE',  ( 0.8492726096241208777, -15.39617198623466976, 8.319207606560656387 ) ) ;
#25775=CARTESIAN_POINT ( 'NONE',  ( -19.49999999999998224, -24.99999999999999289, -8.000000000000007105 ) ) ;
#25776=ORIENTED_EDGE ( 'NONE', *, *, #28436, .T. ) ;
#25777=LINE ( 'NONE', #4724, #19406 ) ;
#25778=ORIENTED_EDGE ( 'NONE', *, *, #4768, .F. ) ;
#25779=CARTESIAN_POINT ( 'NONE',  ( 152.7187500000000284, 2.485281374238555774, -6.000000000000005329 ) ) ;
#25781=CIRCLE ( 'NONE', #4675, 14.49999999999998579 ) ;
#25789=FILL_AREA_STYLE_COLOUR ( '', #8645 ) ;
#25797=CARTESIAN_POINT ( 'NONE',  ( -0.3854532388872504156, -9.307273380556397413, -4.200333198739659935 ) ) ;
#25805=CARTESIAN_POINT ( 'NONE',  ( -0.07769256095283472163, -15.23231281889969146, 7.500000000000007105 ) ) ;
#25806=CYLINDRICAL_SURFACE ( 'NONE', #23903, 0.5000000000000004441 ) ;
#25808=ORIENTED_EDGE ( 'NONE', *, *, #29523, .T. ) ;
#25819=CARTESIAN_POINT ( 'NONE',  ( 137.4375000000000568, -4.242640687119298093, -4.242640687119298093 ) ) ;
#25820=CIRCLE ( 'NONE', #9649, 0.5000000000000004441 ) ;
#25825=CARTESIAN_POINT ( 'NONE',  ( 136.0000000000000284, -9.165151389911695645, -8.500000000000007105 ) ) ;
#25829=CARTESIAN_POINT ( 'NONE',  ( 146.8913997308104626, -2.071067811865468400, 4.999999999999989342 ) ) ;
#25830=DIRECTION ( 'NONE',  ( 0.000000000000000000, 0.000000000000000000, -1.000000000000000000 ) ) ;
#25831=CARTESIAN_POINT ( 'NONE',  ( -4.999999999999886313, -69.50000000000001421, 7.500000000000007105 ) ) ;
#25832=DIRECTION ( 'NONE',  ( 1.000000000000000000, -0.000000000000000000, -0.000000000000000000 ) ) ;
#25837=PRESENTATION_STYLE_ASSIGNMENT (( #16512 ) ) ;
#25840=ORIENTED_EDGE ( 'NONE', *, *, #13949, .T. ) ;
#25842=CARTESIAN_POINT ( 'NONE',  ( -9.999999999999994671, -71.00000000000002842, 4.000000000000003553 ) ) ;
#25843=VERTEX_POINT ( 'NONE', #3239 ) ;
#25845=CARTESIAN_POINT ( 'NONE',  ( 141.3750000000000284, 0.000000000000000000, 6.000000000000005329 ) ) ;
#25848=CARTESIAN_POINT ( 'NONE',  ( 159.4538997308104058, -2.071067811865468400, -4.999999999999989342 ) ) ;
#25851=AXIS2_PLACEMENT_3D ( 'NONE', #14380, #2949, #7276 ) ;
#25853=ORIENTED_EDGE ( 'NONE', *, *, #12260, .T. ) ;
#25858=ADVANCED_FACE ( 'NONE', ( #11112 ), #16051, .F. ) ;
#25865=( NAMED_UNIT ( * ) SI_UNIT ( $, .STERADIAN. ) SOLID_ANGLE_UNIT ( ) );
#25868=CARTESIAN_POINT ( 'NONE',  ( 140.0510979238436278, -8.941207700098154021, 8.003589737453340902 ) ) ;
#25874=CARTESIAN_POINT ( 'NONE',  ( 155.8125000000000284, 4.242640687119298093, -4.242640687119298093 ) ) ;
#25875=( NAMED_UNIT ( * ) SI_UNIT ( $, .STERADIAN. ) SOLID_ANGLE_UNIT ( ) );
#25878=VERTEX_POINT ( 'NONE', #22924 ) ;
#25879=CARTESIAN_POINT ( 'NONE',  ( 152.9062500000000000, 6.000000000000005329, -2.485281374238555774 ) ) ;
#25881=AXIS2_PLACEMENT_3D ( 'NONE', #880, #10128, #21944 ) ;
#25883=VERTEX_POINT ( 'NONE', #16199 ) ;
#25884=VECTOR ( 'NONE', #27875, 1000.000000000000000 ) ;
#25889=COLOUR_RGB ( '', 0.09019608, 0.27058824, 0.51372549) ;
#25890=AXIS2_PLACEMENT_3D ( 'NONE', #19798, #29144, #26833 ) ;
#25892=ADVANCED_FACE ( 'NONE', ( #1867 ), #29818, .F. ) ;
#25894=CARTESIAN_POINT ( 'NONE',  ( 156.5476497308104342, 0.000000000000000000, -5.000000000000004441 ) ) ;
#25899=AXIS2_PLACEMENT_3D ( 'NONE', #1391, #10801, #20445 ) ;
#25903=B_SPLINE_CURVE_WITH_KNOTS ( 'NONE', 3,
 ( #3777, #1478, #22695, #13658, #8712, #29735, #18251, #27418, #11348, #15819 ),
 .UNSPECIFIED., .F., .F.,
 ( 4, 2, 2, 2, 4 ),
 ( 0.000000000000000000, 0.0004454033597584232786, 0.0008908067195168465572, 0.001336210079275269944, 0.001781613439033693114 ),
 .UNSPECIFIED. ) ;
#25904=CARTESIAN_POINT ( 'NONE',  ( 0.000000000000000000, 0.000000000000000000, 0.000000000000000000 ) ) ;
#25909=CARTESIAN_POINT ( 'NONE',  ( 156.5773502691896510, 5.000000000000004441, 0.000000000000000000 ) ) ;
#25910=LINE ( 'NONE', #4858, #21902 ) ;
#25911=VERTEX_POINT ( 'NONE', #27804 ) ;
#25912=UNCERTAINTY_MEASURE_WITH_UNIT (LENGTH_MEASURE( 1.000000000000000082E-05 ), #22010, 'distance_accuracy_value', 'NONE');
#25917=EDGE_LOOP ( 'NONE', ( #3810, #30186, #19229, #24404 ) ) ;
#25919=CARTESIAN_POINT ( 'NONE',  ( -0.07852715771744070428, -14.93815133716600307, -8.093175384816596818 ) ) ;
#25921=ADVANCED_FACE ( 'NONE', ( #20779 ), #6629, .T. ) ;
#25922=DIRECTION ( 'NONE',  ( 1.000000000000000000, 0.000000000000000000, 0.000000000000000000 ) ) ;
#25924=CARTESIAN_POINT ( 'NONE',  ( 149.5312500000000284, -2.485281374238555774, -6.000000000000005329 ) ) ;
#25930=SURFACE_SIDE_STYLE ('',( #6737 ) ) ;
#25933=CARTESIAN_POINT ( 'NONE',  ( 133.1101497308104342, 3.535533905932725318, 3.535533905932725318 ) ) ;
#25936=FILL_AREA_STYLE_COLOUR ( '', #2045 ) ;
#25941=FILL_AREA_STYLE_COLOUR ( '', #10319 ) ;
#25942=CARTESIAN_POINT ( 'NONE',  ( 136.0000000000000284, 0.000000000000000000, 0.000000000000000000 ) ) ;
#25943=UNCERTAINTY_MEASURE_WITH_UNIT (LENGTH_MEASURE( 1.000000000000000082E-05 ), #4123, 'distance_accuracy_value', 'NONE');
#25945=CARTESIAN_POINT ( 'NONE',  ( 134.9999999999992895, -7.147597648790188885, -8.399649850026122522 ) ) ;
#25947=EDGE_LOOP ( 'NONE', ( #9348, #333, #8354, #6234, #9256, #13881, #20330, #18848, #24972, #29063, #24250, #5910, #14270, #18210, #15539, #414, #6490, #7380, #18624, #28441, #19103, #23200, #5428, #4261, #14376, #6537, #14839, #7835, #11181, #17598, #13160, #25193, #19690, #19825, #23488, #26802, #2421, #17947, #4612 ) ) ;
#25949=CARTESIAN_POINT ( 'NONE',  ( 0.7669223171414829565, -15.58766199952932396, -7.954545454545463912 ) ) ;
#25951=ORIENTED_EDGE ( 'NONE', *, *, #18288, .F. ) ;
#25952=DIRECTION ( 'NONE',  ( 0.000000000000000000, 1.000000000000000000, 0.000000000000000000 ) ) ;
#25955=AXIS2_PLACEMENT_3D ( 'NONE', #7711, #28444, #4656 ) ;
#25956=CARTESIAN_POINT ( 'NONE',  ( -4.999999999999990230, -55.00000000000002132, 8.000000000000007105 ) ) ;
#25958=( GEOMETRIC_REPRESENTATION_CONTEXT ( 3 ) GLOBAL_UNCERTAINTY_ASSIGNED_CONTEXT ( ( #17777 ) ) GLOBAL_UNIT_ASSIGNED_CONTEXT ( ( #11908, #14359, #631 ) ) REPRESENTATION_CONTEXT ( 'NONE', 'WORKASPACE' ) );
#25960=ORIENTED_EDGE ( 'NONE', *, *, #15046, .F. ) ;
#25961=VERTEX_POINT ( 'NONE', #8632 ) ;
#25963=CARTESIAN_POINT ( 'NONE',  ( 134.7187500000000284, 2.485281374238555774, -6.000000000000005329 ) ) ;
#25966=VERTEX_POINT ( 'NONE', #2767 ) ;
#25968=CARTESIAN_POINT ( 'NONE',  ( 116.0000000000000142, 0.000000000000000000, 0.000000000000000000 ) ) ;
#25976=CARTESIAN_POINT ( 'NONE',  ( 139.2976497308104058, 0.000000000000000000, 5.000000000000004441 ) ) ;
#25979=CARTESIAN_POINT ( 'NONE',  ( -19.49999999999998224, -54.99999999999992184, 7.500000000000007105 ) ) ;
#25985=ORIENTED_EDGE ( 'NONE', *, *, #26398, .T. ) ;
#25990=ORIENTED_EDGE ( 'NONE', *, *, #9598, .F. ) ;
#25992=CARTESIAN_POINT ( 'NONE',  ( 138.8437500000000568, -6.000000000000005329, -2.485281374238556218 ) ) ;
#25993=ADVANCED_FACE ( 'NONE', ( #12195 ), #2623, .T. ) ;
#25994=CARTESIAN_POINT ( 'NONE',  ( 135.1875000000000568, 4.242640687119269671, 4.242640687119298093 ) ) ;
#25995=AXIS2_PLACEMENT_3D ( 'NONE', #23315, #657, #2259 ) ;
#25996=EDGE_CURVE ( 'NONE', #11247, #14299, #16702, .T. ) ;
#25998=ADVANCED_FACE ( 'NONE', ( #9554 ), #12179, .T. ) ;
#25999=EDGE_LOOP ( 'NONE', ( #14763, #28292, #15216, #11076 ) ) ;
#26000=ORIENTED_EDGE ( 'NONE', *, *, #6659, .T. ) ;
#26003=CARTESIAN_POINT ( 'NONE',  ( 159.8150495723242557, -12.30910372856451396, -3.593108990249125778 ) ) ;
#26006=CARTESIAN_POINT ( 'NONE',  ( 154.6011751345948539, 3.889087296526011706, -3.889087296526011706 ) ) ;
#26008=DIRECTION ( 'NONE',  ( 0.000000000000000000, 0.000000000000000000, -1.000000000000000000 ) ) ;
#26009=DIRECTION ( 'NONE',  ( 1.000000000000000000, -0.000000000000000000, -0.000000000000000000 ) ) ;
#26011=CARTESIAN_POINT ( 'NONE',  ( 140.3936200311551374, -9.249647488735854850, 7.646135955868133216 ) ) ;
#26014=AXIS2_PLACEMENT_3D ( 'NONE', #19377, #7524, #7673 ) ;
#26016=DIRECTION ( 'NONE',  ( 1.000000000000000000, -0.000000000000000000, -0.000000000000000000 ) ) ;
#26018=CARTESIAN_POINT ( 'NONE',  ( 139.6831941873303720, -9.225388190634568275, 7.967326043633793375 ) ) ;
#26019=CARTESIAN_POINT ( 'NONE',  ( 146.1711002691896226, 4.999999999999989342, 2.071067811865468400 ) ) ;
#26021=CARTESIAN_POINT ( 'NONE',  ( 160.7812500000000284, 2.485281374238585972, 6.000000000000005329 ) ) ;
#26024=DIRECTION ( 'NONE',  ( 0.000000000000000000, 0.000000000000000000, -1.000000000000000000 ) ) ;
#26029=CARTESIAN_POINT ( 'NONE',  ( 153.0937500000000284, 6.000000000000005329, 2.485281374238585972 ) ) ;
#26030=DIRECTION ( 'NONE',  ( -0.000000000000000000, -0.000000000000000000, -1.000000000000000000 ) ) ;
#26032=FILL_AREA_STYLE_COLOUR ( '', #30300 ) ;
#26034=LINE ( 'NONE', #827, #27056 ) ;
#26036=EDGE_LOOP ( 'NONE', ( #520, #21042, #10920, #28331 ) ) ;
#26044=AXIS2_PLACEMENT_3D ( 'NONE', #22259, #1349, #26545 ) ;
#26045=CARTESIAN_POINT ( 'NONE',  ( 155.2351497308104058, 3.535533905932725318, -3.535533905932725318 ) ) ;
#26046=DIRECTION ( 'NONE',  ( 0.000000000000000000, 0.8570991287109669399, -0.5151515151515151381 ) ) ;
#26055=FACE_OUTER_BOUND ( 'NONE', #11698, .T. ) ;
#26057=CARTESIAN_POINT ( 'NONE',  ( 155.5461002691896510, -2.071067811865468400, 4.999999999999989342 ) ) ;
#26059=ORIENTED_EDGE ( 'NONE', *, *, #25544, .F. ) ;
#26062=AXIS2_PLACEMENT_3D ( 'NONE', #25831, #18491, #18343 ) ;
#26068=CARTESIAN_POINT ( 'NONE',  ( -0.06536716197634070968, -14.68492711179653121, -8.235952467655341280 ) ) ;
#26074=EDGE_LOOP ( 'NONE', ( #18936, #24462, #3764, #26112 ) ) ;
#26082=AXIS2_PLACEMENT_3D ( 'NONE', #707, #12569, #19746 ) ;
#26083=CARTESIAN_POINT ( 'NONE',  ( -8.673617379884035472E-16, -9.500000000000008882, 4.414213562373099364 ) ) ;
#26084=AXIS2_PLACEMENT_3D ( 'NONE', #26229, #5181, #2883 ) ;
#26085=EDGE_LOOP ( 'NONE', ( #22192, #14471, #6582, #31 ) ) ;
#26090=CARTESIAN_POINT ( 'NONE',  ( 152.3363248654052029, 0.000000000000000000, -5.500000000000005329 ) ) ;
#26103=ORIENTED_EDGE ( 'NONE', *, *, #29167, .F. ) ;
#26106=ORIENTED_EDGE ( 'NONE', *, *, #362, .F. ) ;
#26108=ORIENTED_EDGE ( 'NONE', *, *, #18120, .F. ) ;
#26111=CARTESIAN_POINT ( 'NONE',  ( 134.4375000000000568, -4.242640687119298093, -4.242640687119298093 ) ) ;
#26112=ORIENTED_EDGE ( 'NONE', *, *, #2216, .F. ) ;
#26121=CARTESIAN_POINT ( 'NONE',  ( -0.7071067811865487940, -9.585786437626913070, 4.000000000000004441 ) ) ;
#26122=CARTESIAN_POINT ( 'NONE',  ( 136.4851497308104058, -3.535533905932725318, 3.535533905932725318 ) ) ;
#26129=DIRECTION ( 'NONE',  ( -0.000000000000000000, -0.000000000000000000, -1.000000000000000000 ) ) ;
#26130=ORIENTED_EDGE ( 'NONE', *, *, #12067, .T. ) ;
#26134=EDGE_CURVE ( 'NONE', #6918, #4026, #27934, .T. ) ;
#26140=CARTESIAN_POINT ( 'NONE',  ( 134.7187500000000284, 2.485281374238555774, -6.000000000000005329 ) ) ;
#26147=DIRECTION ( 'NONE',  ( 1.000000000000000000, -0.000000000000000000, -0.000000000000000000 ) ) ;
#26153=CARTESIAN_POINT ( 'NONE',  ( 140.5000000000000284, -10.99818166789401275, 4.799999999999998934 ) ) ;
#26158=CARTESIAN_POINT ( 'NONE',  ( -4.999999999999920952, -65.50000000000001421, 8.000000000000007105 ) ) ;
#26160=CARTESIAN_POINT ( 'NONE',  ( 145.4925748654052029, 2.278174593052012309, 5.500000000000012434 ) ) ;
#26161=EDGE_CURVE ( 'NONE', #4004, #1664, #30409, .T. ) ;
#26163=ADVANCED_FACE ( 'NONE', ( #19964 ), #1723, .T. ) ;
#26165=CARTESIAN_POINT ( 'NONE',  ( 144.9523502691896510, 0.000000000000000000, 5.000000000000004441 ) ) ;
#26168=CARTESIAN_POINT ( 'NONE',  ( 152.9062500000000568, 6.000000000000005329, -2.485281374238556218 ) ) ;
#26170=LINE ( 'NONE', #11646, #7220 ) ;
#26174=CARTESIAN_POINT ( 'NONE',  ( 152.2500000000000284, -6.000000000000005329, 0.000000000000000000 ) ) ;
#26176=( LENGTH_UNIT ( ) NAMED_UNIT ( * ) SI_UNIT ( .MILLI., .METRE. ) );
#26181=ORIENTED_EDGE ( 'NONE', *, *, #13913, .T. ) ;
#26184=EDGE_LOOP ( 'NONE', ( #10755, #24000, #16600, #17266, #17645 ) ) ;
#26187=CARTESIAN_POINT ( 'NONE',  ( 129.9999999999998010, -90.00000000000001421, 4.000000000000003553 ) ) ;
#26189=( NAMED_UNIT ( * ) SI_UNIT ( $, .STERADIAN. ) SOLID_ANGLE_UNIT ( ) );
#26190=CARTESIAN_POINT ( 'NONE',  ( 140.0000000000000284, -11.48520880827722124, 4.868161254798543780 ) ) ;
#26197=EDGE_CURVE ( 'NONE', #4156, #234, #23062, .T. ) ;
#26200=CARTESIAN_POINT ( 'NONE',  ( 156.4836002691896795, 4.999999999999989342, -2.071067811865468400 ) ) ;
#26206=VERTEX_POINT ( 'NONE', #29781 ) ;
#26207=DIRECTION ( 'NONE',  ( 0.000000000000000000, 0.9730085108210397848, -0.2307692307692307265 ) ) ;
#26210=ORIENTED_EDGE ( 'NONE', *, *, #28278, .T. ) ;
#26211=CARTESIAN_POINT ( 'NONE',  ( 145.5937500000000284, 6.000000000000005329, 2.485281374238585972 ) ) ;
#26215=UNCERTAINTY_MEASURE_WITH_UNIT (LENGTH_MEASURE( 1.000000000000000082E-05 ), #8737, 'distance_accuracy_value', 'NONE');
#26220=CARTESIAN_POINT ( 'NONE',  ( 132.2663997308104342, -4.999999999999989342, -2.071067811865468400 ) ) ;
#26221=TOROIDAL_SURFACE ( 'NONE', #20858, 14.49999999999999822, 0.5000000000000000000 ) ;
#26222=ADVANCED_FACE ( 'NONE', ( #13547 ), #547, .T. ) ;
#26225=CARTESIAN_POINT ( 'NONE',  ( 0.8492607147730748540, -15.39618690451816008, -8.319180134514111202 ) ) ;
#26229=CARTESIAN_POINT ( 'NONE',  ( -19.99999999999998224, -54.99999999999990763, 8.000000000000007105 ) ) ;
#26235=DIRECTION ( 'NONE',  ( -1.000000000000000000, 0.000000000000000000, 0.000000000000000000 ) ) ;
#26243=B_SPLINE_CURVE_WITH_KNOTS ( 'NONE', 3,
 ( #29893, #27573, #6553, #15973, #25271, #13666, #23008, #11356 ),
 .UNSPECIFIED., .F., .F.,
 ( 4, 2, 2, 4 ),
 ( 0.000000000000000000, 0.0008823129044422798641, 0.001323469356663417628, 0.001764625808884555391 ),
 .UNSPECIFIED. ) ;
#26248=MECHANICAL_DESIGN_GEOMETRIC_PRESENTATION_REPRESENTATION('',(#6122),#3316);
#26255=CARTESIAN_POINT ( 'NONE',  ( 132.8437500000000284, -6.000000000000005329, -2.485281374238555774 ) ) ;
#26256=CARTESIAN_POINT ( 'NONE',  ( 132.9523502691896510, 0.000000000000000000, 5.000000000000004441 ) ) ;
#26257=VERTEX_POINT ( 'NONE', #5623 ) ;
#26258=CARTESIAN_POINT ( 'NONE',  ( 139.4136751345948539, 0.000000000000000000, -5.500000000000005329 ) ) ;
#26267=CARTESIAN_POINT ( 'NONE',  ( 149.8199251345948824, -2.278174593051981223, -5.500000000000041744 ) ) ;
#26269=CARTESIAN_POINT ( 'NONE',  ( 138.3601497308104058, -3.535533905932725318, -3.535533905932725318 ) ) ;
#26270=CARTESIAN_POINT ( 'NONE',  ( 152.3363248654052029, 0.000000000000000000, -5.500000000000005329 ) ) ;
#26271=AXIS2_PLACEMENT_3D ( 'NONE', #25252, #6530, #1928 ) ;
#26285=CARTESIAN_POINT ( 'NONE',  ( 136.6875000000000284, 4.242640687119269671, 4.242640687119298093 ) ) ;
#26288=( NAMED_UNIT ( * ) SI_UNIT ( $, .STERADIAN. ) SOLID_ANGLE_UNIT ( ) );
#26289=DIRECTION ( 'NONE',  ( -0.000000000000000000, -0.000000000000000000, -1.000000000000000000 ) ) ;
#26295=PLANE ( 'NONE',  #20455 ) ;
#26299=EDGE_CURVE ( 'NONE', #17999, #27945, #29120, .T. ) ;
#26300=DIRECTION ( 'NONE',  ( 1.000000000000000000, 6.938893903907221278E-15, 0.000000000000000000 ) ) ;
#26301=FACE_OUTER_BOUND ( 'NONE', #7215, .T. ) ;
#26302=CARTESIAN_POINT ( 'NONE',  ( 1.000000000000000888, 2.143131898507868643E-15, -17.50000000000000355 ) ) ;
#26303=DIRECTION ( 'NONE',  ( -0.000000000000000000, 1.000000000000000000, -0.000000000000000000 ) ) ;
#26306=CARTESIAN_POINT ( 'NONE',  ( -4.999999999999886313, -10.00000000000000888, 8.000000000000007105 ) ) ;
#26312=SURFACE_STYLE_USAGE ( .BOTH. , #22176 ) ;
#26313=CARTESIAN_POINT ( 'NONE',  ( 154.0312500000000284, -2.485281374238556218, -6.000000000000005329 ) ) ;
#26314=CARTESIAN_POINT ( 'NONE',  ( 135.0000000000000000, -8.132390304760285460, -7.784889480266582673 ) ) ;
#26319=CARTESIAN_POINT ( 'NONE',  ( 148.2187500000000568, 2.485281374238555774, -6.000000000000005329 ) ) ;
#26321=UNCERTAINTY_MEASURE_WITH_UNIT (LENGTH_MEASURE( 1.000000000000000082E-05 ), #12459, 'distance_accuracy_value', 'NONE');
#26322=( BOUNDED_CURVE ( )  B_SPLINE_CURVE ( 2, ( #27024, #19973, #8129, #15406, #29327, #18011, #8453, #20137, #18153 ),
 .UNSPECIFIED., .F., .T. ) 
 B_SPLINE_CURVE_WITH_KNOTS ( ( 3, 2, 2, 2, 3 ),
 ( 0.5124999999999990674, 0.5187499999999993783, 0.5249999999999995781, 0.5312499999999997780, 0.5374999999999999778 ),
 .UNSPECIFIED. ) 
 CURVE ( )  GEOMETRIC_REPRESENTATION_ITEM ( )  RATIONAL_B_SPLINE_CURVE ( ( 1.000000000000010880, 0.9238795325112759693, 1.000000000000000000, 0.9238795325112867385, 1.000000000000000000, 0.9238795325112867385, 1.000000000000000000, 0.9238795325112867385, 1.000000000000000000 ) ) 
 REPRESENTATION_ITEM ( '' )  );
#26333=EDGE_LOOP ( 'NONE', ( #20688, #15970, #25990, #2868 ) ) ;
#26335=FILL_AREA_STYLE_COLOUR ( '', #14756 ) ;
#26338=CARTESIAN_POINT ( 'NONE',  ( 140.5126264503616085, -11.05212133306724276, 4.674908800638664097 ) ) ;
#26342=LINE ( 'NONE', #7901, #28228 ) ;
#26349=CARTESIAN_POINT ( 'NONE',  ( 157.1398502691896510, -3.535533905932752852, 3.535533905932725318 ) ) ;
#26353=CARTESIAN_POINT ( 'NONE',  ( -1.000000000000000888, 9.000000000000007105, -3.000000000000002665 ) ) ;
#26354=( NAMED_UNIT ( * ) SI_UNIT ( $, .STERADIAN. ) SOLID_ANGLE_UNIT ( ) );
#26356=ORIENTED_EDGE ( 'NONE', *, *, #30191, .F. ) ;
#26357=CARTESIAN_POINT ( 'NONE',  ( 135.0000000000000284, -8.798545334315205579, 8.160000000000000142 ) ) ;
#26358=FACE_OUTER_BOUND ( 'NONE', #7039, .T. ) ;
#26361=ADVANCED_FACE ( 'NONE', ( #12302 ), #19345, .T. ) ;
#26362=ORIENTED_EDGE ( 'NONE', *, *, #9953, .T. ) ;
#26363=TOROIDAL_SURFACE ( 'NONE', #358, 11.00000000000000355, 1.000000000000000000 ) ;
#26365=CARTESIAN_POINT ( 'NONE',  ( 147.4687500000000853, -2.485281374238585972, 6.000000000000005329 ) ) ;
#26373=FACE_OUTER_BOUND ( 'NONE', #15803, .T. ) ;
#26374=FILL_AREA_STYLE ('',( #25789 ) ) ;
#26381=MECHANICAL_DESIGN_GEOMETRIC_PRESENTATION_REPRESENTATION('',(#22484),#8219);
#26383=CARTESIAN_POINT ( 'NONE',  ( -0.07769256095284393648, -15.23231281889969679, 7.500000000000007105 ) ) ;
#26390=DIRECTION ( 'NONE',  ( 1.000000000000000000, 0.000000000000000000, 0.000000000000000000 ) ) ;
#26393=CARTESIAN_POINT ( 'NONE',  ( 8.673617379884035472E-16, -15.46112173798350753, 5.976438085239231590 ) ) ;
#26396=( NAMED_UNIT ( * ) SI_UNIT ( $, .STERADIAN. ) SOLID_ANGLE_UNIT ( ) );
#26398=EDGE_CURVE ( 'NONE', #11694, #8247, #3927, .T. ) ;
#26405=CARTESIAN_POINT ( 'NONE',  ( 160.3125000000000284, 4.242640687119298093, -4.242640687119298093 ) ) ;
#26406=ORIENTED_EDGE ( 'NONE', *, *, #12210, .T. ) ;
#26407=AXIS2_PLACEMENT_3D ( 'NONE', #28569, #14209, #16948 ) ;
#26410=CARTESIAN_POINT ( 'NONE',  ( 135.8257310488615417, -9.165151389911700974, -8.000000000000007105 ) ) ;
#26411=CARTESIAN_POINT ( 'NONE',  ( 144.6636751345948255, 0.000000000000000000, 5.500000000000005329 ) ) ;
#26414=CARTESIAN_POINT ( 'NONE',  ( 0.1991271335306928347, -15.94713376385915637, -7.214644098438425246 ) ) ;
#26415=LINE ( 'NONE', #21829, #18647 ) ;
#26416=CARTESIAN_POINT ( 'NONE',  ( 137.3288997308104342, 4.999999999999989342, -2.071067811865468400 ) ) ;
#26417=LINE ( 'NONE', #24122, #1548 ) ;
#26419=SURFACE_STYLE_USAGE ( .BOTH. , #14926 ) ;
#26422=( BOUNDED_CURVE ( )  B_SPLINE_CURVE ( 2, ( #12452, #21942, #15035, #19778, #5480, #10427, #29126, #3325, #26090 ),
 .UNSPECIFIED., .F., .T. ) 
 B_SPLINE_CURVE_WITH_KNOTS ( ( 3, 2, 2, 2, 3 ),
 ( 0.2874999999999998113, 0.2937500000000000666, 0.3000000000000002665, 0.3062500000000005773, 0.3125000000000007772 ),
 .UNSPECIFIED. ) 
 CURVE ( )  GEOMETRIC_REPRESENTATION_ITEM ( )  RATIONAL_B_SPLINE_CURVE ( ( 1.000000000000001998, 0.9238795325112847401, 1.000000000000000000, 0.9238795325112867385, 1.000000000000000000, 0.9238795325112867385, 1.000000000000000000, 0.9238795325112773016, 1.000000000000009548 ) ) 
 REPRESENTATION_ITEM ( '' )  );
#26427=CARTESIAN_POINT ( 'NONE',  ( 1.000000000000000888, -15.50000000000001421, -5.656854249492387687 ) ) ;
#26433=CARTESIAN_POINT ( 'NONE',  ( 135.0000000000000284, 6.000000000000005329, 0.000000000000000000 ) ) ;
#26434=EDGE_CURVE ( 'NONE', #1653, #476, #24679, .T. ) ;
#26437=ORIENTED_EDGE ( 'NONE', *, *, #16303, .F. ) ;
#26449=CARTESIAN_POINT ( 'NONE',  ( 160.0000000000000284, -59.99999999999980105, 3.000000000000002665 ) ) ;
#26451=PRESENTATION_STYLE_ASSIGNMENT (( #14813 ) ) ;
#26455=CARTESIAN_POINT ( 'NONE',  ( 140.0304953857124701, -9.269783219788546802, 7.622864659627890838 ) ) ;
#26457=FILL_AREA_STYLE_COLOUR ( '', #21899 ) ;
#26460=CARTESIAN_POINT ( 'NONE',  ( 144.5773502691896510, 5.000000000000004441, 0.000000000000000000 ) ) ;
#26461=CARTESIAN_POINT ( 'NONE',  ( 152.5312500000000568, -2.485281374238556218, -6.000000000000005329 ) ) ;
#26465=ORIENTED_EDGE ( 'NONE', *, *, #17146, .F. ) ;
#26466=CARTESIAN_POINT ( 'NONE',  ( 145.3125000000000284, 4.242640687119298093, -4.242640687119298093 ) ) ;
#26467=AXIS2_PLACEMENT_3D ( 'NONE', #1529, #11085, #25022 ) ;
#26469=CARTESIAN_POINT ( 'NONE',  ( 135.0448603013149977, 1.007610841837577542, 5.499999999999951150 ) ) ;
#26472=ORIENTED_EDGE ( 'NONE', *, *, #10649, .T. ) ;
#26475=( NAMED_UNIT ( * ) PLANE_ANGLE_UNIT ( ) SI_UNIT ( $, .RADIAN. ) );
#26477=PRESENTATION_STYLE_ASSIGNMENT (( #28934 ) ) ;
#26478=CARTESIAN_POINT ( 'NONE',  ( 140.5384615384615756, -11.07692307692309264, 4.615384615384626521 ) ) ;
#26487=PLANE ( 'NONE',  #28959 ) ;
#26489=CARTESIAN_POINT ( 'NONE',  ( 135.3675748654052313, -5.500000000000012434, 2.278174593052012309 ) ) ;
#26490=CARTESIAN_POINT ( 'NONE',  ( 157.3273502691896510, -5.000000000000004441, 0.000000000000000000 ) ) ;
#26497=CARTESIAN_POINT ( 'NONE',  ( 161.0000000000000284, 3.467572205841706889, 4.269185284954735593 ) ) ;
#26498=( BOUNDED_SURFACE ( )  B_SPLINE_SURFACE ( 3, 2, ( 
 ( #13522, #9336, #30368 ),
 ( #27739, #16292, #25764 ),
 ( #22862, #11677, #1961 ),
 ( #8883, #29903, #14143 ),
 ( #1800, #4406, #25442 ),
 ( #21170, #18726, #112 ),
 ( #11206, #23176, #25135 ),
 ( #18575, #23015, #15836 ),
 ( #20713, #28199, #16136 ),
 ( #4100, #20552, #18271 ),
 ( #27583, #6561, #4253 ),
 ( #15982, #13674, #9030 ),
 ( #18419, #20865, #11366 ),
 ( #13831, #30215, #9178 ) ),
 .UNSPECIFIED., .F., .F., .T. ) 
 B_SPLINE_SURFACE_WITH_KNOTS ( ( 4, 2, 2, 2, 2, 2, 4 ),
 ( 3, 3 ),
 ( 0.007035869656342713836, 0.007146012451658744456, 0.007256155246974775076, 0.007311226644632790386, 0.007366298042290805696, 0.007421369439948821006, 0.007476440837606836316 ),
 ( 0.000000000000000000, 1.000000000000000000 ),
 .UNSPECIFIED. ) 
 GEOMETRIC_REPRESENTATION_ITEM ( )  RATIONAL_B_SPLINE_SURFACE ( (
 ( 1.000000000000000000, 0.7743236465966892856, 1.000000000000000000),
 ( 1.000000000000000000, 0.7823573883663251793, 1.000000000000000000),
 ( 1.000000000000000000, 0.7919060189340916267, 1.000000000000000000),
 ( 1.000000000000000000, 0.8152203555693537940, 1.000000000000000000),
 ( 1.000000000000000000, 0.8293580484731973845, 1.000000000000000000),
 ( 1.000000000000000000, 0.8517285253148718649, 1.000000000000000000),
 ( 1.000000000000000000, 0.8593271320052130458, 1.000000000000000000),
 ( 1.000000000000000000, 0.8720599197349646614, 1.000000000000000000),
 ( 1.000000000000000000, 0.8771186710024685418, 1.000000000000000000),
 ( 1.000000000000000000, 0.8813077611509017029, 1.000000000000000000),
 ( 1.000000000000000000, 0.8802096620080653855, 1.000000000000000000),
 ( 1.000000000000000000, 0.8725983457344340666, 1.000000000000000000),
 ( 1.000000000000000000, 0.8663204784655903490, 1.000000000000000000),
 ( 1.000000000000000000, 0.8593225670956808893, 1.000000000000000000) ) ) 
 REPRESENTATION_ITEM ( '' )  SURFACE ( )  );
#26499=EDGE_CURVE ( 'NONE', #10998, #13277, #16229, .T. ) ;
#26500=ORIENTED_EDGE ( 'NONE', *, *, #3601, .T. ) ;
#26501=CARTESIAN_POINT ( 'NONE',  ( 161.5312500000000568, -2.485281374238555774, -6.000000000000005329 ) ) ;
#26505=VECTOR ( 'NONE', #19525, 1000.000000000000000 ) ;
#26506=VERTEX_POINT ( 'NONE', #16724 ) ;
#26509=ORIENTED_EDGE ( 'NONE', *, *, #13249, .F. ) ;
#26510=ORIENTED_EDGE ( 'NONE', *, *, #5928, .F. ) ;
#26514=AXIS2_PLACEMENT_3D ( 'NONE', #7120, #20971, #27537 ) ;
#26519=LINE ( 'NONE', #29270, #23849 ) ;
#26524=FACE_OUTER_BOUND ( 'NONE', #1056, .T. ) ;
#26527=CARTESIAN_POINT ( 'NONE',  ( -0.01297627431098077530, -14.38419007667407890, 8.362424020360270660 ) ) ;
#26529=FACE_OUTER_BOUND ( 'NONE', #9726, .T. ) ;
#26537=EDGE_LOOP ( 'NONE', ( #22608, #10631, #11429, #29904 ) ) ;
#26544=AXIS2_PLACEMENT_3D ( 'NONE', #11491, #2087, #18841 ) ;
#26545=DIRECTION ( 'NONE',  ( 0.000000000000000000, 0.000000000000000000, -1.000000000000000000 ) ) ;
#26550=FACE_OUTER_BOUND ( 'NONE', #2562, .T. ) ;
#26553=CARTESIAN_POINT ( 'NONE',  ( 159.8437500000000000, -6.000000000000005329, -2.485281374238555774 ) ) ;
#26554=CIRCLE ( 'NONE', #11912, 1.000000000000000000 ) ;
#26555=ORIENTED_EDGE ( 'NONE', *, *, #22651, .F. ) ;
#26559=CARTESIAN_POINT ( 'NONE',  ( 0.000000000000000000, -10.00000000000000888, -5.000000000000004441 ) ) ;
#26565=CARTESIAN_POINT ( 'NONE',  ( 139.5788997308104342, -4.999999999999989342, 2.071067811865468400 ) ) ;
#26566=DIRECTION ( 'NONE',  ( 0.000000000000000000, 0.000000000000000000, 1.000000000000000000 ) ) ;
#26570=ADVANCED_FACE ( 'NONE', ( #16281 ), #24859, .F. ) ;
#26578=CARTESIAN_POINT ( 'NONE',  ( 0.000000000000000000, 9.000000000000007105, 3.000000000000002665 ) ) ;
#26579=EDGE_LOOP ( 'NONE', ( #20085, #9469, #3453, #21210 ) ) ;
#26583=CARTESIAN_POINT ( 'NONE',  ( -38.99999999999998579, -59.99999999999980105, 3.000000000000002665 ) ) ;
#26585=ORIENTED_EDGE ( 'NONE', *, *, #21814, .T. ) ;
#26587=ORIENTED_EDGE ( 'NONE', *, *, #13519, .F. ) ;
#26590=CARTESIAN_POINT ( 'NONE',  ( 140.5386751345948255, -5.500000000000005329, 0.000000000000000000 ) ) ;
#26596=CARTESIAN_POINT ( 'NONE',  ( 158.7038997308104058, 2.071067811865468400, 4.999999999999989342 ) ) ;
#26597=CARTESIAN_POINT ( 'NONE',  ( 152.8199251345948255, -2.278174593051950136, -5.500000000000074607 ) ) ;
#26598=SURFACE_SIDE_STYLE ('',( #7865 ) ) ;
#26599=EDGE_CURVE ( 'NONE', #1119, #17742, #24995, .T. ) ;
#26605=LINE ( 'NONE', #14670, #2742 ) ;
#26606=FILL_AREA_STYLE ('',( #26457 ) ) ;
#26610=CARTESIAN_POINT ( 'NONE',  ( 137.4523502691896510, 0.000000000000000000, 5.000000000000004441 ) ) ;
#26611=CARTESIAN_POINT ( 'NONE',  ( 153.0000000000000284, 6.000000000000005329, 0.000000000000000000 ) ) ;
#26614=VECTOR ( 'NONE', #20585, 1000.000000000000000 ) ;
#26616=CARTESIAN_POINT ( 'NONE',  ( 144.4687500000000568, -2.485281374238585972, 6.000000000000005329 ) ) ;
#26617=CARTESIAN_POINT ( 'NONE',  ( 161.4205085250501668, -5.148837675204802622, -2.939615011427564539 ) ) ;
#26627=DIRECTION ( 'NONE',  ( 0.000000000000000000, 0.000000000000000000, 1.000000000000000000 ) ) ;
#26629=EDGE_CURVE ( 'NONE', #5531, #9311, #12710, .T. ) ;
#26634=( BOUNDED_CURVE ( )  B_SPLINE_CURVE ( 2, ( #7348, #2443, #28071, #30082, #16755, #21043, #5021, #14451, #573 ),
 .UNSPECIFIED., .F., .F. ) 
 B_SPLINE_CURVE_WITH_KNOTS ( ( 3, 2, 2, 2, 3 ),
 ( 0.08749999999999961975, 0.09374999999999986122, 0.1000000000000000888, 0.1062500000000003164, 0.1125000000000005579 ),
 .UNSPECIFIED. ) 
 CURVE ( )  GEOMETRIC_REPRESENTATION_ITEM ( )  RATIONAL_B_SPLINE_CURVE ( ( 1.000000000000004663, 0.9238795325112821866, 1.000000000000000000, 0.9238795325112867385, 1.000000000000000000, 0.9238795325112867385, 1.000000000000000000, 0.9238795325112799661, 1.000000000000006661 ) ) 
 REPRESENTATION_ITEM ( '' )  );
#26636=PRESENTATION_STYLE_ASSIGNMENT (( #10864 ) ) ;
#26638=CARTESIAN_POINT ( 'NONE',  ( 153.3898502691896510, 3.535533905932725318, -3.535533905932725318 ) ) ;
#26640=CARTESIAN_POINT ( 'NONE',  ( 161.0000000000000284, -5.424442335930618420, -0.9085292203135086897 ) ) ;
#26641=CARTESIAN_POINT ( 'NONE',  ( 1.000000000000000888, -14.99923475244191451, 9.015151515151503148 ) ) ;
#26646=CARTESIAN_POINT ( 'NONE',  ( 159.4687500000000568, -2.485281374238585972, 6.000000000000005329 ) ) ;
#26650=CIRCLE ( 'NONE', #13474, 6.499999999999977796 ) ;
#26651=ADVANCED_FACE ( 'NONE', ( #10383 ), #6833, .F. ) ;
#26655=EDGE_LOOP ( 'NONE', ( #24894, #10299, #8938, #27642 ) ) ;
#26659=CARTESIAN_POINT ( 'NONE',  ( 147.2886751345948539, 5.500000000000005329, 0.000000000000000000 ) ) ;
#26662=CARTESIAN_POINT ( 'NONE',  ( -0.06967686769852464435, -14.74880632522791579, -8.209202207805669005 ) ) ;
#26664=ADVANCED_FACE ( 'NONE', ( #3136 ), #21904, .F. ) ;
#26671=CARTESIAN_POINT ( 'NONE',  ( 154.9613248654052029, -5.500000000000005329, 0.000000000000000000 ) ) ;
#26674=CARTESIAN_POINT ( 'NONE',  ( 135.0710398743875373, -7.730392528201072366, 8.358534351738736490 ) ) ;
#26681=DIRECTION ( 'NONE',  ( -1.000000000000000000, 3.469446951953694061E-16, 0.000000000000000000 ) ) ;
#26682=ORIENTED_EDGE ( 'NONE', *, *, #23823, .F. ) ;
#26685=SURFACE_SIDE_STYLE ('',( #28846 ) ) ;
#26689=ORIENTED_EDGE ( 'NONE', *, *, #15571, .T. ) ;
#26690=CARTESIAN_POINT ( 'NONE',  ( 132.7648502691896510, 3.535533905932725318, 3.535533905932752852 ) ) ;
#26691=ADVANCED_FACE ( 'NONE', ( #24940 ), #29398, .F. ) ;
#26692=ORIENTED_EDGE ( 'NONE', *, *, #14228, .F. ) ;
#26698=EDGE_CURVE ( 'NONE', #28026, #16343, #1134, .T. ) ;
#26701=CARTESIAN_POINT ( 'NONE',  ( 134.6101497308104342, 3.535533905932725318, 3.535533905932725318 ) ) ;
#26707=PLANE ( 'NONE',  #6882 ) ;
#26709=CARTESIAN_POINT ( 'NONE',  ( 1.000000000000000888, -15.13479642978409245, -8.789606617933440447 ) ) ;
#26711=EDGE_LOOP ( 'NONE', ( #16595, #20161, #15133, #24307, #14880, #27493, #25613, #12771, #16418, #24204, #5569, #3914, #28033, #6623, #12483, #29260 ) ) ;
#26713=CIRCLE ( 'NONE', #28191, 17.50000000000000355 ) ;
#26714=DIRECTION ( 'NONE',  ( 0.000000000000000000, 0.000000000000000000, -1.000000000000000000 ) ) ;
#26718=ORIENTED_EDGE ( 'NONE', *, *, #20813, .F. ) ;
#26722=SURFACE_STYLE_USAGE ( .BOTH. , #12509 ) ;
#26723=CARTESIAN_POINT ( 'NONE',  ( 155.3511751345948539, -3.889087296526011706, 3.889087296526011706 ) ) ;
#26725=CARTESIAN_POINT ( 'NONE',  ( 140.0000000000000284, -11.48545691804907420, 4.867024281885878878 ) ) ;
#26726=ORIENTED_EDGE ( 'NONE', *, *, #30256, .F. ) ;
#26727=CARTESIAN_POINT ( 'NONE',  ( 141.0000000000000284, -12.00000000000001066, 4.000000000000003553 ) ) ;
#26736=CARTESIAN_POINT ( 'NONE',  ( 157.3913997308104058, -2.071067811865468400, 4.999999999999989342 ) ) ;
#26738=DIRECTION ( 'NONE',  ( 1.000000000000000000, -0.000000000000000000, -0.000000000000000000 ) ) ;
#26744=FACE_OUTER_BOUND ( 'NONE', #18742, .T. ) ;
#26748=CARTESIAN_POINT ( 'NONE',  ( 154.5000000000000284, 6.000000000000005329, 0.000000000000000000 ) ) ;
#26749=CARTESIAN_POINT ( 'NONE',  ( 142.2261751345948539, -3.889087296526011706, -3.889087296526011706 ) ) ;
#26755=CARTESIAN_POINT ( 'NONE',  ( 144.5625000000000284, -4.242640687119298093, 4.242640687119298093 ) ) ;
#26763=VERTEX_POINT ( 'NONE', #18220 ) ;
#26769=LINE ( 'NONE', #834, #15807 ) ;
#26773=CARTESIAN_POINT ( 'NONE',  ( 134.9985123063161723, -7.386692690774673054, 8.423607852766412663 ) ) ;
#26778=DIRECTION ( 'NONE',  ( 1.000000000000000000, 0.000000000000000000, 0.000000000000000000 ) ) ;
#26780=FACE_OUTER_BOUND ( 'NONE', #1810, .T. ) ;
#26782=CARTESIAN_POINT ( 'NONE',  ( 152.1711002691896226, 4.999999999999989342, 2.071067811865468400 ) ) ;
#26783=CARTESIAN_POINT ( 'NONE',  ( 152.1636751345948255, 0.000000000000000000, 5.500000000000005329 ) ) ;
#26784=VECTOR ( 'NONE', #23712, 1000.000000000000000 ) ;
#26785=AXIS2_PLACEMENT_3D ( 'NONE', #15909, #25206, #15595 ) ;
#26788=CARTESIAN_POINT ( 'NONE',  ( -4.999999999999886313, -9.000000000000007105, 5.000000000000004441 ) ) ;
#26791=( LENGTH_UNIT ( ) NAMED_UNIT ( * ) SI_UNIT ( .MILLI., .METRE. ) );
#26797=EDGE_LOOP ( 'NONE', ( #7654, #27946, #22838, #5804 ) ) ;
#26799=( GEOMETRIC_REPRESENTATION_CONTEXT ( 3 ) GLOBAL_UNCERTAINTY_ASSIGNED_CONTEXT ( ( #2975 ) ) GLOBAL_UNIT_ASSIGNED_CONTEXT ( ( #20026, #6036, #1269 ) ) REPRESENTATION_CONTEXT ( 'NONE', 'WORKASPACE' ) );
#26800=CIRCLE ( 'NONE', #12174, 0.5000000000000000000 ) ;
#26802=ORIENTED_EDGE ( 'NONE', *, *, #9187, .T. ) ;
#26804=CYLINDRICAL_SURFACE ( 'NONE', #2942, 5.500000000000000000 ) ;
#26805=CARTESIAN_POINT ( 'NONE',  ( 147.5699251345948255, 2.278174593052259667, 5.499999999999763745 ) ) ;
#26813=CIRCLE ( 'NONE', #348, 0.5000000000000004441 ) ;
#26817=CARTESIAN_POINT ( 'NONE',  ( 140.5000000000000284, -9.599999999999997868, 7.200000000000011724 ) ) ;
#26821=PLANE ( 'NONE',  #10125 ) ;
#26827=AXIS2_PLACEMENT_3D ( 'NONE', #25956, #23672, #7072 ) ;
#26828=FACE_OUTER_BOUND ( 'NONE', #12919, .T. ) ;
#26829=ORIENTED_EDGE ( 'NONE', *, *, #13949, .F. ) ;
#26831=CARTESIAN_POINT ( 'NONE',  ( 139.3988248654052313, 3.889087296526011706, 3.889087296526011706 ) ) ;
#26833=DIRECTION ( 'NONE',  ( 0.000000000000000000, 1.776356839400250465E-15, -1.000000000000000000 ) ) ;
#26837=AXIS2_PLACEMENT_3D ( 'NONE', #5482, #19498, #3180 ) ;
#26838=ORIENTED_EDGE ( 'NONE', *, *, #22049, .F. ) ;
#26839=ORIENTED_EDGE ( 'NONE', *, *, #6477, .F. ) ;
#26840=CARTESIAN_POINT ( 'NONE',  ( 134.7336002691896795, -4.999999999999989342, 2.071067811865468400 ) ) ;
#26843=CARTESIAN_POINT ( 'NONE',  ( 157.4925748654052313, 2.278174593051919494, 5.500000000000105693 ) ) ;
#26849=EDGE_LOOP ( 'NONE', ( #7033, #23565, #12939, #12003, #21739, #9923, #14791, #26914, #6877, #3235, #19297, #9761 ) ) ;
#26850=AXIS2_PLACEMENT_3D ( 'NONE', #18088, #29717, #17628 ) ;
#26853=( BOUNDED_CURVE ( )  B_SPLINE_CURVE ( 2, ( #17296, #6040, #15135, #24621, #12696, #3268, #24928, #3729, #5571 ),
 .UNSPECIFIED., .F., .T. ) 
 B_SPLINE_CURVE_WITH_KNOTS ( ( 3, 2, 2, 2, 3 ),
 ( 0.6125000000000010436, 0.6187500000000007994, 0.6250000000000006661, 0.6312500000000004219, 0.6375000000000001776 ),
 .UNSPECIFIED. ) 
 CURVE ( )  GEOMETRIC_REPRESENTATION_ITEM ( )  RATIONAL_B_SPLINE_CURVE ( ( 0.9999999999999877875, 0.9238795325112989509, 1.000000000000000000, 0.9238795325112867385, 1.000000000000000000, 0.9238795325112867385, 1.000000000000000000, 0.9238795325112840739, 1.000000000000002665 ) ) 
 REPRESENTATION_ITEM ( '' )  );
#26865=EDGE_CURVE ( 'NONE', #29031, #3651, #17118, .T. ) ;
#26873=ORIENTED_EDGE ( 'NONE', *, *, #19855, .T. ) ;
#26879=ADVANCED_FACE ( 'NONE', ( #26373 ), #2926, .T. ) ;
#26880=CARTESIAN_POINT ( 'NONE',  ( 158.1636751345948255, 0.000000000000000000, 5.500000000000005329 ) ) ;
#26882=LINE ( 'NONE', #24143, #20872 ) ;
#26885=CARTESIAN_POINT ( 'NONE',  ( 160.9318293186996414, -11.54853638030490259, 3.263004215147740084 ) ) ;
#26890=CARTESIAN_POINT ( 'NONE',  ( 148.7663997308104058, -4.999999999999989342, -2.071067811865468400 ) ) ;
#26894=FACE_OUTER_BOUND ( 'NONE', #26797, .T. ) ;
#26897=DIRECTION ( 'NONE',  ( 1.000000000000000000, 0.000000000000000000, 0.000000000000000000 ) ) ;
#26903=CARTESIAN_POINT ( 'NONE',  ( 137.1636751345948255, 0.000000000000000000, 5.500000000000005329 ) ) ;
#26905=CARTESIAN_POINT ( 'NONE',  ( 144.4687500000000568, -2.485281374238585972, 6.000000000000005329 ) ) ;
#26906=CARTESIAN_POINT ( 'NONE',  ( 141.9449251345948255, -5.500000000000012434, 2.278174593052012309 ) ) ;
#26910=ADVANCED_FACE ( 'NONE', ( #17492 ), #26804, .F. ) ;
#26912=CARTESIAN_POINT ( 'NONE',  ( 143.8125000000000284, 4.242640687119298093, -4.242640687119298093 ) ) ;
#26913=CARTESIAN_POINT ( 'NONE',  ( 161.1118616798009953, -0.3161702963393516752, 5.611861679801007696 ) ) ;
#26914=ORIENTED_EDGE ( 'NONE', *, *, #27125, .T. ) ;
#26917=AXIS2_PLACEMENT_3D ( 'NONE', #24266, #917, #12796 ) ;
#26920=ORIENTED_EDGE ( 'NONE', *, *, #26299, .T. ) ;
#26924=EDGE_LOOP ( 'NONE', ( #5878, #23936, #10174, #28805 ) ) ;
#26929=CARTESIAN_POINT ( 'NONE',  ( -4.999999999999879208, -70.00000000000001421, -5.000000000000004441 ) ) ;
#26932=DIRECTION ( 'NONE',  ( 1.000000000000000000, 0.000000000000000000, 0.000000000000000000 ) ) ;
#26936=UNCERTAINTY_MEASURE_WITH_UNIT (LENGTH_MEASURE( 1.000000000000000082E-05 ), #17500, 'distance_accuracy_value', 'NONE');
#26937=EDGE_CURVE ( 'NONE', #11692, #20342, #13303, .T. ) ;
#26938=AXIS2_PLACEMENT_3D ( 'NONE', #27729, #4992, #18561 ) ;
#26941=TOROIDAL_SURFACE ( 'NONE', #20113, 16.50000000000000355, 1.000000000000000000 ) ;
#26942=CARTESIAN_POINT ( 'NONE',  ( 135.8363248654052029, 0.000000000000000000, -5.500000000000005329 ) ) ;
#26943=CARTESIAN_POINT ( 'NONE',  ( 153.2023502691896510, 0.000000000000000000, -5.000000000000004441 ) ) ;
#26946=STYLED_ITEM ( 'NONE', ( #22395 ), #13969 ) ;
#26947=CARTESIAN_POINT ( 'NONE',  ( 144.7425748654051461, -2.278174593052290753, -5.499999999999732658 ) ) ;
#26948=CARTESIAN_POINT ( 'NONE',  ( 160.4136751345948824, 0.000000000000000000, -5.500000000000005329 ) ) ;
#26950=EDGE_CURVE ( 'NONE', #22266, #2390, #9624, .T. ) ;
#26960=COLOUR_RGB ( '', 0.72549020, 0.75294118, 0.79215686) ;
#26969=CARTESIAN_POINT ( 'NONE',  ( 146.6324251345948539, -5.500000000000012434, -2.278174593052012309 ) ) ;
#26975=CARTESIAN_POINT ( 'NONE',  ( -9.757819552369539906E-16, -10.00000000000000888, 5.000000000000004441 ) ) ;
#26976=EDGE_CURVE ( 'NONE', #7376, #18429, #25903, .T. ) ;
#26978=CARTESIAN_POINT ( 'NONE',  ( -4.999999999999990230, -24.99999999999999289, -5.000000000000004441 ) ) ;
#26982=CARTESIAN_POINT ( 'NONE',  ( 135.0000000000000284, -8.448271545446896624, 7.965230813406249055 ) ) ;
#26985=CYLINDRICAL_SURFACE ( 'NONE', #22152, 1.000000000000000000 ) ;
#26992=CARTESIAN_POINT ( 'NONE',  ( -0.5000000000000004441, -10.50000000000000888, -8.500000000000007105 ) ) ;
#26995=ORIENTED_EDGE ( 'NONE', *, *, #17627, .T. ) ;
#26997=AXIS2_PLACEMENT_3D ( 'NONE', #20350, #6210, #15148 ) ;
#26999=ORIENTED_EDGE ( 'NONE', *, *, #16966, .F. ) ;
#27000=CARTESIAN_POINT ( 'NONE',  ( 156.0937500000000000, 6.000000000000005329, 2.485281374238585972 ) ) ;
#27007=CYLINDRICAL_SURFACE ( 'NONE', #9851, 1.000000000000000888 ) ;
#27009=CARTESIAN_POINT ( 'NONE',  ( 135.5000000000000284, -9.047800747817580813, -8.000000000000007105 ) ) ;
#27010=DIRECTION ( 'NONE',  ( 1.000000000000000000, 0.000000000000000000, 0.000000000000000000 ) ) ;
#27011=AXIS2_PLACEMENT_3D ( 'NONE', #1826, #11230, #8907 ) ;
#27012=ORIENTED_EDGE ( 'NONE', *, *, #19067, .F. ) ;
#27014=CARTESIAN_POINT ( 'NONE',  ( 0.1950273200666168272, -15.66255992321440438, -7.807776097887558997 ) ) ;
#27018=CARTESIAN_POINT ( 'NONE',  ( 0.7660434483343199208, -15.49920295329753550, -8.125643190292789697 ) ) ;
#27022=CARTESIAN_POINT ( 'NONE',  ( 159.0000000000000284, -59.99999999999980105, 4.000000000000003553 ) ) ;
#27024=CARTESIAN_POINT ( 'NONE',  ( 147.6636751345948255, 0.000000000000000000, 5.500000000000005329 ) ) ;
#27034=( NAMED_UNIT ( * ) PLANE_ANGLE_UNIT ( ) SI_UNIT ( $, .RADIAN. ) );
#27036=CARTESIAN_POINT ( 'NONE',  ( 135.0000000000000284, 4.401348733996699458, -3.652467542001735179 ) ) ;
#27040=CARTESIAN_POINT ( 'NONE',  ( 159.9746938747179854, -12.51900727150228931, 3.255903183154158498 ) ) ;
#27041=CARTESIAN_POINT ( 'NONE',  ( 140.1562500000000853, -6.000000000000005329, 2.485281374238555774 ) ) ;
#27042=( BOUNDED_CURVE ( )  B_SPLINE_CURVE ( 2, ( #1069, #3354, #12628, #10459, #19382, #19232, #17088, #26267, #5512 ),
 .UNSPECIFIED., .F., .T. ) 
 B_SPLINE_CURVE_WITH_KNOTS ( ( 3, 2, 2, 2, 3 ),
 ( 0.5624999999999991118, 0.5687499999999993117, 0.5749999999999995115, 0.5812499999999999334, 0.5875000000000001332 ),
 .UNSPECIFIED. ) 
 CURVE ( )  GEOMETRIC_REPRESENTATION_ITEM ( )  RATIONAL_B_SPLINE_CURVE ( ( 1.000000000000010880, 0.9238795325112759693, 1.000000000000000000, 0.9238795325112867385, 1.000000000000000000, 0.9238795325112867385, 1.000000000000000000, 0.9238795325112854062, 1.000000000000001332 ) ) 
 REPRESENTATION_ITEM ( '' )  );
#27044=CIRCLE ( 'NONE', #10391, 0.5000000000000000000 ) ;
#27052=CARTESIAN_POINT ( 'NONE',  ( 149.0476497308104058, 0.000000000000000000, -5.000000000000004441 ) ) ;
#27055=PRESENTATION_STYLE_ASSIGNMENT (( #13139 ) ) ;
#27056=VECTOR ( 'NONE', #5572, 1000.000000000000000 ) ;
#27066=ORIENTED_EDGE ( 'NONE', *, *, #10130, .F. ) ;
#27068=CARTESIAN_POINT ( 'NONE',  ( 145.5000000000000284, 6.000000000000005329, 0.000000000000000000 ) ) ;
#27071=VECTOR ( 'NONE', #12390, 1000.000000000000114 ) ;
#27074=CARTESIAN_POINT ( 'NONE',  ( 147.0000000000000284, 6.000000000000005329, 0.000000000000000000 ) ) ;
#27075=CARTESIAN_POINT ( 'NONE',  ( 161.1719978263368205, -2.466862157723925364, 5.117282274813819143 ) ) ;
#27076=VERTEX_POINT ( 'NONE', #13351 ) ;
#27080=VERTEX_POINT ( 'NONE', #11032 ) ;
#27087=CARTESIAN_POINT ( 'NONE',  ( -9.999999999999793943, 9.000000000000007105, -4.000000000000003553 ) ) ;
#27092=EDGE_CURVE ( 'NONE', #20296, #24857, #21126, .T. ) ;
#27094=CARTESIAN_POINT ( 'NONE',  ( 137.0550748654052597, -5.500000000000012434, -2.278174593052012309 ) ) ;
#27098=CYLINDRICAL_SURFACE ( 'NONE', #180, 15.00000000000000000 ) ;
#27101=CIRCLE ( 'NONE', #2605, 15.00000000000000000 ) ;
#27103=CARTESIAN_POINT ( 'NONE',  ( 0.000000000000000000, -14.14213562373095634, 8.500000000000007105 ) ) ;
#27104=DIRECTION ( 'NONE',  ( 0.000000000000000000, 1.000000000000000000, 0.000000000000000000 ) ) ;
#27109=ORIENTED_EDGE ( 'NONE', *, *, #3574, .T. ) ;
#27111=CARTESIAN_POINT ( 'NONE',  ( 145.8824251345948539, 5.500000000000012434, 2.278174593052012309 ) ) ;
#27114=EDGE_CURVE ( 'NONE', #23700, #16823, #13972, .T. ) ;
#27118=CIRCLE ( 'NONE', #15409, 28.99999999999999645 ) ;
#27124=CARTESIAN_POINT ( 'NONE',  ( -4.999999999999886313, -14.50000000000001243, -7.500000000000007105 ) ) ;
#27125=EDGE_CURVE ( 'NONE', #15294, #14644, #487, .T. ) ;
#27130=CYLINDRICAL_SURFACE ( 'NONE', #7441, 14.99999999999998579 ) ;
#27137=DIRECTION ( 'NONE',  ( -0.000000000000000000, -0.000000000000000000, -1.000000000000000000 ) ) ;
#27139=( BOUNDED_CURVE ( )  B_SPLINE_CURVE ( 2, ( #24592, #1097, #19998, #6010, #10813, #8311, #3695, #20163, #15429 ),
 .UNSPECIFIED., .F., .T. ) 
 B_SPLINE_CURVE_WITH_KNOTS ( ( 3, 2, 2, 2, 3 ),
 ( 0.8375000000000002442, 0.8437500000000004441, 0.8500000000000007550, 0.8562500000000009548, 0.8625000000000012657 ),
 .UNSPECIFIED. ) 
 CURVE ( )  GEOMETRIC_REPRESENTATION_ITEM ( )  RATIONAL_B_SPLINE_CURVE ( ( 0.9999999999999973355, 0.9238795325112894030, 1.000000000000000000, 0.9238795325112867385, 1.000000000000000000, 0.9238795325112867385, 1.000000000000000000, 0.9238795325112718615, 1.000000000000014877 ) ) 
 REPRESENTATION_ITEM ( '' )  );
#27147=ORIENTED_EDGE ( 'NONE', *, *, #9048, .T. ) ;
#27151=ORIENTED_EDGE ( 'NONE', *, *, #7338, .T. ) ;
#27154=EDGE_LOOP ( 'NONE', ( #16263, #21001, #27012, #24511 ) ) ;
#27155=CARTESIAN_POINT ( 'NONE',  ( 158.2500000000000284, -6.000000000000005329, 0.000000000000000000 ) ) ;
#27156=ADVANCED_FACE ( 'NONE', ( #11663 ), #21007, .F. ) ;
#27164=CARTESIAN_POINT ( 'NONE',  ( 159.7627798038683693, -11.43531980891128796, 3.685954457582622190 ) ) ;
#27165=VERTEX_POINT ( 'NONE', #28107 ) ;
#27170=DIRECTION ( 'NONE',  ( 0.000000000000000000, 0.000000000000000000, 1.000000000000000000 ) ) ;
#27175=DIRECTION ( 'NONE',  ( -0.000000000000000000, -0.000000000000000000, 1.000000000000000000 ) ) ;
#27178=AXIS2_PLACEMENT_3D ( 'NONE', #14793, #19402, #12059 ) ;
#27185=CARTESIAN_POINT ( 'NONE',  ( 137.3586002691896226, 2.071067811865468400, 4.999999999999989342 ) ) ;
#27188=FACE_OUTER_BOUND ( 'NONE', #25069, .T. ) ;
#27193=ORIENTED_EDGE ( 'NONE', *, *, #1936, .F. ) ;
#27195=CARTESIAN_POINT ( 'NONE',  ( 142.9687500000000000, -2.485281374238585972, 6.000000000000005329 ) ) ;
#27197=ADVANCED_FACE ( 'NONE', ( #9702 ), #7386, .F. ) ;
#27199=CARTESIAN_POINT ( 'NONE',  ( 159.4761751345948255, 3.889087296526011706, 3.889087296526011706 ) ) ;
#27203=DIRECTION ( 'NONE',  ( -1.000000000000000000, -0.000000000000000000, -0.000000000000000000 ) ) ;
#27204=CARTESIAN_POINT ( 'NONE',  ( 147.7351497308104342, 3.535533905932725318, -3.535533905932725318 ) ) ;
#27207=CIRCLE ( 'NONE', #24786, 1.000000000000000888 ) ;
#27210=CARTESIAN_POINT ( 'NONE',  ( 135.0085428039600970, -7.340339031313663831, 8.407416807790594859 ) ) ;
#27219=CARTESIAN_POINT ( 'NONE',  ( 143.3437500000000853, -6.000000000000005329, -2.485281374238556218 ) ) ;
#27225=CARTESIAN_POINT ( 'NONE',  ( 135.9375000000000568, -4.242640687119298093, -4.242640687119298093 ) ) ;
#27226=CARTESIAN_POINT ( 'NONE',  ( 161.4122677408628874, -5.290788382733226491, -2.657712799832109063 ) ) ;
#27236=AXIS2_PLACEMENT_3D ( 'NONE', #23167, #2111, #11515 ) ;
#27237=CARTESIAN_POINT ( 'NONE',  ( -10.00000000000000178, 9.000000000000007105, -4.000000000000003553 ) ) ;
#27238=DIRECTION ( 'NONE',  ( 0.000000000000000000, 0.000000000000000000, 1.000000000000000000 ) ) ;
#27239=CARTESIAN_POINT ( 'NONE',  ( 148.0238248654052313, 3.889087296526011706, -3.889087296526011706 ) ) ;
#27244=CARTESIAN_POINT ( 'NONE',  ( 156.5550748654052029, -5.500000000000012434, -2.278174593052012309 ) ) ;
#27245=AXIS2_PLACEMENT_3D ( 'NONE', #7653, #14604, #16915 ) ;
#27249=CARTESIAN_POINT ( 'NONE',  ( 152.4523502691896510, 0.000000000000000000, 5.000000000000004441 ) ) ;
#27250=CARTESIAN_POINT ( 'NONE',  ( 161.3393457717174044, -4.235451996440949607, -4.042466237327082546 ) ) ;
#27251=DIRECTION ( 'NONE',  ( 0.000000000000000000, 1.000000000000000000, -0.000000000000000000 ) ) ;
#27254=CARTESIAN_POINT ( 'NONE',  ( 116.0000000000000142, 6.735557395310442023E-16, 5.500000000000000000 ) ) ;
#27256=ORIENTED_EDGE ( 'NONE', *, *, #3456, .T. ) ;
#27257=CARTESIAN_POINT ( 'NONE',  ( 157.3125000000000284, 4.242640687119298093, -4.242640687119298093 ) ) ;
#27260=AXIS2_PLACEMENT_3D ( 'NONE', #8564, #12759, #3481 ) ;
#27262=ADVANCED_FACE ( 'NONE', ( #19375 ), #28699, .F. ) ;
#27263=ORIENTED_EDGE ( 'NONE', *, *, #5413, .F. ) ;
#27267=ORIENTED_EDGE ( 'NONE', *, *, #1648, .T. ) ;
#27268=DIRECTION ( 'NONE',  ( 0.000000000000000000, 0.000000000000000000, -1.000000000000000000 ) ) ;
#27272=EDGE_LOOP ( 'NONE', ( #29845, #7076, #259, #11986 ) ) ;
#27273=SHAPE_REPRESENTATION_RELATIONSHIP ( 'NONE' , 'NONE' ,  #15661, #13685 ) ;
#27278=CARTESIAN_POINT ( 'NONE',  ( 160.0000000000000284, -12.64911064067353408, -3.000000000000002665 ) ) ;
#27285=ORIENTED_EDGE ( 'NONE', *, *, #16540, .F. ) ;
#27288=ADVANCED_FACE ( 'NONE', ( #16645 ), #18786, .F. ) ;
#27299=EDGE_CURVE ( 'NONE', #14042, #22235, #14319, .T. ) ;
#27303=CARTESIAN_POINT ( 'NONE',  ( 153.7500000000000284, -6.000000000000005329, 0.000000000000000000 ) ) ;
#27313=CARTESIAN_POINT ( 'NONE',  ( 159.2646601775326474, -12.02761966486299627, 3.966636896921674982 ) ) ;
#27321=CARTESIAN_POINT ( 'NONE',  ( 140.2425748654052029, -2.278174593052322283, -5.499999999999701572 ) ) ;
#27322=DIRECTION ( 'NONE',  ( 1.000000000000000000, -3.469446951953694061E-16, 0.000000000000000000 ) ) ;
#27328=DIRECTION ( 'NONE',  ( 0.000000000000000000, 1.000000000000000000, -0.000000000000000000 ) ) ;
#27336=ADVANCED_FACE ( 'NONE', ( #15064 ), #27007, .T. ) ;
#27337=CARTESIAN_POINT ( 'NONE',  ( 138.2961002691896795, 2.071067811865468400, -4.999999999999989342 ) ) ;
#27347=CARTESIAN_POINT ( 'NONE',  ( 160.0000000000000284, -12.64911064067353408, 3.000000000000002665 ) ) ;
#27348=CARTESIAN_POINT ( 'NONE',  ( 139.5937500000000284, 6.000000000000005329, 2.485281374238585972 ) ) ;
#27349=AXIS2_PLACEMENT_3D ( 'NONE', #28594, #9591, #26008 ) ;
#27355=CARTESIAN_POINT ( 'NONE',  ( -9.999999999999765521, -89.00000000000001421, -3.000000000000002665 ) ) ;
#27356=CARTESIAN_POINT ( 'NONE',  ( 151.8601497308104058, -3.535533905932725318, -3.535533905932725318 ) ) ;
#27371=CARTESIAN_POINT ( 'NONE',  ( 144.6562500000000284, -6.000000000000005329, 2.485281374238556218 ) ) ;
#27373=DIRECTION ( 'NONE',  ( -0.9230769230769184652, 0.000000000000000000, 0.3846153846153959610 ) ) ;
#27375=CARTESIAN_POINT ( 'NONE',  ( 140.0625000000000284, -4.242640687119298093, 4.242640687119298093 ) ) ;
#27377=VERTEX_POINT ( 'NONE', #6927 ) ;
#27379=B_SPLINE_CURVE_WITH_KNOTS ( 'NONE', 3,
 ( #22664, #11155, #27541, #18225 ),
 .UNSPECIFIED., .F., .F.,
 ( 4, 4 ),
 ( 0.000000000000000000, 0.0004167600821326112193 ),
 .UNSPECIFIED. ) ;
#27381=ORIENTED_EDGE ( 'NONE', *, *, #9843, .T. ) ;
#27387=FACE_OUTER_BOUND ( 'NONE', #22906, .T. ) ;
#27388=CARTESIAN_POINT ( 'NONE',  ( 135.2584316331435446, -8.263189528310192600, -8.258603766105704125 ) ) ;
#27390=FACE_OUTER_BOUND ( 'NONE', #4140, .T. ) ;
#27393=CARTESIAN_POINT ( 'NONE',  ( -4.999999999999879208, -14.50000000000001243, -7.500000000000007105 ) ) ;
#27395=( BOUNDED_CURVE ( )  B_SPLINE_CURVE ( 2, ( #2462, #28391, #19904, #8376, #11018, #24810, #29574, #8530, #12875 ),
 .UNSPECIFIED., .F., .T. ) 
 B_SPLINE_CURVE_WITH_KNOTS ( ( 3, 2, 2, 2, 3 ),
 ( 0.09038686088851133338, 0.09374999999999979183, 0.09999999999999939493, 0.1062499999999989980, 0.1124999999999987121 ),
 .UNSPECIFIED. ) 
 CURVE ( )  GEOMETRIC_REPRESENTATION_ITEM ( )  RATIONAL_B_SPLINE_CURVE ( ( 0.9621607869126793666, 0.9590394045766249542, 1.000000000000000000, 0.9238795325112867385, 1.000000000000000000, 0.9238795325112867385, 1.000000000000000000, 0.9238795325113029477, 0.9999999999999837907 ) ) 
 REPRESENTATION_ITEM ( '' )  );
#27396=EDGE_CURVE ( 'NONE', #28026, #9311, #20619, .T. ) ;
#27398=CARTESIAN_POINT ( 'NONE',  ( 149.2648502691896510, 3.535533905932725318, 3.535533905932752852 ) ) ;
#27407=AXIS2_PLACEMENT_3D ( 'NONE', #6296, #2000, #23059 ) ;
#27408=CARTESIAN_POINT ( 'NONE',  ( 157.5937500000000284, 6.000000000000005329, 2.485281374238585972 ) ) ;
#27412=ORIENTED_EDGE ( 'NONE', *, *, #11869, .F. ) ;
#27416=VERTEX_POINT ( 'NONE', #16197 ) ;
#27418=CARTESIAN_POINT ( 'NONE',  ( 140.4778447815541256, -9.422006252106452706, -7.432744258808803295 ) ) ;
#27419=CARTESIAN_POINT ( 'NONE',  ( 0.8353624398881696056, -15.41361754457665612, 8.287081578747827137 ) ) ;
#27424=SURFACE_STYLE_USAGE ( .BOTH. , #22700 ) ;
#27426=DIRECTION ( 'NONE',  ( 1.000000000000000000, 0.000000000000000000, 0.000000000000000000 ) ) ;
#27429=( NAMED_UNIT ( * ) PLANE_ANGLE_UNIT ( ) SI_UNIT ( $, .RADIAN. ) );
#27430=CARTESIAN_POINT ( 'NONE',  ( 159.9449251345948539, -5.500000000000012434, 2.278174593052012309 ) ) ;
#27434=ORIENTED_EDGE ( 'NONE', *, *, #11584, .T. ) ;
#27438=CARTESIAN_POINT ( 'NONE',  ( 159.0000000000000284, -59.99999999999980105, -3.000000000000002665 ) ) ;
#27444=ORIENTED_EDGE ( 'NONE', *, *, #5486, .F. ) ;
#27446=CARTESIAN_POINT ( 'NONE',  ( 159.1875000000000284, 4.242640687119269671, 4.242640687119298093 ) ) ;
#27449=ORIENTED_EDGE ( 'NONE', *, *, #11188, .F. ) ;
#27450=CARTESIAN_POINT ( 'NONE',  ( 150.6636751345948255, 0.000000000000000000, 5.500000000000005329 ) ) ;
#27459=DIRECTION ( 'NONE',  ( 0.000000000000000000, 1.000000000000000000, 0.000000000000000000 ) ) ;
#27463=DIRECTION ( 'NONE',  ( 1.000000000000000000, 0.000000000000000000, 0.000000000000000000 ) ) ;
#27465=CARTESIAN_POINT ( 'NONE',  ( -1.000000000000002220, -9.000000000000007105, -4.000000000000005329 ) ) ;
#27467=STYLED_ITEM ( 'NONE', ( #18710 ), #27156 ) ;
#27470=EDGE_CURVE ( 'NONE', #28093, #4225, #8359, .T. ) ;
#27473=ORIENTED_EDGE ( 'NONE', *, *, #8584, .F. ) ;
#27475=CYLINDRICAL_SURFACE ( 'NONE', #10166, 1.000000000000000000 ) ;
#27477=CARTESIAN_POINT ( 'NONE',  ( 140.8273502691896510, -5.000000000000004441, 0.000000000000000000 ) ) ;
#27480=CARTESIAN_POINT ( 'NONE',  ( 124.9999999999999432, -65.00000000000000000, -7.500000000000007105 ) ) ;
#27483=CARTESIAN_POINT ( 'NONE',  ( 140.0769230769231228, -11.53846153846155254, -4.615384615384630074 ) ) ;
#27488=CARTESIAN_POINT ( 'NONE',  ( 140.4375000000000284, -4.242640687119298093, -4.242640687119298093 ) ) ;
#27491=CIRCLE ( 'NONE', #11374, 0.5000000000000004441 ) ;
#27493=ORIENTED_EDGE ( 'NONE', *, *, #12965, .T. ) ;
#27494=MECHANICAL_DESIGN_GEOMETRIC_PRESENTATION_REPRESENTATION('',(#7894),#5918);
#27499=DIRECTION ( 'NONE',  ( 0.000000000000000000, 0.000000000000000000, 1.000000000000000000 ) ) ;
#27503=CARTESIAN_POINT ( 'NONE',  ( 148.6726497308104058, -5.000000000000004441, 0.000000000000000000 ) ) ;
#27504=DIRECTION ( 'NONE',  ( 0.000000000000000000, 0.000000000000000000, -1.000000000000000000 ) ) ;
#27505=CARTESIAN_POINT ( 'NONE',  ( 0.7669223171414760731, -14.69693845669906018, 7.500000000000007105 ) ) ;
#27507=ADVANCED_FACE ( 'NONE', ( #2335 ), #3427, .T. ) ;
#27509=LINE ( 'NONE', #1878, #24030 ) ;
#27512=VECTOR ( 'NONE', #8511, 1000.000000000000000 ) ;
#27517=ORIENTED_EDGE ( 'NONE', *, *, #25214, .F. ) ;
#27520=CARTESIAN_POINT ( 'NONE',  ( 147.0937500000000284, 6.000000000000005329, 2.485281374238585972 ) ) ;
#27522=CARTESIAN_POINT ( 'NONE',  ( 138.0937500000000284, 6.000000000000005329, 2.485281374238585972 ) ) ;
#27524=ORIENTED_EDGE ( 'NONE', *, *, #24562, .F. ) ;
#27525=TOROIDAL_SURFACE ( 'NONE', #11412, 28.99999999999999645, 1.000000000000000000 ) ;
#27531=EDGE_CURVE ( 'NONE', #2984, #20340, #19240, .T. ) ;
#27533=EDGE_CURVE ( 'NONE', #2252, #1389, #617, .T. ) ;
#27537=DIRECTION ( 'NONE',  ( 0.000000000000000000, 0.000000000000000000, -1.000000000000000000 ) ) ;
#27541=CARTESIAN_POINT ( 'NONE',  ( -0.01290326774830613359, -14.38393108808779175, -8.362582996346231923 ) ) ;
#27542=VECTOR ( 'NONE', #9522, 1000.000000000000000 ) ;
#27546=CARTESIAN_POINT ( 'NONE',  ( -19.99999999999998224, -54.99999999999990763, 5.000000000000004441 ) ) ;
#27547=LINE ( 'NONE', #6524, #20602 ) ;
#27548=CARTESIAN_POINT ( 'NONE',  ( 135.5000000000000000, -9.047800747817552391, 8.000000000000007105 ) ) ;
#27549=CARTESIAN_POINT ( 'NONE',  ( 135.4709958594519037, -8.959870900750173561, -7.999999999999970690 ) ) ;
#27552=CARTESIAN_POINT ( 'NONE',  ( 150.8363248654052029, 0.000000000000000000, -5.500000000000005329 ) ) ;
#27555=CARTESIAN_POINT ( 'NONE',  ( 154.0312500000000568, -2.485281374238555774, -6.000000000000005329 ) ) ;
#27567=FACE_OUTER_BOUND ( 'NONE', #18257, .T. ) ;
#27573=CARTESIAN_POINT ( 'NONE',  ( 140.5000000000000284, -9.422078944634874276, 7.437228073820182139 ) ) ;
#27581=CARTESIAN_POINT ( 'NONE',  ( 158.8273502691896510, -5.000000000000004441, 0.000000000000000000 ) ) ;
#27583=CARTESIAN_POINT ( 'NONE',  ( -0.08237205255902971257, -15.17882982317237150, 7.764958073340198830 ) ) ;
#27589=CARTESIAN_POINT ( 'NONE',  ( 161.0173279456235207, 2.969419107450559814, 4.660845171074455173 ) ) ;
#27593=EDGE_CURVE ( 'NONE', #21900, #30382, #16273, .T. ) ;
#27595=ORIENTED_EDGE ( 'NONE', *, *, #10802, .F. ) ;
#27597=ORIENTED_EDGE ( 'NONE', *, *, #25688, .T. ) ;
#27598=CARTESIAN_POINT ( 'NONE',  ( 152.4375000000000284, -4.242640687119298093, -4.242640687119298093 ) ) ;
#27605=ORIENTED_EDGE ( 'NONE', *, *, #15085, .T. ) ;
#27606=DIRECTION ( 'NONE',  ( 1.000000000000000000, 0.000000000000000000, 0.000000000000000000 ) ) ;
#27609=CARTESIAN_POINT ( 'NONE',  ( 159.0000000000000284, -12.00000000000001066, 4.000000000000004441 ) ) ;
#27614=CARTESIAN_POINT ( 'NONE',  ( -20.99999999999998224, -54.99999999999990763, -4.000000000000003553 ) ) ;
#27615=FACE_OUTER_BOUND ( 'NONE', #26074, .T. ) ;
#27623=CARTESIAN_POINT ( 'NONE',  ( 140.5000000000000284, -9.599999999999997868, -7.200000000000011724 ) ) ;
#27625=CARTESIAN_POINT ( 'NONE',  ( 116.0000000000000142, 0.000000000000000000, 0.000000000000000000 ) ) ;
#27630=CARTESIAN_POINT ( 'NONE',  ( 143.6324251345948824, -5.500000000000012434, -2.278174593052012309 ) ) ;
#27631=DIRECTION ( 'NONE',  ( 1.000000000000000000, 0.000000000000000000, 0.000000000000000000 ) ) ;
#27632=CARTESIAN_POINT ( 'NONE',  ( 139.5148502691896510, -3.535533905932725318, -3.535533905932725318 ) ) ;
#27633=ORIENTED_EDGE ( 'NONE', *, *, #26134, .F. ) ;
#27640=CARTESIAN_POINT ( 'NONE',  ( 130.0000000000000284, -60.00000000000001421, -3.000000000000002665 ) ) ;
#27641=EDGE_LOOP ( 'NONE', ( #19626, #14691, #22837, #14083 ) ) ;
#27642=ORIENTED_EDGE ( 'NONE', *, *, #7275, .T. ) ;
#27644=CARTESIAN_POINT ( 'NONE',  ( 144.0937500000000000, 6.000000000000005329, 2.485281374238585972 ) ) ;
#27649=ORIENTED_EDGE ( 'NONE', *, *, #19363, .F. ) ;
#27650=AXIS2_PLACEMENT_3D ( 'NONE', #15585, #21077, #16646 ) ;
#27651=LINE ( 'NONE', #23237, #2298 ) ;
#27653=DIRECTION ( 'NONE',  ( 0.000000000000000000, 1.000000000000000000, 0.000000000000000000 ) ) ;
#27656=CARTESIAN_POINT ( 'NONE',  ( 141.8288997308104058, 4.999999999999989342, -2.071067811865468400 ) ) ;
#27658=LINE ( 'NONE', #14204, #7912 ) ;
#27660=CARTESIAN_POINT ( 'NONE',  ( 135.0000000000000284, 0.000000000000000000, 0.000000000000000000 ) ) ;
#27666=( LENGTH_UNIT ( ) NAMED_UNIT ( * ) SI_UNIT ( .MILLI., .METRE. ) );
#27673=ORIENTED_EDGE ( 'NONE', *, *, #195, .F. ) ;
#27675=CARTESIAN_POINT ( 'NONE',  ( 137.8125000000000284, 4.242640687119298093, -4.242640687119298093 ) ) ;
#27678=CARTESIAN_POINT ( 'NONE',  ( 140.3437500000000284, -6.000000000000005329, -2.485281374238555774 ) ) ;
#27683=ORIENTED_EDGE ( 'NONE', *, *, #6677, .T. ) ;
#27689=DIRECTION ( 'NONE',  ( 1.000000000000000000, 0.000000000000000000, 0.000000000000000000 ) ) ;
#27692=FACE_OUTER_BOUND ( 'NONE', #7222, .T. ) ;
#27695=FACE_OUTER_BOUND ( 'NONE', #8349, .T. ) ;
#27701=CARTESIAN_POINT ( 'NONE',  ( 160.9613248654052029, -5.500000000000005329, 0.000000000000000000 ) ) ;
#27702=CARTESIAN_POINT ( 'NONE',  ( 135.0000000000000284, 1.949781249179022291, 5.142796231657420947 ) ) ;
#27712=CARTESIAN_POINT ( 'NONE',  ( 157.2187500000000284, 2.485281374238555774, -6.000000000000005329 ) ) ;
#27713=DIRECTION ( 'NONE',  ( 0.000000000000000000, -1.000000000000000000, 0.000000000000000000 ) ) ;
#27722=ORIENTED_EDGE ( 'NONE', *, *, #24886, .T. ) ;
#27725=AXIS2_PLACEMENT_3D ( 'NONE', #4066, #77, #9462 ) ;
#27728=ORIENTED_EDGE ( 'NONE', *, *, #9598, .T. ) ;
#27729=CARTESIAN_POINT ( 'NONE',  ( 136.0000000000000284, 1.347111479062088799E-15, 11.00000000000000355 ) ) ;
#27730=( LENGTH_UNIT ( ) NAMED_UNIT ( * ) SI_UNIT ( .MILLI., .METRE. ) );
#27736=FACE_OUTER_BOUND ( 'NONE', #10317, .T. ) ;
#27739=CARTESIAN_POINT ( 'NONE',  ( -0.05026229418827968254, -14.53482904599736791, 8.281231568825615952 ) ) ;
#27740=EDGE_LOOP ( 'NONE', ( #21037, #9507, #27595, #12468 ) ) ;
#27741=AXIS2_PLACEMENT_3D ( 'NONE', #16900, #13053, #12592 ) ;
#27745=CARTESIAN_POINT ( 'NONE',  ( 139.5000000000000284, -8.500000000000007105, -7.500000000000007105 ) ) ;
#27748=CYLINDRICAL_SURFACE ( 'NONE', #13843, 5.500000000000000000 ) ;
#27751=EDGE_LOOP ( 'NONE', ( #19574, #13097, #29689, #13367, #13765, #9189, #28025, #9521, #13998, #17115, #3805, #4975, #13459, #6428 ) ) ;
#27754=CARTESIAN_POINT ( 'NONE',  ( 150.4687500000000284, -2.485281374238585972, 6.000000000000005329 ) ) ;
#27764=FILL_AREA_STYLE ('',( #15860 ) ) ;
#27765=FILL_AREA_STYLE ('',( #12113 ) ) ;
#27766=VERTEX_POINT ( 'NONE', #1066 ) ;
#27768=CARTESIAN_POINT ( 'NONE',  ( 0.7617735382584472914, -15.57904714829914461, -7.971427046324570220 ) ) ;
#27775=ADVANCED_FACE ( 'NONE', ( #17379 ), #23607, .T. ) ;
#27777=CARTESIAN_POINT ( 'NONE',  ( -0.05236263670368471873, -9.947637363296282231, -4.619711369386857669 ) ) ;
#27782=ORIENTED_EDGE ( 'NONE', *, *, #27114, .F. ) ;
#27789=LINE ( 'NONE', #28250, #7401 ) ;
#27796=EDGE_LOOP ( 'NONE', ( #27842, #1929, #5490, #16514 ) ) ;
#27797=DIRECTION ( 'NONE',  ( 0.000000000000000000, 0.000000000000000000, -1.000000000000000000 ) ) ;
#27798=CARTESIAN_POINT ( 'NONE',  ( 135.8437500000000284, -6.000000000000005329, -2.485281374238555774 ) ) ;
#27800=CIRCLE ( 'NONE', #25851, 5.500000000000000000 ) ;
#27804=CARTESIAN_POINT ( 'NONE',  ( 0.000000000000000000, 2.081899558550501068E-15, 16.50000000000000355 ) ) ;
#27805=AXIS2_PLACEMENT_3D ( 'NONE', #3526, #29026, #26714 ) ;
#27807=CARTESIAN_POINT ( 'NONE',  ( 145.5788997308104342, -4.999999999999989342, 2.071067811865468400 ) ) ;
#27810=EDGE_CURVE ( 'NONE', #22119, #26506, #29153, .T. ) ;
#27818=AXIS2_PLACEMENT_3D ( 'NONE', #15925, #11462, #6338 ) ;
#27821=DIRECTION ( 'NONE',  ( 1.000000000000000000, 0.000000000000000000, 0.000000000000000000 ) ) ;
#27828=ORIENTED_EDGE ( 'NONE', *, *, #24562, .T. ) ;
#27830=CARTESIAN_POINT ( 'NONE',  ( 138.0937500000000568, 6.000000000000005329, 2.485281374238585972 ) ) ;
#27831=LINE ( 'NONE', #4339, #2793 ) ;
#27832=STYLED_ITEM ( 'NONE', ( #7997 ), #5167 ) ;
#27833=CARTESIAN_POINT ( 'NONE',  ( 136.5000000000000284, 6.000000000000005329, 0.000000000000000000 ) ) ;
#27835=ORIENTED_EDGE ( 'NONE', *, *, #14910, .T. ) ;
#27842=ORIENTED_EDGE ( 'NONE', *, *, #5312, .F. ) ;
#27845=DIRECTION ( 'NONE',  ( 1.000000000000000000, -0.000000000000000000, -0.000000000000000000 ) ) ;
#27846=CARTESIAN_POINT ( 'NONE',  ( 140.2643372958527266, -11.26433729585143340, -4.292342582647269644 ) ) ;
#27848=( BOUNDED_CURVE ( )  B_SPLINE_CURVE ( 2, ( #1244, #25199, #20166, #17885, #1407, #8315, #4162, #1716, #29515 ),
 .UNSPECIFIED., .F., .T. ) 
 B_SPLINE_CURVE_WITH_KNOTS ( ( 3, 2, 2, 2, 3 ),
 ( 0.1124999999999987121, 0.1187499999999989536, 0.1249999999999991951, 0.1312499999999994227, 0.1374999999999996780 ),
 .UNSPECIFIED. ) 
 CURVE ( )  GEOMETRIC_REPRESENTATION_ITEM ( )  RATIONAL_B_SPLINE_CURVE ( ( 1.000000000000016209, 0.9238795325112705292, 1.000000000000000000, 0.9238795325112867385, 1.000000000000000000, 0.9238795325112867385, 1.000000000000000000, 0.9238795325112900692, 0.9999999999999966693 ) ) 
 REPRESENTATION_ITEM ( '' )  );
#27857=( BOUNDED_CURVE ( )  B_SPLINE_CURVE ( 2, ( #4760, #16036, #23224, #25333, #4308, #23069, #21065, #6765, #16186 ),
 .UNSPECIFIED., .F., .T. ) 
 B_SPLINE_CURVE_WITH_KNOTS ( ( 3, 2, 2, 2, 3 ),
 ( 0.3374999999999998557, 0.3437500000000000555, 0.3500000000000003109, 0.3562500000000005662, 0.3625000000000007661 ),
 .UNSPECIFIED. ) 
 CURVE ( )  GEOMETRIC_REPRESENTATION_ITEM ( )  RATIONAL_B_SPLINE_CURVE ( ( 1.000000000000001998, 0.9238795325112847401, 1.000000000000000000, 0.9238795325112867385, 1.000000000000000000, 0.9238795325112867385, 1.000000000000000000, 0.9238795325112773016, 1.000000000000009548 ) ) 
 REPRESENTATION_ITEM ( '' )  );
#27860=CARTESIAN_POINT ( 'NONE',  ( 150.3898502691896510, 3.535533905932725318, -3.535533905932725318 ) ) ;
#27861=DIRECTION ( 'NONE',  ( 0.000000000000000000, 0.000000000000000000, -1.000000000000000000 ) ) ;
#27864=CARTESIAN_POINT ( 'NONE',  ( 156.0000000000000284, 6.000000000000005329, 0.000000000000000000 ) ) ;
#27869=CARTESIAN_POINT ( 'NONE',  ( -0.5000000000000004441, -9.500000000000008882, 5.000000000000004441 ) ) ;
#27871=CARTESIAN_POINT ( 'NONE',  ( 158.3437500000000568, -6.000000000000005329, -2.485281374238555774 ) ) ;
#27875=DIRECTION ( 'NONE',  ( -1.000000000000000000, -0.000000000000000000, -0.000000000000000000 ) ) ;
#27877=ORIENTED_EDGE ( 'NONE', *, *, #19553, .T. ) ;
#27883=EDGE_CURVE ( 'NONE', #476, #25526, #27979, .T. ) ;
#27885=ORIENTED_EDGE ( 'NONE', *, *, #19430, .F. ) ;
#27886=DIRECTION ( 'NONE',  ( 0.000000000000000000, -1.000000000000000000, 0.000000000000000000 ) ) ;
#27895=CARTESIAN_POINT ( 'NONE',  ( 161.7336002691896510, -4.999999999999989342, 2.071067811865468400 ) ) ;
#27902=ORIENTED_EDGE ( 'NONE', *, *, #19488, .T. ) ;
#27906=CARTESIAN_POINT ( 'NONE',  ( 147.9375000000000284, -4.242640687119298093, -4.242640687119298093 ) ) ;
#27911=ORIENTED_EDGE ( 'NONE', *, *, #16946, .T. ) ;
#27912=FACE_OUTER_BOUND ( 'NONE', #18166, .T. ) ;
#27913=CIRCLE ( 'NONE', #14709, 5.500000000000000000 ) ;
#27917=ADVANCED_FACE ( 'NONE', ( #11391 ), #15861, .F. ) ;
#27923=PLANE ( 'NONE',  #158 ) ;
#27928=CARTESIAN_POINT ( 'NONE',  ( 161.0000000000000284, 0.000000000000000000, -5.500000000000000000 ) ) ;
#27932=ORIENTED_EDGE ( 'NONE', *, *, #18299, .F. ) ;
#27934=CIRCLE ( 'NONE', #13766, 10.49999999999998224 ) ;
#27935=DIRECTION ( 'NONE',  ( 0.000000000000000000, 0.000000000000000000, -1.000000000000000000 ) ) ;
#27936=CIRCLE ( 'NONE', #5852, 10.49999999999999645 ) ;
#27942=PLANE ( 'NONE',  #8196 ) ;
#27945=VERTEX_POINT ( 'NONE', #18594 ) ;
#27946=ORIENTED_EDGE ( 'NONE', *, *, #14847, .F. ) ;
#27947=CARTESIAN_POINT ( 'NONE',  ( 135.2812500000000284, 2.485281374238585972, 6.000000000000005329 ) ) ;
#27957=CARTESIAN_POINT ( 'NONE',  ( 142.8601497308104058, -3.535533905932725318, -3.535533905932725318 ) ) ;
#27961=DIRECTION ( 'NONE',  ( 1.000000000000000000, 1.067522139062651904E-16, -0.000000000000000000 ) ) ;
#27968=SURFACE_STYLE_USAGE ( .BOTH. , #13911 ) ;
#27973=CARTESIAN_POINT ( 'NONE',  ( 116.0000000000000142, 0.000000000000000000, -5.500000000000000000 ) ) ;
#27977=CARTESIAN_POINT ( 'NONE',  ( 140.5312500000000284, -2.485281374238556218, -6.000000000000005329 ) ) ;
#27979=CIRCLE ( 'NONE', #5409, 1.000000000000000888 ) ;
#27980=DIRECTION ( 'NONE',  ( 0.000000000000000000, 0.000000000000000000, -1.000000000000000000 ) ) ;
#27981=CARTESIAN_POINT ( 'NONE',  ( 133.8750000000000284, 0.000000000000000000, 6.000000000000005329 ) ) ;
#27982=DIRECTION ( 'NONE',  ( -1.000000000000000000, 0.000000000000000000, 0.000000000000000000 ) ) ;
#27983=VERTEX_POINT ( 'NONE', #10529 ) ;
#27984=EDGE_CURVE ( 'NONE', #8808, #30157, #26769, .T. ) ;
#27986=VECTOR ( 'NONE', #26009, 1000.000000000000000 ) ;
#27990=( BOUNDED_CURVE ( )  B_SPLINE_CURVE ( 2, ( #1062, #26843, #3505, #24110, #21821, #1980, #6276, #13541, #1513 ),
 .UNSPECIFIED., .F., .F. ) 
 B_SPLINE_CURVE_WITH_KNOTS ( ( 3, 2, 2, 2, 3 ),
 ( 0.1374999999999996780, 0.1437499999999998779, 0.1500000000000001332, 0.1562500000000003886, 0.1625000000000006162 ),
 .UNSPECIFIED. ) 
 CURVE ( )  GEOMETRIC_REPRESENTATION_ITEM ( )  RATIONAL_B_SPLINE_CURVE ( ( 1.000000000000003997, 0.9238795325112826307, 1.000000000000000000, 0.9238795325112867385, 1.000000000000000000, 0.9238795325112867385, 1.000000000000000000, 0.9238795325112793000, 1.000000000000007327 ) ) 
 REPRESENTATION_ITEM ( '' )  );
#27991=DIRECTION ( 'NONE',  ( 1.000000000000000000, 0.000000000000000000, 0.000000000000000000 ) ) ;
#27997=CARTESIAN_POINT ( 'NONE',  ( 140.1944936379390754, -11.19449363793808239, -4.371599137206734653 ) ) ;
#28002=CARTESIAN_POINT ( 'NONE',  ( 140.4148756743437048, -9.242664784350015594, -7.657040506132355873 ) ) ;
#28010=CARTESIAN_POINT ( 'NONE',  ( 144.6636751345948255, 0.000000000000000000, 5.500000000000005329 ) ) ;
#28011=STYLED_ITEM ( 'NONE', ( #11643 ), #11474 ) ;
#28012=CARTESIAN_POINT ( 'NONE',  ( 158.0625000000000284, -4.242640687119298093, 4.242640687119298093 ) ) ;
#28013=( LENGTH_UNIT ( ) NAMED_UNIT ( * ) SI_UNIT ( .MILLI., .METRE. ) );
#28015=CARTESIAN_POINT ( 'NONE',  ( -19.49999999999998224, -54.99999999999990763, 8.000000000000007105 ) ) ;
#28020=CARTESIAN_POINT ( 'NONE',  ( 148.7812500000000284, 2.485281374238585972, 6.000000000000005329 ) ) ;
#28023=EDGE_CURVE ( 'NONE', #16823, #22218, #16297, .T. ) ;
#28025=ORIENTED_EDGE ( 'NONE', *, *, #19956, .T. ) ;
#28026=VERTEX_POINT ( 'NONE', #19301 ) ;
#28029=EDGE_CURVE ( 'NONE', #19511, #25088, #28623, .T. ) ;
#28033=ORIENTED_EDGE ( 'NONE', *, *, #168, .T. ) ;
#28036=CARTESIAN_POINT ( 'NONE',  ( 158.1413997308104058, 2.071067811865468400, -4.999999999999989342 ) ) ;
#28042=MECHANICAL_DESIGN_GEOMETRIC_PRESENTATION_REPRESENTATION('',(#101),#14580);
#28049=CARTESIAN_POINT ( 'NONE',  ( 134.9999999999997158, -6.982120021894168360, 8.500000000000007105 ) ) ;
#28064=CARTESIAN_POINT ( 'NONE',  ( 151.5000000000000284, 6.000000000000005329, 0.000000000000000000 ) ) ;
#28070=ORIENTED_EDGE ( 'NONE', *, *, #11726, .F. ) ;
#28071=CARTESIAN_POINT ( 'NONE',  ( 158.8988248654052313, 3.889087296526011706, 3.889087296526011706 ) ) ;
#28076=CARTESIAN_POINT ( 'NONE',  ( 153.3824251345948539, 5.500000000000012434, 2.278174593052012309 ) ) ;
#28082=CARTESIAN_POINT ( 'NONE',  ( 125.0000000000000568, -55.00000000000000711, 8.000000000000007105 ) ) ;
#28083=DIRECTION ( 'NONE',  ( 1.000000000000000000, 1.674905425081055330E-15, 0.000000000000000000 ) ) ;
#28087=ORIENTED_EDGE ( 'NONE', *, *, #16303, .T. ) ;
#28089=CARTESIAN_POINT ( 'NONE',  ( 0.2151077267762193934, -15.80992884008447241, 7.511547624681091051 ) ) ;
#28090=CARTESIAN_POINT ( 'NONE',  ( 143.4449251345948539, -5.500000000000012434, 2.278174593052012309 ) ) ;
#28092=COLOUR_RGB ( '', 0.31764706, 0.68627451, 0.89019608) ;
#28093=VERTEX_POINT ( 'NONE', #12554 ) ;
#28098=CARTESIAN_POINT ( 'NONE',  ( 156.6636751345948255, 0.000000000000000000, 5.500000000000005329 ) ) ;
#28104=CARTESIAN_POINT ( 'NONE',  ( 136.3125000000000284, 4.242640687119298093, -4.242640687119298093 ) ) ;
#28107=CARTESIAN_POINT ( 'NONE',  ( 161.0000000000000284, 3.467572205841706889, 4.269185284954735593 ) ) ;
#28115=CIRCLE ( 'NONE', #18836, 2.000000000000000000 ) ;
#28116=CARTESIAN_POINT ( 'NONE',  ( 144.1726497308104058, -5.000000000000004441, 0.000000000000000000 ) ) ;
#28121=CYLINDRICAL_SURFACE ( 'NONE', #3735, 1.000000000000000888 ) ;
#28125=SURFACE_STYLE_FILL_AREA ( #4927 ) ;
#28126=DIRECTION ( 'NONE',  ( 6.938893903907222067E-15, -1.000000000000000000, 0.000000000000000000 ) ) ;
#28129=FACE_OUTER_BOUND ( 'NONE', #5916, .T. ) ;
#28130=( BOUNDED_CURVE ( )  B_SPLINE_CURVE ( 2, ( #27552, #3908, #24499, #1619, #8213, #29576, #20366, #10871, #6370 ),
 .UNSPECIFIED., .F., .T. ) 
 B_SPLINE_CURVE_WITH_KNOTS ( ( 3, 2, 2, 2, 3 ),
 ( 0.3625000000000007661, 0.3687500000000005773, 0.3750000000000003331, 0.3812500000000000888, 0.3874999999999999001 ),
 .UNSPECIFIED. ) 
 CURVE ( )  GEOMETRIC_REPRESENTATION_ITEM ( )  RATIONAL_B_SPLINE_CURVE ( ( 0.9999999999999905631, 0.9238795325112961754, 1.000000000000000000, 0.9238795325112867385, 1.000000000000000000, 0.9238795325112867385, 1.000000000000000000, 0.9238795325112880708, 0.9999999999999986677 ) ) 
 REPRESENTATION_ITEM ( '' )  );
#28134=CARTESIAN_POINT ( 'NONE',  ( 141.8437500000000568, -6.000000000000005329, -2.485281374238556218 ) ) ;
#28138=EDGE_CURVE ( 'NONE', #16010, #15961, #22350, .T. ) ;
#28139=CARTESIAN_POINT ( 'NONE',  ( 132.5625000000000284, -4.242640687119298093, 4.242640687119298093 ) ) ;
#28141=CLOSED_SHELL ( 'NONE', ( #1185, #15198, #27507, #3859, #5179, #11474, #3817, #12843, #30120, #6884, #14454, #979, #17033, #27288, #21334, #4571, #25177, #27262, #3790, #27917, #3422, #24848, #23960, #10017, #15922, #27156, #5546, #3263, #12368, #23889, #13558, #3252, #2852, #16057, #26910, #25858, #14331, #6354, #23989, #29379, #7443, #16776, #943, #10296, #328, #22508, #7471, #19286, #9, #19292, #13276, #27197, #21849, #139, #29410, #13311, #19722, #18571, #16674, #7065, #10399, #16810, #29092, #14513, #29627, #5900, #98, #6324, #29496, #5129, #10870, #25921, #23110, #15738, #28636, #18363, #18162, #7957, #13310, #9576, #25993, #2364, #13845, #12132, #10259, #4906, #5167, #7131, #24129, #2220, #7737, #20695, #2508, #22155, #6788, #16651, #6089, #23581, #3883, #9279, #26664, #27775, #9723, #20155, #4379, #27336, #169, #16033, #13451, #24351, #25626, #30341, #15893, #790, #17004, #10628, #28571, #21199, #29191, #10909, #21405, #12964, #11763, #23460, #11827, #6379, #3187, #7634, #26651, #19323, #18543, #9541, #26570, #21086, #19781, #29265, #29201, #17807, #26879, #28887, #20530, #3948, #24911, #22956, #18677, #13286, #23035, #14226, #8474, #9076, #28363, #25892, #24286, #6817, #26361, #19562, #18401, #7572, #11137, #29226, #56, #8743, #29340, #16818, #2179, #18190, #16643, #25504, #11403, #24453, #14617, #8665, #780, #8107, #12436, #20643, #9473, #26691, #5037, #23821, #26163, #26222, #4202, #22999, #12893, #10530, #19821, #25998, #7544, #7074 ) ) ;
#28143=ORIENTED_EDGE ( 'NONE', *, *, #16540, .T. ) ;
#28149=CARTESIAN_POINT ( 'NONE',  ( 154.7886751345948255, 5.500000000000005329, 0.000000000000000000 ) ) ;
#28151=DIRECTION ( 'NONE',  ( 0.000000000000000000, -1.000000000000000000, -0.000000000000000000 ) ) ;
#28154=FACE_OUTER_BOUND ( 'NONE', #7768, .T. ) ;
#28160=DIRECTION ( 'NONE',  ( 0.000000000000000000, 8.881784197001252323E-16, 1.000000000000000000 ) ) ;
#28162=SURFACE_STYLE_USAGE ( .BOTH. , #14105 ) ;
#28163=CARTESIAN_POINT ( 'NONE',  ( 143.9211002691896510, -4.999999999999989342, -2.071067811865468400 ) ) ;
#28166=CARTESIAN_POINT ( 'NONE',  ( 158.4375000000000284, -4.242640687119298093, -4.242640687119298093 ) ) ;
#28167=SURFACE_STYLE_USAGE ( .BOTH. , #4827 ) ;
#28172=ORIENTED_EDGE ( 'NONE', *, *, #3158, .T. ) ;
#28173=CARTESIAN_POINT ( 'NONE',  ( 147.5625000000000284, -4.242640687119298093, 4.242640687119298093 ) ) ;
#28174=CARTESIAN_POINT ( 'NONE',  ( -4.999999999999990230, -24.99999999999999289, 7.500000000000007105 ) ) ;
#28180=COLOUR_RGB ( '', 0.72549020, 0.75294118, 0.79215686) ;
#28182=CARTESIAN_POINT ( 'NONE',  ( 140.0000000000000284, -54.99999999999990763, 8.000000000000007105 ) ) ;
#28183=CARTESIAN_POINT ( 'NONE',  ( 156.1726497308104058, -5.000000000000004441, 0.000000000000000000 ) ) ;
#28188=CARTESIAN_POINT ( 'NONE',  ( 147.0863248654052313, 0.000000000000000000, 5.500000000000005329 ) ) ;
#28191=AXIS2_PLACEMENT_3D ( 'NONE', #4529, #8997, #2239 ) ;
#28194=CARTESIAN_POINT ( 'NONE',  ( 116.0000000000000142, 0.000000000000000000, 0.000000000000000000 ) ) ;
#28198=CARTESIAN_POINT ( 'NONE',  ( 161.2648502691896510, 3.535533905932725318, 3.535533905932752852 ) ) ;
#28199=CARTESIAN_POINT ( 'NONE',  ( 0.2111556581636949148, -15.49108841857535168, 8.141471415412047108 ) ) ;
#28203=DIRECTION ( 'NONE',  ( 1.000000000000000000, 0.000000000000000000, 0.000000000000000000 ) ) ;
#28208=TOROIDAL_SURFACE ( 'NONE', #15993, 10.49999999999999822, 0.5000000000000000000 ) ;
#28211=EDGE_CURVE ( 'NONE', #2390, #17791, #13975, .T. ) ;
#28214=CARTESIAN_POINT ( 'NONE',  ( 124.9999999999999432, -65.50000000000000000, 8.000000000000007105 ) ) ;
#28217=CARTESIAN_POINT ( 'NONE',  ( 151.0312500000000568, -2.485281374238555774, -6.000000000000005329 ) ) ;
#28218=VERTEX_POINT ( 'NONE', #3739 ) ;
#28226=CARTESIAN_POINT ( 'NONE',  ( 131.5163997308104626, 4.999999999999989342, 2.071067811865468400 ) ) ;
#28227=EDGE_LOOP ( 'NONE', ( #4044, #3865, #18766, #8399 ) ) ;
#28228=VECTOR ( 'NONE', #19599, 1000.000000000000000 ) ;
#28235=EDGE_CURVE ( 'NONE', #29963, #18576, #20217, .T. ) ;
#28239=CARTESIAN_POINT ( 'NONE',  ( 134.9999999999992895, -6.982120021884476557, -8.500000000000007105 ) ) ;
#28243=CARTESIAN_POINT ( 'NONE',  ( 8.673617379884035472E-16, -16.43939393939395188, 5.999693900976774685 ) ) ;
#28249=DIRECTION ( 'NONE',  ( -0.000000000000000000, 1.000000000000000000, 0.000000000000000000 ) ) ;
#28250=CARTESIAN_POINT ( 'NONE',  ( 116.0000000000000142, 6.735557395310442023E-16, 5.500000000000000000 ) ) ;
#28253=CARTESIAN_POINT ( 'NONE',  ( 140.7113248654052313, 5.500000000000005329, 0.000000000000000000 ) ) ;
#28255=ORIENTED_EDGE ( 'NONE', *, *, #9466, .T. ) ;
#28256=CARTESIAN_POINT ( 'NONE',  ( 152.3363248654052029, 0.000000000000000000, -5.500000000000005329 ) ) ;
#28257=CARTESIAN_POINT ( 'NONE',  ( 136.9687500000000000, -2.485281374238585972, 6.000000000000005329 ) ) ;
#28258=CIRCLE ( 'NONE', #22889, 30.00000000000000000 ) ;
#28261=CARTESIAN_POINT ( 'NONE',  ( 144.1011751345948539, 3.889087296526011706, -3.889087296526011706 ) ) ;
#28263=CARTESIAN_POINT ( 'NONE',  ( 8.673617379884035472E-16, -14.14213562373095634, 8.500000000000007105 ) ) ;
#28264=DIRECTION ( 'NONE',  ( 1.000000000000000000, -0.000000000000000000, -0.000000000000000000 ) ) ;
#28265=CARTESIAN_POINT ( 'NONE',  ( 144.4538997308104626, -2.071067811865468400, -4.999999999999989342 ) ) ;
#28269=CARTESIAN_POINT ( 'NONE',  ( 156.6636751345948255, 0.000000000000000000, 5.500000000000005329 ) ) ;
#28270=DIRECTION ( 'NONE',  ( 0.000000000000000000, 0.000000000000000000, -1.000000000000000000 ) ) ;
#28272=EDGE_CURVE ( 'NONE', #24844, #12427, #6427, .T. ) ;
#28273=AXIS2_PLACEMENT_3D ( 'NONE', #23874, #3409, #24169 ) ;
#28275=AXIS2_PLACEMENT_3D ( 'NONE', #25979, #23839, #2774 ) ;
#28278=EDGE_CURVE ( 'NONE', #6130, #13456, #22148, .T. ) ;
#28283=CARTESIAN_POINT ( 'NONE',  ( 139.5937500000000568, 6.000000000000005329, 2.485281374238585972 ) ) ;
#28285=CARTESIAN_POINT ( 'NONE',  ( 142.5074251345948255, 2.278174593051965235, -5.500000000000058620 ) ) ;
#28286=CARTESIAN_POINT ( 'NONE',  ( 133.9687500000000284, -2.485281374238585972, 6.000000000000005329 ) ) ;
#28288=VERTEX_POINT ( 'NONE', #18520 ) ;
#28289=AXIS2_PLACEMENT_3D ( 'NONE', #1517, #22587, #6280 ) ;
#28292=ORIENTED_EDGE ( 'NONE', *, *, #20411, .F. ) ;
#28295=CARTESIAN_POINT ( 'NONE',  ( -20.99999999999998224, -25.00000000000010658, 4.000000000000003553 ) ) ;
#28300=CARTESIAN_POINT ( 'NONE',  ( 139.5000000000000000, -9.165151389911669000, 8.000000000000007105 ) ) ;
#28305=EDGE_CURVE ( 'NONE', #11174, #6130, #28485, .T. ) ;
#28313=CIRCLE ( 'NONE', #12194, 11.00000000000000355 ) ;
#28318=CARTESIAN_POINT ( 'NONE',  ( 160.5000000000000284, 6.000000000000005329, 0.000000000000000000 ) ) ;
#28324=CARTESIAN_POINT ( 'NONE',  ( 152.0625000000000568, -4.242640687119298093, 4.242640687119298093 ) ) ;
#28326=AXIS2_PLACEMENT_3D ( 'NONE', #13944, #16691, #4961 ) ;
#28330=VERTEX_POINT ( 'NONE', #28300 ) ;
#28331=ORIENTED_EDGE ( 'NONE', *, *, #2719, .F. ) ;
#28333=VECTOR ( 'NONE', #12879, 1000.000000000000000 ) ;
#28336=CARTESIAN_POINT ( 'NONE',  ( 153.8288997308104058, 4.999999999999989342, -2.071067811865468400 ) ) ;
#28339=DIRECTION ( 'NONE',  ( 0.000000000000000000, 0.000000000000000000, -1.000000000000000000 ) ) ;
#28341=EDGE_CURVE ( 'NONE', #3216, #6343, #29878, .T. ) ;
#28342=CARTESIAN_POINT ( 'NONE',  ( 144.0863248654052313, 0.000000000000000000, 5.500000000000005329 ) ) ;
#28349=CARTESIAN_POINT ( 'NONE',  ( 155.7336002691896226, -4.999999999999989342, 2.071067811865468400 ) ) ;
#28350=DIRECTION ( 'NONE',  ( -1.000000000000000000, -1.067522139062651411E-16, 0.000000000000000000 ) ) ;
#28351=ORIENTED_EDGE ( 'NONE', *, *, #7338, .F. ) ;
#28358=EDGE_LOOP ( 'NONE', ( #6378, #27524, #19580, #15777 ) ) ;
#28359=CARTESIAN_POINT ( 'NONE',  ( 146.1636751345948255, 0.000000000000000000, 5.500000000000005329 ) ) ;
#28361=VERTEX_POINT ( 'NONE', #28449 ) ;
#28363=ADVANCED_FACE ( 'NONE', ( #26301 ), #10042, .T. ) ;
#28367=UNCERTAINTY_MEASURE_WITH_UNIT (LENGTH_MEASURE( 1.000000000000000082E-05 ), #26791, 'distance_accuracy_value', 'NONE');
#28369=FILL_AREA_STYLE ('',( #6890 ) ) ;
#28372=CARTESIAN_POINT ( 'NONE',  ( 131.4226497308104058, 5.000000000000004441, 0.000000000000000000 ) ) ;
#28375=CYLINDRICAL_SURFACE ( 'NONE', #10101, 0.5000000000000004441 ) ;
#28376=CYLINDRICAL_SURFACE ( 'NONE', #4979, 5.500000000000000000 ) ;
#28380=DIRECTION ( 'NONE',  ( 1.000000000000000000, 0.000000000000000000, 0.000000000000000000 ) ) ;
#28382=CARTESIAN_POINT ( 'NONE',  ( 162.0000000000000284, 0.000000000000000000, -11.00000000000000355 ) ) ;
#28383=UNCERTAINTY_MEASURE_WITH_UNIT (LENGTH_MEASURE( 1.000000000000000082E-05 ), #314, 'distance_accuracy_value', 'NONE');
#28391=CARTESIAN_POINT ( 'NONE',  ( 135.0525775163646074, 3.054031077158521068, -4.724143515893503675 ) ) ;
#28396=CIRCLE ( 'NONE', #17644, 0.5000000000000000000 ) ;
#28399=MECHANICAL_DESIGN_GEOMETRIC_PRESENTATION_REPRESENTATION('',(#18137),#29381);
#28400=CARTESIAN_POINT ( 'NONE',  ( 141.0863248654052313, 0.000000000000000000, 5.500000000000005329 ) ) ;
#28402=EDGE_LOOP ( 'NONE', ( #10220, #26465, #9771, #17404 ) ) ;
#28404=CARTESIAN_POINT ( 'NONE',  ( 133.9687500000000284, -2.485281374238585972, 6.000000000000005329 ) ) ;
#28412=CARTESIAN_POINT ( 'NONE',  ( -0.5000000000000014433, -10.00000000000000711, 4.414213562373099364 ) ) ;
#28414=CARTESIAN_POINT ( 'NONE',  ( 138.5476497308104058, 0.000000000000000000, -5.000000000000004441 ) ) ;
#28422=CARTESIAN_POINT ( 'NONE',  ( 154.3199251345948539, -2.278174593051950136, -5.500000000000074607 ) ) ;
#28424=( GEOMETRIC_REPRESENTATION_CONTEXT ( 3 ) GLOBAL_UNCERTAINTY_ASSIGNED_CONTEXT ( ( #13044 ) ) GLOBAL_UNIT_ASSIGNED_CONTEXT ( ( #10235, #21302, #26189 ) ) REPRESENTATION_CONTEXT ( 'NONE', 'WORKASPACE' ) );
#28432=CARTESIAN_POINT ( 'NONE',  ( 138.3675748654052029, -5.500000000000012434, 2.278174593052012309 ) ) ;
#28433=CARTESIAN_POINT ( 'NONE',  ( 160.6726497308104058, -5.000000000000004441, 0.000000000000000000 ) ) ;
#28436=EDGE_CURVE ( 'NONE', #22235, #11502, #21864, .T. ) ;
#28437=COLOUR_RGB ( '', 0.40784314, 0.44705882, 0.49803922) ;
#28441=ORIENTED_EDGE ( 'NONE', *, *, #19582, .T. ) ;
#28444=DIRECTION ( 'NONE',  ( -1.000000000000000000, -0.000000000000000000, 0.000000000000000000 ) ) ;
#28449=CARTESIAN_POINT ( 'NONE',  ( -1.000000000000000888, 10.00000000000000888, 3.000000000000002665 ) ) ;
#28451=CARTESIAN_POINT ( 'NONE',  ( 124.9999999999999432, -65.50000000000000000, -7.500000000000007105 ) ) ;
#28458=STYLED_ITEM ( 'NONE', ( #23536 ), #27507 ) ;
#28460=CARTESIAN_POINT ( 'NONE',  ( 145.2113248654052313, 5.500000000000005329, 0.000000000000000000 ) ) ;
#28463=CARTESIAN_POINT ( 'NONE',  ( 145.3273502691896510, -5.000000000000004441, 0.000000000000000000 ) ) ;
#28465=CARTESIAN_POINT ( 'NONE',  ( 159.0000000000000284, 6.000000000000005329, 0.000000000000000000 ) ) ;
#28466=LINE ( 'NONE', #7434, #27071 ) ;
#28471=ORIENTED_EDGE ( 'NONE', *, *, #22087, .T. ) ;
#28472=CARTESIAN_POINT ( 'NONE',  ( 148.1250000000000284, 0.000000000000000000, -6.000000000000005329 ) ) ;
#28475=DIRECTION ( 'NONE',  ( 1.000000000000000000, -0.000000000000000000, -0.000000000000000000 ) ) ;
#28476=UNCERTAINTY_MEASURE_WITH_UNIT (LENGTH_MEASURE( 1.000000000000000082E-05 ), #14760, 'distance_accuracy_value', 'NONE');
#28485=CIRCLE ( 'NONE', #2982, 10.49999999999999645 ) ;
#28490=CARTESIAN_POINT ( 'NONE',  ( 153.2663997308103774, -4.999999999999989342, -2.071067811865468400 ) ) ;
#28493=DIRECTION ( 'NONE',  ( 1.000000000000000000, 0.000000000000000000, 0.000000000000000000 ) ) ;
#28501=CARTESIAN_POINT ( 'NONE',  ( 155.1711002691897079, 4.999999999999989342, 2.071067811865468400 ) ) ;
#28504=LINE ( 'NONE', #7330, #23242 ) ;
#28515=EDGE_LOOP ( 'NONE', ( #19946, #11456, #23195, #11225, #29023, #25382 ) ) ;
#28528=CARTESIAN_POINT ( 'NONE',  ( -4.999999999999886313, -71.00000000000002842, -5.000000000000004441 ) ) ;
#28530=CARTESIAN_POINT ( 'NONE',  ( 116.0000000000000142, 0.000000000000000000, 0.000000000000000000 ) ) ;
#28532=CYLINDRICAL_SURFACE ( 'NONE', #17104, 5.500000000000000000 ) ;
#28536=CIRCLE ( 'NONE', #15346, 1.000000000000000000 ) ;
#28545=( NAMED_UNIT ( * ) SI_UNIT ( $, .STERADIAN. ) SOLID_ANGLE_UNIT ( ) );
#28548=EDGE_CURVE ( 'NONE', #13349, #13602, #21175, .T. ) ;
#28551=CARTESIAN_POINT ( 'NONE',  ( 134.8273502691896510, -5.000000000000004441, 0.000000000000000000 ) ) ;
#28552=ORIENTED_EDGE ( 'NONE', *, *, #23526, .F. ) ;
#28560=CARTESIAN_POINT ( 'NONE',  ( 139.5000000000000284, -9.165151389911669000, -8.000000000000007105 ) ) ;
#28561=CARTESIAN_POINT ( 'NONE',  ( 141.0788997308104058, -4.999999999999989342, 2.071067811865468400 ) ) ;
#28562=CARTESIAN_POINT ( 'NONE',  ( 137.7113248654052029, 5.500000000000005329, 0.000000000000000000 ) ) ;
#28566=( BOUNDED_CURVE ( )  B_SPLINE_CURVE ( 2, ( #10281, #12457, #15197, #27430, #20094, #6397, #6106, #18266, #24981 ),
 .UNSPECIFIED., .F., .T. ) 
 B_SPLINE_CURVE_WITH_KNOTS ( ( 3, 2, 2, 2, 3 ),
 ( 0.9124999999999995337, 0.9187499999999997335, 0.9250000000000000444, 0.9312500000000002442, 0.9375000000000004441 ),
 .UNSPECIFIED. ) 
 CURVE ( )  GEOMETRIC_REPRESENTATION_ITEM ( )  RATIONAL_B_SPLINE_CURVE ( ( 1.000000000000005329, 0.9238795325112812984, 1.000000000000000000, 0.9238795325112867385, 1.000000000000000000, 0.9238795325112867385, 1.000000000000000000, 0.9238795325112812984, 1.000000000000005329 ) ) 
 REPRESENTATION_ITEM ( '' )  );
#28569=CARTESIAN_POINT ( 'NONE',  ( -4.999999999999990230, -55.00000000000002132, 4.000000000000003553 ) ) ;
#28570=ORIENTED_EDGE ( 'NONE', *, *, #22214, .F. ) ;
#28571=ADVANCED_FACE ( 'NONE', ( #10973 ), #29521, .F. ) ;
#28575=STYLED_ITEM ( 'NONE', ( #15824 ), #13685 ) ;
#28577=ORIENTED_EDGE ( 'NONE', *, *, #2646, .T. ) ;
#28579=CARTESIAN_POINT ( 'NONE',  ( 136.4062500000000284, 6.000000000000005329, -2.485281374238556218 ) ) ;
#28583=CARTESIAN_POINT ( 'NONE',  ( 161.4226497308104058, 5.000000000000004441, 0.000000000000000000 ) ) ;
#28586=ORIENTED_EDGE ( 'NONE', *, *, #21254, .F. ) ;
#28589=FACE_OUTER_BOUND ( 'NONE', #5543, .T. ) ;
#28590=LINE ( 'NONE', #16534, #17163 ) ;
#28594=CARTESIAN_POINT ( 'NONE',  ( 116.0000000000000142, 0.000000000000000000, 0.000000000000000000 ) ) ;
#28604=CARTESIAN_POINT ( 'NONE',  ( 142.7023502691896510, 0.000000000000000000, -5.000000000000004441 ) ) ;
#28606=CARTESIAN_POINT ( 'NONE',  ( 151.4062500000000284, 6.000000000000005329, -2.485281374238556218 ) ) ;
#28609=MECHANICAL_DESIGN_GEOMETRIC_PRESENTATION_REPRESENTATION('',(#10514),#19333);
#28614=CARTESIAN_POINT ( 'NONE',  ( 151.3125000000000568, 4.242640687119298093, -4.242640687119298093 ) ) ;
#28619=VERTEX_POINT ( 'NONE', #10822 ) ;
#28623=LINE ( 'NONE', #19732, #11370 ) ;
#28624=DIRECTION ( 'NONE',  ( 1.000000000000000000, 0.000000000000000000, 0.000000000000000000 ) ) ;
#28625=DIRECTION ( 'NONE',  ( -0.000000000000000000, -0.000000000000000000, -1.000000000000000000 ) ) ;
#28626=CARTESIAN_POINT ( 'NONE',  ( 134.5000410784367944, -6.964617708436220411, 8.000000000000007105 ) ) ;
#28630=CARTESIAN_POINT ( 'NONE',  ( 134.9999999999999716, 4.954201571808754423, 2.980857315194011203 ) ) ;
#28631=CARTESIAN_POINT ( 'NONE',  ( 149.2425748654052029, -2.278174593052245012, -5.499999999999781508 ) ) ;
#28636=ADVANCED_FACE ( 'NONE', ( #3705 ), #1249, .F. ) ;
#28639=CARTESIAN_POINT ( 'NONE',  ( 158.1711002691896510, 4.999999999999989342, 2.071067811865468400 ) ) ;
#28644=DIRECTION ( 'NONE',  ( 1.000000000000000000, -0.000000000000000000, -0.000000000000000000 ) ) ;
#28646=DIRECTION ( 'NONE',  ( -0.2768592823360735977, 0.4367774878841475528, -0.8559055811606602893 ) ) ;
#28649=CARTESIAN_POINT ( 'NONE',  ( -0.05795336459416459973, -14.59255675236215666, -8.264483820923475221 ) ) ;
#28651=ORIENTED_EDGE ( 'NONE', *, *, #13614, .T. ) ;
#28653=ORIENTED_EDGE ( 'NONE', *, *, #20777, .T. ) ;
#28661=CARTESIAN_POINT ( 'NONE',  ( 131.6101497308104342, 3.535533905932725318, 3.535533905932725318 ) ) ;
#28662=AXIS2_PLACEMENT_3D ( 'NONE', #12635, #15236, #22134 ) ;
#28672=DIRECTION ( 'NONE',  ( 0.000000000000000000, 0.000000000000000000, 1.000000000000000000 ) ) ;
#28678=MECHANICAL_DESIGN_GEOMETRIC_PRESENTATION_REPRESENTATION('',(#6624),#8596);
#28680=ORIENTED_EDGE ( 'NONE', *, *, #195, .T. ) ;
#28682=CARTESIAN_POINT ( 'NONE',  ( 0.7669223171414760731, -15.58766199952930620, 7.954545454545462135 ) ) ;
#28688=AXIS2_PLACEMENT_3D ( 'NONE', #29714, #9144, #18385 ) ;
#28689=CARTESIAN_POINT ( 'NONE',  ( 136.0000000000000284, 0.000000000000000000, 0.000000000000000000 ) ) ;
#28695=CARTESIAN_POINT ( 'NONE',  ( 160.5000000000000284, 6.000000000000005329, 0.000000000000000000 ) ) ;
#28699=CYLINDRICAL_SURFACE ( 'NONE', #9830, 5.500000000000000000 ) ;
#28701=EDGE_CURVE ( 'NONE', #29595, #12702, #17259, .T. ) ;
#28702=CARTESIAN_POINT ( 'NONE',  ( 144.3824251345948255, 5.500000000000012434, 2.278174593052012309 ) ) ;
#28703=ORIENTED_EDGE ( 'NONE', *, *, #2366, .F. ) ;
#28705=CARTESIAN_POINT ( 'NONE',  ( -15.49999999999999289, -25.00000000000007816, 7.500000000000007105 ) ) ;
#28708=CARTESIAN_POINT ( 'NONE',  ( 138.2663997308104342, -4.999999999999989342, -2.071067811865468400 ) ) ;
#28715=EDGE_CURVE ( 'NONE', #15499, #22218, #21085, .T. ) ;
#28725=CARTESIAN_POINT ( 'NONE',  ( 135.6562500000000284, -6.000000000000005329, 2.485281374238556218 ) ) ;
#28728=MECHANICAL_DESIGN_GEOMETRIC_PRESENTATION_REPRESENTATION('',(#8651),#868);
#28732=AXIS2_PLACEMENT_3D ( 'NONE', #18499, #27821, #25 ) ;
#28746=MECHANICAL_DESIGN_GEOMETRIC_PRESENTATION_REPRESENTATION('',(#24836),#2299);
#28748=SURFACE_SIDE_STYLE ('',( #21721 ) ) ;
#28752=CARTESIAN_POINT ( 'NONE',  ( 139.7122326009735218, -8.976976166826791115, 7.966489656652901985 ) ) ;
#28758=FILL_AREA_STYLE ('',( #21732 ) ) ;
#28759=CARTESIAN_POINT ( 'NONE',  ( 145.8898502691896510, 3.535533905932725318, -3.535533905932725318 ) ) ;
#28760=CARTESIAN_POINT ( 'NONE',  ( 149.6250000000000284, 0.000000000000000000, -6.000000000000005329 ) ) ;
#28764=DIRECTION ( 'NONE',  ( 1.000000000000000000, 0.000000000000000000, 0.000000000000000000 ) ) ;
#28766=CARTESIAN_POINT ( 'NONE',  ( 144.3750000000000284, 0.000000000000000000, 6.000000000000005329 ) ) ;
#28768=DIRECTION ( 'NONE',  ( 0.000000000000000000, -0.7999999999999996003, -0.6000000000000006439 ) ) ;
#28771=VERTEX_POINT ( 'NONE', #20629 ) ;
#28776=DIRECTION ( 'NONE',  ( 1.000000000000000000, -0.000000000000000000, -0.000000000000000000 ) ) ;
#28782=EDGE_CURVE ( 'NONE', #19300, #605, #27658, .T. ) ;
#28784=EDGE_CURVE ( 'NONE', #22616, #11342, #2481, .T. ) ;
#28792=CARTESIAN_POINT ( 'NONE',  ( 145.2261751345948539, -3.889087296526011706, -3.889087296526011706 ) ) ;
#28798=CARTESIAN_POINT ( 'NONE',  ( -4.999999999999984013, -10.50000000000000888, -8.000000000000007105 ) ) ;
#28805=ORIENTED_EDGE ( 'NONE', *, *, #28305, .F. ) ;
#28806=( GEOMETRIC_REPRESENTATION_CONTEXT ( 3 ) GLOBAL_UNCERTAINTY_ASSIGNED_CONTEXT ( ( #16853 ) ) GLOBAL_UNIT_ASSIGNED_CONTEXT ( ( #16924, #7513, #28545 ) ) REPRESENTATION_CONTEXT ( 'NONE', 'WORKASPACE' ) );
#28807=ORIENTED_EDGE ( 'NONE', *, *, #4729, .F. ) ;
#28808=ORIENTED_EDGE ( 'NONE', *, *, #493, .T. ) ;
#28813=ORIENTED_EDGE ( 'NONE', *, *, #5344, .F. ) ;
#28816=CARTESIAN_POINT ( 'NONE',  ( 135.0000000000000284, -7.146604258052373204, 8.399325966929822584 ) ) ;
#28818=CARTESIAN_POINT ( 'NONE',  ( 131.8913997308104058, -2.071067811865468400, 4.999999999999989342 ) ) ;
#28832=( BOUNDED_SURFACE ( )  B_SPLINE_SURFACE ( 3, 2, ( 
 ( #12165, #21354, #438 ),
 ( #6757, #16178, #16328 ),
 ( #150, #20907, #25482 ),
 ( #11563, #14323, #4449 ),
 ( #13874, #16473, #18918 ),
 ( #4751, #21056, #14178 ),
 ( #23215, #30251, #9220 ),
 ( #30404, #4892, #9373 ),
 ( #25945, #18764, #23515 ),
 ( #2456, #11872, #28239 ) ),
 .UNSPECIFIED., .F., .F., .T. ) 
 B_SPLINE_SURFACE_WITH_KNOTS ( ( 4, 2, 2, 2, 4 ),
 ( 3, 3 ),
 ( 0.0004283140159002545347, 0.001007014806553221432, 0.001585715597206188276, 0.002164416387859155119, 0.002743117178512121963 ),
 ( 0.000000000000000000, 1.000000000000000000 ),
 .UNSPECIFIED. ) 
 GEOMETRIC_REPRESENTATION_ITEM ( )  RATIONAL_B_SPLINE_SURFACE ( (
 ( 1.000000000000000000, 0.7071067811872737696, 1.000000000000000000),
 ( 1.000000000000000000, 0.7334468984528983437, 1.000000000000000000),
 ( 1.000000000000000000, 0.7709563466230319184, 1.000000000000000000),
 ( 1.000000000000000000, 0.8514970365135478003, 1.000000000000000000),
 ( 1.000000000000000000, 0.8914860584493291551, 1.000000000000000000),
 ( 1.000000000000000000, 0.9504033078762521569, 1.000000000000000000),
 ( 1.000000000000000000, 0.9703159229117922502, 1.000000000000000000),
 ( 1.000000000000000000, 0.9949510651229506175, 1.000000000000000000),
 ( 1.000000000000000000, 0.9999594700102402145, 1.000000000000000000),
 ( 1.000000000000000000, 1.000000000000000000, 1.000000000000000000) ) ) 
 REPRESENTATION_ITEM ( '' )  SURFACE ( )  );
#28834=( NAMED_UNIT ( * ) SI_UNIT ( $, .STERADIAN. ) SOLID_ANGLE_UNIT ( ) );
#28846=SURFACE_STYLE_FILL_AREA ( #894 ) ;
#28850=VERTEX_POINT ( 'NONE', #26270 ) ;
#28853=CARTESIAN_POINT ( 'NONE',  ( 133.9836002691896510, 4.999999999999989342, -2.071067811865468400 ) ) ;
#28860=ORIENTED_EDGE ( 'NONE', *, *, #1575, .T. ) ;
#28864=CARTESIAN_POINT ( 'NONE',  ( 140.8913997308104626, -2.071067811865468400, 4.999999999999989342 ) ) ;
#28876=DIRECTION ( 'NONE',  ( 0.000000000000000000, 0.000000000000000000, 1.000000000000000000 ) ) ;
#28877=EDGE_LOOP ( 'NONE', ( #13650, #23222, #11927, #24790 ) ) ;
#28883=CARTESIAN_POINT ( 'NONE',  ( 155.8199251345948255, -2.278174593051950136, -5.500000000000074607 ) ) ;
#28887=ADVANCED_FACE ( 'NONE', ( #23979 ), #29502, .T. ) ;
#28900=CARTESIAN_POINT ( 'NONE',  ( 116.0000000000000142, 0.000000000000000000, 0.000000000000000000 ) ) ;
#28902=CARTESIAN_POINT ( 'NONE',  ( -10.00000000000000178, -19.99999999999998934, 3.000000000000002665 ) ) ;
#28910=CARTESIAN_POINT ( 'NONE',  ( 138.1086002691896510, -2.071067811865468400, -4.999999999999989342 ) ) ;
#28911=CARTESIAN_POINT ( 'NONE',  ( 149.2500000000000284, -6.000000000000005329, 0.000000000000000000 ) ) ;
#28917=COLOUR_RGB ( '', 0.66274510, 0.83137255, 0.94901961) ;
#28918=CARTESIAN_POINT ( 'NONE',  ( 146.5312500000000284, -2.485281374238555774, -6.000000000000005329 ) ) ;
#28920=AXIS2_PLACEMENT_3D ( 'NONE', #6148, #15563, #29486 ) ;
#28922=( BOUNDED_CURVE ( )  B_SPLINE_CURVE ( 2, ( #28342, #10085, #11978, #14849, #12560, #23905, #17013, #10240, #543 ),
 .UNSPECIFIED., .F., .T. ) 
 B_SPLINE_CURVE_WITH_KNOTS ( ( 3, 2, 2, 2, 3 ),
 ( 0.5875000000000001332, 0.5937500000000003331, 0.6000000000000005329, 0.6062500000000007327, 0.6125000000000010436 ),
 .UNSPECIFIED. ) 
 CURVE ( )  GEOMETRIC_REPRESENTATION_ITEM ( )  RATIONAL_B_SPLINE_CURVE ( ( 0.9999999999999986677, 0.9238795325112880708, 1.000000000000000000, 0.9238795325112867385, 1.000000000000000000, 0.9238795325112867385, 1.000000000000000000, 0.9238795325112745260, 1.000000000000012212 ) ) 
 REPRESENTATION_ITEM ( '' )  );
#28923=EDGE_CURVE ( 'NONE', #11992, #25088, #13886, .T. ) ;
#28927=ORIENTED_EDGE ( 'NONE', *, *, #26499, .T. ) ;
#28932=CARTESIAN_POINT ( 'NONE',  ( 162.0000000000000284, 0.000000000000000000, 0.000000000000000000 ) ) ;
#28934=SURFACE_STYLE_USAGE ( .BOTH. , #387 ) ;
#28941=DIRECTION ( 'NONE',  ( 0.000000000000000000, -1.000000000000000000, 0.000000000000000000 ) ) ;
#28942=CARTESIAN_POINT ( 'NONE',  ( 148.6800748654052029, -2.278174593052027408, 5.499999999999996447 ) ) ;
#28953=CARTESIAN_POINT ( 'NONE',  ( 159.8437500000000000, -6.000000000000005329, -2.485281374238555774 ) ) ;
#28957=ORIENTED_EDGE ( 'NONE', *, *, #29666, .T. ) ;
#28959=AXIS2_PLACEMENT_3D ( 'NONE', #7906, #1296, #20054 ) ;
#28961=CARTESIAN_POINT ( 'NONE',  ( 146.5312500000000284, -2.485281374238555774, -6.000000000000005329 ) ) ;
#28979=CARTESIAN_POINT ( 'NONE',  ( -0.5130136762305975706, -9.973972647538824177, 4.738252045315890726 ) ) ;
#28980=LINE ( 'NONE', #1031, #11399 ) ;
#28981=AXIS2_PLACEMENT_3D ( 'NONE', #1412, #8638, #8481 ) ;
#28983=SURFACE_SIDE_STYLE ('',( #17058 ) ) ;
#28995=EDGE_LOOP ( 'NONE', ( #10112, #4506, #22915, #24868, #3727, #17837, #12211, #18425, #27722, #14515, #28957, #12954, #21021, #26585, #24581, #24314, #4685, #17197, #11107, #16887, #13540, #11607, #16809, #15850, #12619, #21151, #21488, #15573, #22067, #25808, #28087, #16475, #26406, #18049, #3781, #21966, #27683, #6544, #3352 ) ) ;
#28996=EDGE_CURVE ( 'NONE', #20381, #13576, #26417, .T. ) ;
#28998=ORIENTED_EDGE ( 'NONE', *, *, #9883, .F. ) ;
#28999=CARTESIAN_POINT ( 'NONE',  ( 132.8586002691896510, 2.071067811865468400, 4.999999999999989342 ) ) ;
#29002=DIRECTION ( 'NONE',  ( 1.000000000000000000, 0.000000000000000000, 0.000000000000000000 ) ) ;
#29007=ORIENTED_EDGE ( 'NONE', *, *, #14398, .T. ) ;
#29012=CARTESIAN_POINT ( 'NONE',  ( 138.0788997308104342, -4.999999999999989342, 2.071067811865468400 ) ) ;
#29016=CIRCLE ( 'NONE', #15844, 15.99999999999998579 ) ;
#29019=DIRECTION ( 'NONE',  ( -1.000000000000000000, -3.469446951953614189E-15, 0.000000000000000000 ) ) ;
#29023=ORIENTED_EDGE ( 'NONE', *, *, #25051, .T. ) ;
#29026=DIRECTION ( 'NONE',  ( -0.000000000000000000, 1.000000000000000000, -0.000000000000000000 ) ) ;
#29027=PLANE ( 'NONE',  #29613 ) ;
#29028=DIRECTION ( 'NONE',  ( -1.000000000000000000, 0.000000000000000000, 0.000000000000000000 ) ) ;
#29029=EDGE_CURVE ( 'NONE', #10410, #22270, #2268, .T. ) ;
#29031=VERTEX_POINT ( 'NONE', #22130 ) ;
#29034=CARTESIAN_POINT ( 'NONE',  ( 135.3750000000000284, 0.000000000000000000, 6.000000000000005329 ) ) ;
#29045=CARTESIAN_POINT ( 'NONE',  ( 158.9136751345948539, 0.000000000000000000, -5.500000000000005329 ) ) ;
#29047=( NAMED_UNIT ( * ) SI_UNIT ( $, .STERADIAN. ) SOLID_ANGLE_UNIT ( ) );
#29050=CARTESIAN_POINT ( 'NONE',  ( 155.9851497308104058, -3.535533905932725318, 3.535533905932725318 ) ) ;
#29051=DIRECTION ( 'NONE',  ( -1.000000000000000000, 0.000000000000000000, 0.000000000000000000 ) ) ;
#29053=FILL_AREA_STYLE_COLOUR ( '', #19210 ) ;
#29054=AXIS2_PLACEMENT_3D ( 'NONE', #6856, #6390, #9020 ) ;
#29058=CARTESIAN_POINT ( 'NONE',  ( 146.9925748654052313, 2.278174593052027408, 5.499999999999996447 ) ) ;
#29062=CARTESIAN_POINT ( 'NONE',  ( 116.0000000000000142, 0.000000000000000000, 0.000000000000000000 ) ) ;
#29063=ORIENTED_EDGE ( 'NONE', *, *, #14744, .T. ) ;
#29064=CARTESIAN_POINT ( 'NONE',  ( 155.0625000000000284, -4.242640687119298093, 4.242640687119298093 ) ) ;
#29065=CARTESIAN_POINT ( 'NONE',  ( 135.5000000000000000, -54.99999999999993605, 7.500000000000007105 ) ) ;
#29068=MECHANICAL_DESIGN_GEOMETRIC_PRESENTATION_REPRESENTATION('',(#4555),#19765);
#29070=CARTESIAN_POINT ( 'NONE',  ( 145.0312500000000568, -2.485281374238555774, -6.000000000000005329 ) ) ;
#29081=EDGE_CURVE ( 'NONE', #1732, #21964, #17278, .T. ) ;
#29083=CARTESIAN_POINT ( 'NONE',  ( 140.0000000000000284, -11.48545691804907420, -4.867024281885878878 ) ) ;
#29084=CARTESIAN_POINT ( 'NONE',  ( 134.5875105163469811, -7.951309655804374543, 8.000000000000007105 ) ) ;
#29090=DIRECTION ( 'NONE',  ( -1.000000000000000000, 0.000000000000000000, 0.000000000000000000 ) ) ;
#29092=ADVANCED_FACE ( 'NONE', ( #13251 ), #10934, .T. ) ;
#29093=CARTESIAN_POINT ( 'NONE',  ( 154.0461002691896795, -2.071067811865468400, 4.999999999999989342 ) ) ;
#29095=CARTESIAN_POINT ( 'NONE',  ( 139.9669392956159300, -9.668196137844805804, -7.713418679898259356 ) ) ;
#29112=ORIENTED_EDGE ( 'NONE', *, *, #17222, .F. ) ;
#29120=LINE ( 'NONE', #5773, #17188 ) ;
#29122=CARTESIAN_POINT ( 'NONE',  ( -19.99999999999998224, -54.99999999999990763, 7.500000000000007105 ) ) ;
#29126=CARTESIAN_POINT ( 'NONE',  ( 152.5238248654052313, 3.889087296526011706, -3.889087296526011706 ) ) ;
#29131=( LENGTH_UNIT ( ) NAMED_UNIT ( * ) SI_UNIT ( .MILLI., .METRE. ) );
#29134=CARTESIAN_POINT ( 'NONE',  ( 135.0000000000000284, -8.936766734253373201, 7.963374800949050147 ) ) ;
#29138=LINE ( 'NONE', #7955, #11560 ) ;
#29142=CARTESIAN_POINT ( 'NONE',  ( 138.8363248654052029, 0.000000000000000000, -5.500000000000005329 ) ) ;
#29144=DIRECTION ( 'NONE',  ( -1.000000000000000000, -0.000000000000000000, -0.000000000000000000 ) ) ;
#29148=CARTESIAN_POINT ( 'NONE',  ( 160.9687500000000000, -2.485281374238585972, 6.000000000000005329 ) ) ;
#29152=DIRECTION ( 'NONE',  ( 1.734723475976824844E-16, -1.000000000000000000, 0.000000000000000000 ) ) ;
#29153=LINE ( 'NONE', #5975, #10854 ) ;
#29161=CARTESIAN_POINT ( 'NONE',  ( 0.9999999929836370649, -15.13506141816058914, -8.789165735397107326 ) ) ;
#29163=FILL_AREA_STYLE_COLOUR ( '', #23404 ) ;
#29167=EDGE_CURVE ( 'NONE', #30104, #30382, #12944, .T. ) ;
#29174=CARTESIAN_POINT ( 'NONE',  ( 139.5000000000000284, -9.165151389911669000, -8.500000000000007105 ) ) ;
#29176=CARTESIAN_POINT ( 'NONE',  ( 141.0000000000000284, -19.99999999999998934, 5.000000000000004441 ) ) ;
#29181=CYLINDRICAL_SURFACE ( 'NONE', #746, 5.500000000000000000 ) ;
#29183=CARTESIAN_POINT ( 'NONE',  ( 155.9136751345948539, 0.000000000000000000, -5.500000000000005329 ) ) ;
#29185=CARTESIAN_POINT ( 'NONE',  ( 140.9019117484303933, -11.80382349685853427, 4.000000000000003553 ) ) ;
#29191=ADVANCED_FACE ( 'NONE', ( #20742 ), #4490, .T. ) ;
#29192=CARTESIAN_POINT ( 'NONE',  ( 140.8199251345947687, -2.278174593052058938, -5.499999999999964473 ) ) ;
#29196=CARTESIAN_POINT ( 'NONE',  ( 149.2351497308104342, 3.535533905932725318, -3.535533905932725318 ) ) ;
#29197=CARTESIAN_POINT ( 'NONE',  ( 154.4136751345948539, 0.000000000000000000, -5.500000000000005329 ) ) ;
#29201=ADVANCED_FACE ( 'NONE', ( #27615 ), #142, .T. ) ;
#29203=TOROIDAL_SURFACE ( 'NONE', #11102, 1.000000000000000000, 0.5000000000000000000 ) ;
#29205=AXIS2_PLACEMENT_3D ( 'NONE', #2260, #18557, #8868 ) ;
#29207=DIRECTION ( 'NONE',  ( 1.000000000000000000, 0.000000000000000000, 0.000000000000000000 ) ) ;
#29209=ORIENTED_EDGE ( 'NONE', *, *, #18783, .T. ) ;
#29210=CARTESIAN_POINT ( 'NONE',  ( 145.8750000000000284, 0.000000000000000000, 6.000000000000005329 ) ) ;
#29211=CARTESIAN_POINT ( 'NONE',  ( 159.0000000000000284, -19.99999999999998934, 3.000000000000002665 ) ) ;
#29217=CARTESIAN_POINT ( 'NONE',  ( 144.0937500000000000, 6.000000000000005329, 2.485281374238585972 ) ) ;
#29218=CARTESIAN_POINT ( 'NONE',  ( 161.1201765630156615, -0.6312603797374088943, 5.593606079993166169 ) ) ;
#29219=B_SPLINE_CURVE_WITH_KNOTS ( 'NONE', 3,
 ( #23739, #21435, #10215, #17137, #16990, #26314, #367, #9756, #5270, #2967 ),
 .UNSPECIFIED., .F., .F.,
 ( 4, 2, 2, 2, 4 ),
 ( -1.043662239764700441E-05, 0.0005703011627235046472, 0.001151038947844656339, 0.001731776732965803478, 0.002312514518086950834 ),
 .UNSPECIFIED. ) ;
#29226=ADVANCED_FACE ( 'NONE', ( #6591 ), #30092, .F. ) ;
#29231=CARTESIAN_POINT ( 'NONE',  ( 147.9300748654052313, 2.278174593051764951, -5.500000000000262013 ) ) ;
#29243=CARTESIAN_POINT ( 'NONE',  ( 151.1398502691896510, -3.535533905932752852, 3.535533905932725318 ) ) ;
#29254=DIRECTION ( 'NONE',  ( 1.000000000000000000, 0.000000000000000000, -0.000000000000000000 ) ) ;
#29260=ORIENTED_EDGE ( 'NONE', *, *, #2719, .T. ) ;
#29261=CIRCLE ( 'NONE', #11156, 14.99999999999998579 ) ;
#29265=ADVANCED_FACE ( 'NONE', ( #13707 ), #20203, .T. ) ;
#29270=CARTESIAN_POINT ( 'NONE',  ( 0.000000000000000000, 10.00000000000000888, -5.000000000000004441 ) ) ;
#29276=CARTESIAN_POINT ( 'NONE',  ( 155.7113248654052313, 5.500000000000005329, 0.000000000000000000 ) ) ;
#29279=CARTESIAN_POINT ( 'NONE',  ( -0.08386379889025598333, -15.14278526281355219, 7.883982414521697457 ) ) ;
#29281=CARTESIAN_POINT ( 'NONE',  ( -0.9345383689551277628, -9.130923262089552850, 4.000000000000004441 ) ) ;
#29289=CARTESIAN_POINT ( 'NONE',  ( 135.0000000000000284, -8.656969940506323624, 7.548343266826465836 ) ) ;
#29292=CARTESIAN_POINT ( 'NONE',  ( 159.0000000000000284, -59.99999999999980105, -3.000000000000002665 ) ) ;
#29293=CARTESIAN_POINT ( 'NONE',  ( 161.4375000000000284, -4.242640687119298093, -4.242640687119298093 ) ) ;
#29294=MECHANICAL_DESIGN_GEOMETRIC_PRESENTATION_REPRESENTATION('',(#21485),#7265);
#29298=CARTESIAN_POINT ( 'NONE',  ( 149.9136751345948539, 0.000000000000000000, -5.500000000000005329 ) ) ;
#29302=LINE ( 'NONE', #10915, #17085 ) ;
#29303=ORIENTED_EDGE ( 'NONE', *, *, #6855, .F. ) ;
#29308=CARTESIAN_POINT ( 'NONE',  ( 156.4687500000000284, -2.485281374238585972, 6.000000000000005329 ) ) ;
#29316=CARTESIAN_POINT ( 'NONE',  ( 8.673617379884035472E-16, -15.46117127753089449, -5.976030864474088489 ) ) ;
#29321=CARTESIAN_POINT ( 'NONE',  ( 8.673617379884035472E-16, -14.27031434886951544, -8.428912904374499249 ) ) ;
#29326=CARTESIAN_POINT ( 'NONE',  ( 135.0000000000001137, 4.403472173772889242, 3.650336322691055013 ) ) ;
#29327=CARTESIAN_POINT ( 'NONE',  ( 148.0386751345948539, -5.500000000000005329, 0.000000000000000000 ) ) ;
#29336=CARTESIAN_POINT ( 'NONE',  ( 124.9999999999999432, -71.00000000000001421, 4.000000000000003553 ) ) ;
#29337=ORIENTED_EDGE ( 'NONE', *, *, #23927, .F. ) ;
#29339=PRESENTATION_STYLE_ASSIGNMENT (( #15728 ) ) ;
#29340=ADVANCED_FACE ( 'NONE', ( #11553 ), #21195, .T. ) ;
#29343=CARTESIAN_POINT ( 'NONE',  ( 155.7261751345948539, -3.889087296526011706, -3.889087296526011706 ) ) ;
#29345=CARTESIAN_POINT ( 'NONE',  ( 140.8038234968598488, -11.90191174842882660, 4.000000000000003553 ) ) ;
#29346=CARTESIAN_POINT ( 'NONE',  ( 144.4687500000000568, -2.485281374238585972, 6.000000000000005329 ) ) ;
#29347=EDGE_CURVE ( 'NONE', #8327, #17555, #26554, .T. ) ;
#29349=CARTESIAN_POINT ( 'NONE',  ( 159.9871598483856587, -11.17259796798583515, 4.379265499705882192 ) ) ;
#29351=CARTESIAN_POINT ( 'NONE',  ( 140.4449251345948539, -5.500000000000012434, 2.278174593052012309 ) ) ;
#29355=CARTESIAN_POINT ( 'NONE',  ( 136.0000000000000284, -8.798545334315230448, -8.160000000000007248 ) ) ;
#29356=CARTESIAN_POINT ( 'NONE',  ( 151.2038997308104058, 2.071067811865468400, 4.999999999999989342 ) ) ;
#29359=( NAMED_UNIT ( * ) PLANE_ANGLE_UNIT ( ) SI_UNIT ( $, .RADIAN. ) );
#29363=CARTESIAN_POINT ( 'NONE',  ( -1.000000000000000888, -10.00000000000000888, -4.000000000000003553 ) ) ;
#29364=EDGE_LOOP ( 'NONE', ( #13393, #26181, #13079, #3312, #9955 ) ) ;
#29370=CARTESIAN_POINT ( 'NONE',  ( 143.9062500000000284, 6.000000000000005329, -2.485281374238556218 ) ) ;
#29378=EDGE_LOOP ( 'NONE', ( #27597, #14366, #14728, #14259 ) ) ;
#29379=ADVANCED_FACE ( 'NONE', ( #17049 ), #28376, .F. ) ;
#29381=( GEOMETRIC_REPRESENTATION_CONTEXT ( 3 ) GLOBAL_UNCERTAINTY_ASSIGNED_CONTEXT ( ( #6065 ) ) GLOBAL_UNIT_ASSIGNED_CONTEXT ( ( #12500, #11090, #20755 ) ) REPRESENTATION_CONTEXT ( 'NONE', 'WORKASPACE' ) );
#29384=ORIENTED_EDGE ( 'NONE', *, *, #6922, .F. ) ;
#29398=TOROIDAL_SURFACE ( 'NONE', #960, 12.50000000000000178, 0.5000000000000000000 ) ;
#29402=CIRCLE ( 'NONE', #7808, 0.5000000000000004441 ) ;
#29403=DIRECTION ( 'NONE',  ( 0.000000000000000000, 0.000000000000000000, -1.000000000000000000 ) ) ;
#29404=CARTESIAN_POINT ( 'NONE',  ( 161.3006082692931500, -4.487120878302232718, -3.700106666589778825 ) ) ;
#29410=ADVANCED_FACE ( 'NONE', ( #12156 ), #428, .T. ) ;
#29411=ORIENTED_EDGE ( 'NONE', *, *, #22351, .T. ) ;
#29414=CARTESIAN_POINT ( 'NONE',  ( 145.5074251345947971, 2.278174593051996322, -5.500000000000026645 ) ) ;
#29418=ORIENTED_EDGE ( 'NONE', *, *, #22757, .T. ) ;
#29422=VERTEX_POINT ( 'NONE', #16904 ) ;
#29424=VECTOR ( 'NONE', #7596, 1000.000000000000000 ) ;
#29425=CARTESIAN_POINT ( 'NONE',  ( 135.0000000000000284, -9.047800747817552391, 7.500000000000007105 ) ) ;
#29429=CARTESIAN_POINT ( 'NONE',  ( 135.5000000000000000, -24.99999999999999289, -8.000000000000007105 ) ) ;
#29441=CARTESIAN_POINT ( 'NONE',  ( 140.9136751345948539, 0.000000000000000000, -5.500000000000005329 ) ) ;
#29453=CARTESIAN_POINT ( 'NONE',  ( 149.8050748654052313, 5.500000000000012434, 2.278174593052012309 ) ) ;
#29454=ORIENTED_EDGE ( 'NONE', *, *, #6227, .T. ) ;
#29457=EDGE_LOOP ( 'NONE', ( #1898, #25699, #9426, #15226 ) ) ;
#29459=CARTESIAN_POINT ( 'NONE',  ( 159.2812500000000568, 2.485281374238585972, 6.000000000000005329 ) ) ;
#29464=CARTESIAN_POINT ( 'NONE',  ( 150.8511751345948255, -3.889087296526011706, 3.889087296526011706 ) ) ;
#29467=CARTESIAN_POINT ( 'NONE',  ( 153.6636751345948255, 0.000000000000000000, 5.500000000000005329 ) ) ;
#29474=( BOUNDED_CURVE ( )  B_SPLINE_CURVE ( 2, ( #26942, #15329, #12276, #552, #12721, #26489, #22060, #21619, #9942 ),
 .UNSPECIFIED., .F., .T. ) 
 B_SPLINE_CURVE_WITH_KNOTS ( ( 3, 2, 2, 2, 3 ),
 ( 0.8625000000000012657, 0.8687500000000010214, 0.8750000000000008882, 0.8812500000000006439, 0.8875000000000003997 ),
 .UNSPECIFIED. ) 
 CURVE ( )  GEOMETRIC_REPRESENTATION_ITEM ( )  RATIONAL_B_SPLINE_CURVE ( ( 0.9999999999999851230, 0.9238795325113016155, 1.000000000000000000, 0.9238795325112867385, 1.000000000000000000, 0.9238795325112867385, 1.000000000000000000, 0.9238795325112812984, 1.000000000000005329 ) ) 
 REPRESENTATION_ITEM ( '' )  );
#29475=CARTESIAN_POINT ( 'NONE',  ( 159.7582345317023567, -12.26499483057044415, -3.655200626169436084 ) ) ;
#29485=DIRECTION ( 'NONE',  ( 1.000000000000000000, 0.000000000000000000, -0.000000000000000000 ) ) ;
#29486=DIRECTION ( 'NONE',  ( 1.000000000000000000, 0.000000000000000000, 0.000000000000000000 ) ) ;
#29488=VECTOR ( 'NONE', #27251, 1000.000000000000000 ) ;
#29495=CARTESIAN_POINT ( 'NONE',  ( 139.7023502691896510, 0.000000000000000000, -5.000000000000004441 ) ) ;
#29496=ADVANCED_FACE ( 'NONE', ( #26524 ), #3175, .F. ) ;
#29500=LINE ( 'NONE', #23339, #9225 ) ;
#29502=TOROIDAL_SURFACE ( 'NONE', #9414, 14.49999999999999822, 0.5000000000000000000 ) ;
#29503=CARTESIAN_POINT ( 'NONE',  ( 140.0707155294794006, -11.09459640813432557, -4.575173035329879845 ) ) ;
#29505=AXIS2_PLACEMENT_3D ( 'NONE', #5951, #24097, #12917 ) ;
#29509=CARTESIAN_POINT ( 'NONE',  ( 144.7500000000000568, -6.000000000000005329, 0.000000000000000000 ) ) ;
#29512=DIRECTION ( 'NONE',  ( 1.000000000000000000, 0.000000000000000000, 0.000000000000000000 ) ) ;
#29514=DIRECTION ( 'NONE',  ( -0.000000000000000000, -0.000000000000000000, -1.000000000000000000 ) ) ;
#29515=CARTESIAN_POINT ( 'NONE',  ( 136.4136751345948539, 0.000000000000000000, -5.500000000000005329 ) ) ;
#29518=CARTESIAN_POINT ( 'NONE',  ( 147.8288997308104342, 4.999999999999989342, -2.071067811865468400 ) ) ;
#29519=VECTOR ( 'NONE', #22670, 1000.000000000000000 ) ;
#29521=CYLINDRICAL_SURFACE ( 'NONE', #23123, 1.000000000000000000 ) ;
#29523=EDGE_CURVE ( 'NONE', #17248, #7661, #23273, .T. ) ;
#29524=FACE_OUTER_BOUND ( 'NONE', #9120, .T. ) ;
#29525=SURFACE_SIDE_STYLE ('',( #12984 ) ) ;
#29532=ORIENTED_EDGE ( 'NONE', *, *, #1059, .T. ) ;
#29535=EDGE_CURVE ( 'NONE', #14644, #12881, #24135, .T. ) ;
#29536=DIRECTION ( 'NONE',  ( -0.000000000000000000, -0.000000000000000000, -1.000000000000000000 ) ) ;
#29537=ORIENTED_EDGE ( 'NONE', *, *, #13407, .F. ) ;
#29539=CARTESIAN_POINT ( 'NONE',  ( 145.7812500000000284, 2.485281374238585972, 6.000000000000005329 ) ) ;
#29540=CARTESIAN_POINT ( 'NONE',  ( 141.6636751345948255, 0.000000000000000000, 5.500000000000005329 ) ) ;
#29544=CARTESIAN_POINT ( 'NONE',  ( 138.4687500000000284, -2.485281374238585972, 6.000000000000005329 ) ) ;
#29545=CARTESIAN_POINT ( 'NONE',  ( 161.2143795948215370, -3.807535749796857605, 4.272797826763722995 ) ) ;
#29555=ORIENTED_EDGE ( 'NONE', *, *, #17909, .F. ) ;
#29572=CARTESIAN_POINT ( 'NONE',  ( 153.8586002691896510, 2.071067811865468400, 4.999999999999989342 ) ) ;
#29574=CARTESIAN_POINT ( 'NONE',  ( 135.4761751345948539, 3.889087296526011706, 3.889087296526011706 ) ) ;
#29576=CARTESIAN_POINT ( 'NONE',  ( 150.3675748654052313, -5.500000000000012434, 2.278174593052012309 ) ) ;
#29579=CARTESIAN_POINT ( 'NONE',  ( 157.7812500000000568, 2.485281374238585972, 6.000000000000005329 ) ) ;
#29589=ORIENTED_EDGE ( 'NONE', *, *, #14910, .F. ) ;
#29591=FILL_AREA_STYLE_COLOUR ( '', #15767 ) ;
#29592=CARTESIAN_POINT ( 'NONE',  ( 0.7509638210179210294, -15.55246597669451170, 8.023235780102909942 ) ) ;
#29593=EDGE_CURVE ( 'NONE', #29422, #765, #23152, .T. ) ;
#29595=VERTEX_POINT ( 'NONE', #20088 ) ;
#29596=DIRECTION ( 'NONE',  ( 1.000000000000000000, 0.000000000000000000, 0.000000000000000000 ) ) ;
#29604=SURFACE_SIDE_STYLE ('',( #22560 ) ) ;
#29612=FILL_AREA_STYLE ('',( #6727 ) ) ;
#29613=AXIS2_PLACEMENT_3D ( 'NONE', #7993, #1224, #10321 ) ;
#29618=CARTESIAN_POINT ( 'NONE',  ( 153.8437500000000284, -6.000000000000005329, -2.485281374238555774 ) ) ;
#29621=ORIENTED_EDGE ( 'NONE', *, *, #1092, .F. ) ;
#29622=CARTESIAN_POINT ( 'NONE',  ( 151.2261751345948539, -3.889087296526011706, -3.889087296526011706 ) ) ;
#29626=SURFACE_SIDE_STYLE ('',( #6742 ) ) ;
#29627=ADVANCED_FACE ( 'NONE', ( #15511 ), #27130, .T. ) ;
#29628=ORIENTED_EDGE ( 'NONE', *, *, #27125, .F. ) ;
#29638=DIRECTION ( 'NONE',  ( 0.000000000000000000, -0.9393939393939397808, 0.3428396514843859988 ) ) ;
#29639=CARTESIAN_POINT ( 'NONE',  ( -38.99999999999998579, -59.99999999999980105, -4.000000000000003553 ) ) ;
#29644=CARTESIAN_POINT ( 'NONE',  ( 160.3050748654052029, 5.500000000000012434, 2.278174593052012309 ) ) ;
#29646=CARTESIAN_POINT ( 'NONE',  ( 142.2336002691896226, -4.999999999999989342, 2.071067811865468400 ) ) ;
#29651=CARTESIAN_POINT ( 'NONE',  ( 140.0256844536733922, -11.04862469602451291, -4.684420475249996052 ) ) ;
#29654=ORIENTED_EDGE ( 'NONE', *, *, #4037, .T. ) ;
#29655=CARTESIAN_POINT ( 'NONE',  ( 159.6405936598872586, -12.17689969114422688, 3.778228146401014342 ) ) ;
#29656=CARTESIAN_POINT ( 'NONE',  ( 139.7812500000000284, 2.485281374238585972, 6.000000000000005329 ) ) ;
#29657=( BOUNDED_CURVE ( )  B_SPLINE_CURVE ( 2, ( #4939, #23265, #9730, #14370, #19107, #28432, #16671, #9575, #23708 ),
 .UNSPECIFIED., .F., .T. ) 
 B_SPLINE_CURVE_WITH_KNOTS ( ( 3, 2, 2, 2, 3 ),
 ( 0.7625000000000011768, 0.7687500000000010436, 0.7750000000000007994, 0.7812500000000004441, 0.7875000000000001998 ),
 .UNSPECIFIED. ) 
 CURVE ( )  GEOMETRIC_REPRESENTATION_ITEM ( )  RATIONAL_B_SPLINE_CURVE ( ( 0.9999999999999851230, 0.9238795325113016155, 1.000000000000000000, 0.9238795325112867385, 1.000000000000000000, 0.9238795325112867385, 1.000000000000000000, 0.9238795325112840739, 1.000000000000002665 ) ) 
 REPRESENTATION_ITEM ( '' )  );
#29660=SURFACE_STYLE_USAGE ( .BOTH. , #20312 ) ;
#29666=EDGE_CURVE ( 'NONE', #19330, #3655, #450, .T. ) ;
#29667=FACE_OUTER_BOUND ( 'NONE', #16782, .T. ) ;
#29668=CARTESIAN_POINT ( 'NONE',  ( 149.1413997308104058, 2.071067811865468400, -4.999999999999989342 ) ) ;
#29671=CIRCLE ( 'NONE', #16970, 1.000000000000000222 ) ;
#29676=EDGE_LOOP ( 'NONE', ( #14121, #762, #7354, #2167, #15809 ) ) ;
#29681=ORIENTED_EDGE ( 'NONE', *, *, #26599, .F. ) ;
#29683=CARTESIAN_POINT ( 'NONE',  ( 145.0312500000000568, -2.485281374238556218, -6.000000000000005329 ) ) ;
#29685=CARTESIAN_POINT ( 'NONE',  ( 141.0000000000000284, -12.00000000000001066, -4.000000000000003553 ) ) ;
#29686=CARTESIAN_POINT ( 'NONE',  ( 139.7812500000000284, 2.485281374238585972, 6.000000000000005329 ) ) ;
#29689=ORIENTED_EDGE ( 'NONE', *, *, #21297, .T. ) ;
#29691=EDGE_CURVE ( 'NONE', #23494, #18429, #3026, .T. ) ;
#29693=ORIENTED_EDGE ( 'NONE', *, *, #14719, .F. ) ;
#29699=EDGE_CURVE ( 'NONE', #24857, #8961, #2976, .T. ) ;
#29701=AXIS2_PLACEMENT_3D ( 'NONE', #12448, #21791, #7355 ) ;
#29704=CARTESIAN_POINT ( 'NONE',  ( 135.3537946693345759, -8.430374945247399054, -8.227582779367073940 ) ) ;
#29710=CIRCLE ( 'NONE', #27245, 0.5000000000000004441 ) ;
#29714=CARTESIAN_POINT ( 'NONE',  ( 0.000000000000000000, 0.000000000000000000, 0.000000000000000000 ) ) ;
#29715=CARTESIAN_POINT ( 'NONE',  ( -19.99999999999998224, -25.00000000000010658, -5.000000000000004441 ) ) ;
#29717=DIRECTION ( 'NONE',  ( 1.000000000000000000, -0.000000000000000000, -0.000000000000000000 ) ) ;
#29719=ORIENTED_EDGE ( 'NONE', *, *, #9858, .T. ) ;
#29720=CARTESIAN_POINT ( 'NONE',  ( 157.0312500000000853, -2.485281374238555774, -6.000000000000005329 ) ) ;
#29722=CIRCLE ( 'NONE', #29205, 1.000000000000000444 ) ;
#29725=ORIENTED_EDGE ( 'NONE', *, *, #27299, .F. ) ;
#29727=ORIENTED_EDGE ( 'NONE', *, *, #20566, .T. ) ;
#29730=EDGE_CURVE ( 'NONE', #28093, #15499, #26034, .T. ) ;
#29732=EDGE_CURVE ( 'NONE', #6232, #8188, #19584, .T. ) ;
#29733=ORIENTED_EDGE ( 'NONE', *, *, #8956, .F. ) ;
#29734=FACE_OUTER_BOUND ( 'NONE', #5165, .T. ) ;
#29735=CARTESIAN_POINT ( 'NONE',  ( 140.3265217274359600, -9.159198771249785764, -7.753921182607669493 ) ) ;
#29736=MECHANICAL_DESIGN_GEOMETRIC_PRESENTATION_REPRESENTATION('',(#18016),#22900);
#29740=DIRECTION ( 'NONE',  ( 0.000000000000000000, 0.000000000000000000, -1.000000000000000000 ) ) ;
#29741=( BOUNDED_CURVE ( )  B_SPLINE_CURVE ( 2, ( #5112, #26160, #5411, #10208, #28460, #359, #21428, #14532, #5266 ),
 .UNSPECIFIED., .F., .T. ) 
 B_SPLINE_CURVE_WITH_KNOTS ( ( 3, 2, 2, 2, 3 ),
 ( 0.5374999999999999778, 0.5437500000000001776, 0.5500000000000004885, 0.5562500000000007994, 0.5625000000000009992 ),
 .UNSPECIFIED. ) 
 CURVE ( )  GEOMETRIC_REPRESENTATION_ITEM ( )  RATIONAL_B_SPLINE_CURVE ( ( 1.000000000000000000, 0.9238795325112867385, 1.000000000000000000, 0.9238795325112867385, 1.000000000000000000, 0.9238795325112867385, 1.000000000000000000, 0.9238795325112745260, 1.000000000000012212 ) ) 
 REPRESENTATION_ITEM ( '' )  );
#29745=FILL_AREA_STYLE ('',( #25128 ) ) ;
#29756=ORIENTED_EDGE ( 'NONE', *, *, #22820, .F. ) ;
#29761=DIRECTION ( 'NONE',  ( 1.000000000000000000, 0.000000000000000000, 0.000000000000000000 ) ) ;
#29763=AXIS2_PLACEMENT_3D ( 'NONE', #18058, #25378, #17905 ) ;
#29765=CARTESIAN_POINT ( 'NONE',  ( 125.0000000000000568, -55.00000000000000711, -7.500000000000007105 ) ) ;
#29766=( GEOMETRIC_REPRESENTATION_CONTEXT ( 3 ) GLOBAL_UNCERTAINTY_ASSIGNED_CONTEXT ( ( #7484 ) ) GLOBAL_UNIT_ASSIGNED_CONTEXT ( ( #13423, #11108, #26288 ) ) REPRESENTATION_CONTEXT ( 'NONE', 'WORKASPACE' ) );
#29767=ORIENTED_EDGE ( 'NONE', *, *, #27092, .F. ) ;
#29769=CARTESIAN_POINT ( 'NONE',  ( 156.6562500000000284, -6.000000000000005329, 2.485281374238555774 ) ) ;
#29773=ORIENTED_EDGE ( 'NONE', *, *, #4133, .T. ) ;
#29776=AXIS2_PLACEMENT_3D ( 'NONE', #22069, #22685, #24354 ) ;
#29781=CARTESIAN_POINT ( 'NONE',  ( -4.999999999999886313, -15.00000000000001421, -7.500000000000007105 ) ) ;
#29783=CARTESIAN_POINT ( 'NONE',  ( 159.4504201399719818, -12.08528864193560537, -3.895248697861249276 ) ) ;
#29791=CYLINDRICAL_SURFACE ( 'NONE', #22604, 1.000000000000000888 ) ;
#29792=CIRCLE ( 'NONE', #24364, 0.4999999999999983347 ) ;
#29799=CARTESIAN_POINT ( 'NONE',  ( 136.9836002691896510, 4.999999999999989342, -2.071067811865468400 ) ) ;
#29801=VECTOR ( 'NONE', #8919, 1000.000000000000000 ) ;
#29806=EDGE_CURVE ( 'NONE', #8961, #20296, #14067, .T. ) ;
#29811=CARTESIAN_POINT ( 'NONE',  ( 144.3750000000000284, 0.000000000000000000, 6.000000000000005329 ) ) ;
#29812=STYLED_ITEM ( 'NONE', ( #14650 ), #4906 ) ;
#29814=VERTEX_POINT ( 'NONE', #8799 ) ;
#29815=CYLINDRICAL_SURFACE ( 'NONE', #15574, 0.5000000000000000000 ) ;
#29818=CYLINDRICAL_SURFACE ( 'NONE', #10815, 0.5000000000000004441 ) ;
#29819=DIRECTION ( 'NONE',  ( 1.000000000000000000, 0.000000000000000000, 0.000000000000000000 ) ) ;
#29821=CARTESIAN_POINT ( 'NONE',  ( 152.0476497308104058, 0.000000000000000000, -5.000000000000004441 ) ) ;
#29825=DIRECTION ( 'NONE',  ( 0.000000000000000000, 0.000000000000000000, -1.000000000000000000 ) ) ;
#29826=( LENGTH_UNIT ( ) NAMED_UNIT ( * ) SI_UNIT ( .MILLI., .METRE. ) );
#29827=B_SPLINE_CURVE_WITH_KNOTS ( 'NONE', 3,
 ( #786, #23984, #26709, #2928 ),
 .UNSPECIFIED., .F., .F.,
 ( 4, 4 ),
 ( 0.000000000000000000, 0.0007769152796223661528 ),
 .UNSPECIFIED. ) ;
#29832=ORIENTED_EDGE ( 'NONE', *, *, #26134, .T. ) ;
#29839=CARTESIAN_POINT ( 'NONE',  ( 148.0312500000000284, -2.485281374238556218, -6.000000000000005329 ) ) ;
#29840=CARTESIAN_POINT ( 'NONE',  ( 160.0000000000000284, -11.67610212985246676, -2.769230769230771383 ) ) ;
#29842=EDGE_CURVE ( 'NONE', #15258, #18703, #14834, .T. ) ;
#29843=CARTESIAN_POINT ( 'NONE',  ( 139.4062500000000284, 6.000000000000005329, -2.485281374238555774 ) ) ;
#29845=ORIENTED_EDGE ( 'NONE', *, *, #15498, .F. ) ;
#29863=SURFACE_STYLE_FILL_AREA ( #18381 ) ;
#29867=CARTESIAN_POINT ( 'NONE',  ( 161.1562500000000284, -6.000000000000005329, 2.485281374238556218 ) ) ;
#29870=FACE_OUTER_BOUND ( 'NONE', #5645, .T. ) ;
#29871=AXIS2_PLACEMENT_3D ( 'NONE', #13209, #20965, #15352 ) ;
#29872=DIRECTION ( 'NONE',  ( -1.000000000000000000, 3.469446951953694061E-16, 0.000000000000000000 ) ) ;
#29874=EDGE_CURVE ( 'NONE', #22758, #1710, #13383, .T. ) ;
#29876=CARTESIAN_POINT ( 'NONE',  ( 154.4062500000000284, 6.000000000000005329, -2.485281374238555774 ) ) ;
#29878=( BOUNDED_CURVE ( )  B_SPLINE_CURVE ( 2, ( #11936, #16684, #20968, #2372, #11775, #19268, #660, #26597, #15114 ),
 .UNSPECIFIED., .F., .F. ) 
 B_SPLINE_CURVE_WITH_KNOTS ( ( 3, 2, 2, 2, 3 ),
 ( 0.6624999999999992006, 0.6687499999999994005, 0.6749999999999998224, 0.6812500000000000222, 0.6875000000000002220 ),
 .UNSPECIFIED. ) 
 CURVE ( )  GEOMETRIC_REPRESENTATION_ITEM ( )  RATIONAL_B_SPLINE_CURVE ( ( 1.000000000000009548, 0.9238795325112773016, 1.000000000000000000, 0.9238795325112867385, 1.000000000000000000, 0.9238795325112867385, 1.000000000000000000, 0.9238795325112840739, 1.000000000000002665 ) ) 
 REPRESENTATION_ITEM ( '' )  );
#29893=CARTESIAN_POINT ( 'NONE',  ( 140.5000000000000284, -9.599999999999997868, 7.200000000000011724 ) ) ;
#29896=SURFACE_STYLE_USAGE ( .BOTH. , #3786 ) ;
#29900=DIRECTION ( 'NONE',  ( 1.000000000000000000, 0.000000000000000000, -0.000000000000000000 ) ) ;
#29902=CARTESIAN_POINT ( 'NONE',  ( 159.2961002691896226, 2.071067811865468400, -4.999999999999989342 ) ) ;
#29903=CARTESIAN_POINT ( 'NONE',  ( 0.1512544026176828038, -15.31703501317270977, 8.468610511427742793 ) ) ;
#29904=ORIENTED_EDGE ( 'NONE', *, *, #9118, .F. ) ;
#29909=DIRECTION ( 'NONE',  ( 1.000000000000000000, 0.000000000000000000, 0.000000000000000000 ) ) ;
#29915=ORIENTED_EDGE ( 'NONE', *, *, #11615, .T. ) ;
#29917=AXIS2_PLACEMENT_3D ( 'NONE', #2988, #4437, #28624 ) ;
#29918=ORIENTED_EDGE ( 'NONE', *, *, #14719, .T. ) ;
#29919=CARTESIAN_POINT ( 'NONE',  ( 155.2500000000000284, -6.000000000000005329, 0.000000000000000000 ) ) ;
#29932=DIRECTION ( 'NONE',  ( -1.000000000000000000, 0.000000000000000000, 0.000000000000000000 ) ) ;
#29933=CARTESIAN_POINT ( 'NONE',  ( 0.8631338372297875372, -15.37878787878788067, -8.351220472436777342 ) ) ;
#29939=CARTESIAN_POINT ( 'NONE',  ( -6.110151747013052647E-09, -9.999999993889911565, -4.800749288174391616 ) ) ;
#29941=CARTESIAN_POINT ( 'NONE',  ( 162.0000000000000284, 7.960204194457768853E-16, 6.499999999999977796 ) ) ;
#29949=CARTESIAN_POINT ( 'NONE',  ( 142.5148502691896510, -3.535533905932725318, -3.535533905932725318 ) ) ;
#29960=CARTESIAN_POINT ( 'NONE',  ( 141.6562500000000284, -6.000000000000005329, 2.485281374238555774 ) ) ;
#29962=COLOUR_RGB ( '', 0.08235294, 0.09019608, 0.10196078) ;
#29963=VERTEX_POINT ( 'NONE', #29197 ) ;
#29965=( NAMED_UNIT ( * ) PLANE_ANGLE_UNIT ( ) SI_UNIT ( $, .RADIAN. ) );
#29966=STYLED_ITEM ( 'NONE', ( #19512 ), #12132 ) ;
#29967=DIRECTION ( 'NONE',  ( 0.000000000000000000, 0.000000000000000000, 1.000000000000000000 ) ) ;
#29969=( LENGTH_UNIT ( ) NAMED_UNIT ( * ) SI_UNIT ( .MILLI., .METRE. ) );
#29971=CARTESIAN_POINT ( 'NONE',  ( 142.2038997308104058, 2.071067811865468400, 4.999999999999989342 ) ) ;
#29984=SURFACE_STYLE_USAGE ( .BOTH. , #9412 ) ;
#29990=DIRECTION ( 'NONE',  ( -0.000000000000000000, 1.000000000000000000, 0.000000000000000000 ) ) ;
#29991=ORIENTED_EDGE ( 'NONE', *, *, #22118, .T. ) ;
#29993=CARTESIAN_POINT ( 'NONE',  ( 138.4687500000000284, -2.485281374238585972, 6.000000000000005329 ) ) ;
#29995=CARTESIAN_POINT ( 'NONE',  ( 136.2187500000000284, 2.485281374238555774, -6.000000000000005329 ) ) ;
#29996=CARTESIAN_POINT ( 'NONE',  ( -9.999999999999793943, 9.000000000000007105, -3.000000000000002665 ) ) ;
#29998=ORIENTED_EDGE ( 'NONE', *, *, #332, .T. ) ;
#29999=COLOUR_RGB ( '', 0.08235294, 0.09019608, 0.10196078) ;
#30009=CARTESIAN_POINT ( 'NONE',  ( 129.9999999999998010, -89.00000000000001421, 3.000000000000002665 ) ) ;
#30014=EDGE_CURVE ( 'NONE', #27080, #22830, #12981, .T. ) ;
#30016=CARTESIAN_POINT ( 'NONE',  ( 140.5000000000000284, -9.600000000000010303, -7.200000000000006395 ) ) ;
#30018=CARTESIAN_POINT ( 'NONE',  ( 155.2425748654052313, -2.278174593052205932, -5.499999999999819700 ) ) ;
#30025=CARTESIAN_POINT ( 'NONE',  ( 147.7648502691896510, 3.535533905932725318, 3.535533905932752852 ) ) ;
#30033=ORIENTED_EDGE ( 'NONE', *, *, #13655, .T. ) ;
#30034=CARTESIAN_POINT ( 'NONE',  ( 153.1875000000000284, 4.242640687119269671, 4.242640687119298093 ) ) ;
#30035=DIRECTION ( 'NONE',  ( -1.000000000000000000, -1.067522139062651904E-16, 0.000000000000000000 ) ) ;
#30038=ORIENTED_EDGE ( 'NONE', *, *, #4604, .F. ) ;
#30047=CARTESIAN_POINT ( 'NONE',  ( 159.6488248654052029, -3.889087296526011706, -3.889087296526011706 ) ) ;
#30052=FACE_OUTER_BOUND ( 'NONE', #17603, .T. ) ;
#30059=CARTESIAN_POINT ( 'NONE',  ( 161.3586002691896795, 2.071067811865468400, 4.999999999999989342 ) ) ;
#30061=ORIENTED_EDGE ( 'NONE', *, *, #14946, .F. ) ;
#30066=CARTESIAN_POINT ( 'NONE',  ( 161.1037658773653050, -2.857005778783127844E-13, 5.603765877365280090 ) ) ;
#30068=CARTESIAN_POINT ( 'NONE',  ( 116.0000000000000142, 0.000000000000000000, 0.000000000000000000 ) ) ;
#30071=ORIENTED_EDGE ( 'NONE', *, *, #28235, .F. ) ;
#30073=VECTOR ( 'NONE', #24566, 1000.000000000000000 ) ;
#30075=CARTESIAN_POINT ( 'NONE',  ( 150.1875000000000284, 4.242640687119269671, 4.242640687119298093 ) ) ;
#30082=CARTESIAN_POINT ( 'NONE',  ( 158.8050748654052313, 5.500000000000012434, 2.278174593052012309 ) ) ;
#30085=CARTESIAN_POINT ( 'NONE',  ( 159.0000000000000284, -11.07692307692308908, 4.615384615384620304 ) ) ;
#30092=CYLINDRICAL_SURFACE ( 'NONE', #21676, 0.5000000000000000000 ) ;
#30093=DIRECTION ( 'NONE',  ( 0.000000000000000000, 0.000000000000000000, 1.000000000000000000 ) ) ;
#30098=CARTESIAN_POINT ( 'NONE',  ( -9.757819552369539906E-16, -9.499999999869134015, -4.869076758059751597 ) ) ;
#30103=CIRCLE ( 'NONE', #20295, 5.500000000000000000 ) ;
#30104=VERTEX_POINT ( 'NONE', #16355 ) ;
#30106=FACE_OUTER_BOUND ( 'NONE', #27154, .T. ) ;
#30114=( BOUNDED_SURFACE ( )  B_SPLINE_SURFACE ( 1, 2, ( 
 ( #13195, #8061, #10552, #19909, #10875, #26501, #3447, #22068, #5455, #8216, #14862, #12882, #17632, #24205, #10724, #22219, #3152, #12579, #8382, #19611, #1000, #17792, #5911, #28953, #6077, #7917, #17330, #26646, #5605, #10403, #19757, #8855, #18394, #20369, #16264, #11023, #13803, #2092, #25110, #27871, #23304, #6840, #23149, #15804, #9005, #29579, #6533, #27408, #11175, #1623, #27257, #27712, #6692, #29720, #25583, #4070, #6229, #11497, #4376, #22684, #20838, #4537, #8698, #18092, #15648, #16112, #13492, #22831, #6373, #13339, #30187, #1772, #13962, #9153, #2248, #11650, #18546, #8536, #17942, #20524, #24958, #29876, #18238, #25415, #1931, #27555, #3911, #15956, #25254, #4226, #13644, #22989, #11337, #20682, #30034, #26029, #2973, #25879, #2828, #19137, #7584, #9762, #24029, #4834, #26174, #14261, #28324, #23884, #9307, #9464, #4976, #19002, #21440, #7303, #28614, #14684, #16561, #21590, #14544, #20997, #16707, #12251, #30343, #21142, #79, #23746, #23452, #9914, #16850, #4682, #5120, #18698, #521, #19290, #227, #2675, #16996, #14411, #18849, #12100, #23598, #28020, #25735, #14115, #11961, #372, #6993, #26319, #28472, #5276, #16413, #2391, #7439, #11803, #28173, #7143, #2535, #21287, #9613, #13000, #27074, #24620, #10068, #15134, #7884, #28918, #19581, #5876, #24463, #7735, #965, #17295, #5722, #10366, #6039, #22185, #15457, #19871, #26466, #17441, #8180, #29070, #17596, #3570, #15295, #1120, #26755, #26616, #28766, #5424, #21887, #29217, #19724, #8035, #26912, #3415, #22337, #1272, #24783, #10518, #8343, #12395, #20029, #21740, #10685, #17143, #17749, #24177, #24315, #14833, #680, #12841, #19443, #3122, #12543, #824, #10221, #5570, #14974, #3267, #12695, #22028, #13307, #1891, #6660, #3728, #22953, #20484, #18061, #13161, #10841, #27678, #4191, #6337, #27375, #16076, #23111, #29686, #1589, #22648, #15770, #29843, #16226, #25380, #4340, #8821, #8660, #8970, #20806, #13763, #18511, #29544, #22497, #18205, #2059, #27522, #11461, #6500, #18360, #25076, #6197, #30152, #4033, #15924, #25224, #6802, #9115, #13607, #13453, #1429, #11297, #20194, #27833, #20649, #8500, #29995, #17907, #22799, #27225, #15615, #24927, #3876, #10991, #14079, #9577, #23560, #25994, #11922, #2791, #19255, #21107, #26140, #19109, #7550, #21252, #16819, #25541, #25695, #4648, #28286, #27981, #14511, #21406, #9268, #337, #23266, #5085, #23851, #4796, #7267, #21557, #192, #23415, #18970, #28139, #2208, #18662, #6954, #4501, #13923, #12063 ),
 ( #28583, #12218, #14223, #14372, #16373, #485, #2360, #9733, #28433, #38, #9879, #11612, #20954, #7412, #11764, #4942, #9424, #2498, #18812, #7107, #16527, #25848, #23709, #2644, #16672, #8015, #7156, #18711, #14956, #26596, #14127, #12670, #17423, #2405, #11816, #28036, #7453, #16570, #14271, #23467, #4693, #22007, #9477, #26736, #945, #5703, #15112, #3242, #5551, #10344, #23613, #19705, #25894, #93, #19153, #23756, #28183, #21008, #29050, #4844, #24444, #11972, #3395, #383, #9776, #30354, #26045, #9319, #2546, #7005, #16424, #25746, #239, #2690, #21154, #7313, #18862, #16719, #21300, #9622, #19012, #28336, #4988, #14419, #17274, #12114, #21452, #28490, #24295, #8479, #17889, #22164, #6318, #1410, #15745, #15905, #1718, #22472, #1565, #3549, #29821, #24599, #27356, #25056, #8318, #11115, #6481, #20463, #4013, #29356, #22629, #12822, #20171, #10656, #24763, #15271, #10497, #10971, #20319, #12980, #8798, #17728, #19848, #13430, #18040, #5853, #22776, #18184, #22315, #1247, #29196, #29668, #27052, #6019, #20004, #26890, #27503, #15436, #25202, #1101, #8157, #17573, #3703, #13134, #10820, #29518, #27204, #6179, #15592, #8636, #24906, #3855, #13288, #16502, #9092, #25829, #25514, #7245, #14054, #23393, #11899, #9241, #16653, #18489, #4779, #2340, #21233, #11740, #4165, #27807, #9402, #6782, #11590, #7087, #22930, #23089, #18636, #2184, #4623, #20932, #176, #28265, #30130, #14202, #28116, #13589, #30283, #23540, #1870, #4325, #13743, #6932, #6632, #2479, #17, #18342, #18792, #9557, #27957, #16354, #11273, #18947, #2031, #25675, #20627, #29971, #11437, #21083, #8950, #27656, #16054, #25355, #16203, #20783, #4477, #13902, #23243, #28561, #9860, #28864, #14922, #12197, #23834, #14497, #7529, #21688, #7977, #17239, #7823, #12337, #464, #777, #12630, #26565, #10307, #21385, #25976, #624, #5515, #10008, #24259, #2919, #10158, #16940, #28414, #3207, #26269, #28708, #7681, #29012, #909, #19383, #21538, #4918, #17089, #14349, #5219, #26416, #23689, #21830, #5367, #21977, #19532, #19672, #3069, #14776, #26122, #19091, #2626, #12045, #319, #9708, #7394, #16802, #5069, #24120, #19233, #14633, #2770, #23978, #12493, #17384, #15072, #5664, #24415, #3357, #26701, #21341, #3025, #23941, #136, #21497, #12298, #2725, #21641, #7633, #19342, #5175, #423, #23651, #2447, #9520, #25933, #2878, #5024, #12152, #577, #23789, #9964, #5322, #10116, #26220, #12443, #19487, #24076, #28818, #14733, #11856, #28661, #28226, #28372 ) ),
 .UNSPECIFIED., .F., .F., .T. ) 
 B_SPLINE_SURFACE_WITH_KNOTS ( ( 2, 2 ),
 ( 3, 2, 2, 2, 2, 2, 2, 2, 2, 2, 2, 2, 2, 2, 2, 2, 2, 2, 2, 2, 2, 2, 2, 2, 2, 2, 2, 2, 2, 2, 2, 2, 2, 2, 2, 2, 2, 2, 2, 2, 2, 2, 2, 2, 2, 2, 2, 2, 2, 2, 2, 2, 2, 2, 2, 2, 2, 2, 2, 2, 2, 2, 2, 2, 2, 2, 2, 2, 2, 2, 2, 2, 2, 2, 2, 2, 2, 2, 2, 2, 2, 2, 2, 2, 2, 2, 2, 2, 2, 2, 2, 2, 2, 2, 2, 2, 2, 2, 2, 2, 2, 2, 2, 2, 2, 2, 2, 2, 2, 2, 2, 2, 2, 2, 2, 2, 2, 2, 2, 2, 2, 2, 2, 2, 2, 2, 2, 2, 2, 2, 2, 2, 2, 2, 2, 2, 2, 2, 2, 2, 2, 2, 2, 2, 2, 2, 2, 2, 2, 2, 2, 2, 2, 2, 2, 2, 2, 2, 2, 2, 3 ),
 ( 0.000000000000000000, 1.000000000000000000 ),
 ( 0.000000000000000000, 0.006250000000000000347, 0.01250000000000000069, 0.01874999999999999931, 0.02500000000000000139, 0.03125000000000000000, 0.03749999999999999861, 0.04374999999999999722, 0.05000000000000000278, 0.05625000000000000139, 0.06250000000000000000, 0.06875000000000000555, 0.07499999999999999722, 0.08125000000000000278, 0.08749999999999999445, 0.09375000000000000000, 0.1000000000000000056, 0.1062499999999999972, 0.1125000000000000028, 0.1187499999999999944, 0.1250000000000000000, 0.1312500000000000056, 0.1375000000000000111, 0.1437499999999999889, 0.1499999999999999944, 0.1562500000000000000, 0.1625000000000000056, 0.1687500000000000111, 0.1749999999999999889, 0.1812499999999999944, 0.1875000000000000000, 0.1937500000000000056, 0.2000000000000000111, 0.2062499999999999889, 0.2124999999999999944, 0.2187500000000000000, 0.2250000000000000056, 0.2312500000000000111, 0.2374999999999999889, 0.2437499999999999944, 0.2500000000000000000, 0.2562499999999999778, 0.2625000000000000111, 0.2687499999999999889, 0.2750000000000000222, 0.2812500000000000000, 0.2874999999999999778, 0.2937500000000000111, 0.2999999999999999889, 0.3062500000000000222, 0.3125000000000000000, 0.3187499999999999778, 0.3250000000000000111, 0.3312499999999999889, 0.3375000000000000222, 0.3437500000000000000, 0.3499999999999999778, 0.3562500000000000111, 0.3624999999999999889, 0.3687500000000000222, 0.3750000000000000000, 0.3812499999999999778, 0.3875000000000000111, 0.3937499999999999889, 0.4000000000000000222, 0.4062500000000000000, 0.4124999999999999778, 0.4187500000000000111, 0.4249999999999999889, 0.4312500000000000222, 0.4375000000000000000, 0.4437499999999999778, 0.4500000000000000111, 0.4562499999999999889, 0.4625000000000000222, 0.4687500000000000000, 0.4749999999999999778, 0.4812500000000000111, 0.4874999999999999889, 0.4937500000000000222, 0.5000000000000000000, 0.5062499999999999778, 0.5124999999999999556, 0.5187500000000000444, 0.5250000000000000222, 0.5312500000000000000, 0.5374999999999999778, 0.5437499999999999556, 0.5500000000000000444, 0.5562500000000000222, 0.5625000000000000000, 0.5687499999999999778, 0.5749999999999999556, 0.5812500000000000444, 0.5875000000000000222, 0.5937500000000000000, 0.5999999999999999778, 0.6062499999999999556, 0.6125000000000000444, 0.6187500000000000222, 0.6250000000000000000, 0.6312499999999999778, 0.6374999999999999556, 0.6437500000000000444, 0.6500000000000000222, 0.6562500000000000000, 0.6624999999999999778, 0.6687499999999999556, 0.6750000000000000444, 0.6812500000000000222, 0.6875000000000000000, 0.6937499999999999778, 0.6999999999999999556, 0.7062500000000000444, 0.7125000000000000222, 0.7187500000000000000, 0.7249999999999999778, 0.7312499999999999556, 0.7375000000000000444, 0.7437500000000000222, 0.7500000000000000000, 0.7562499999999999778, 0.7624999999999999556, 0.7687500000000000444, 0.7750000000000000222, 0.7812500000000000000, 0.7874999999999999778, 0.7937499999999999556, 0.8000000000000000444, 0.8062500000000000222, 0.8125000000000000000, 0.8187499999999999778, 0.8249999999999999556, 0.8312500000000000444, 0.8375000000000000222, 0.8437500000000000000, 0.8499999999999999778, 0.8562499999999999556, 0.8625000000000000444, 0.8687500000000000222, 0.8750000000000000000, 0.8812499999999999778, 0.8874999999999999556, 0.8937500000000000444, 0.9000000000000000222, 0.9062500000000000000, 0.9124999999999999778, 0.9187499999999999556, 0.9250000000000000444, 0.9312500000000000222, 0.9375000000000000000, 0.9437499999999999778, 0.9499999999999999556, 0.9562500000000000444, 0.9625000000000000222, 0.9687500000000000000, 0.9749999999999999778, 0.9812499999999999556, 0.9875000000000000444, 0.9937500000000000222, 1.000000000000000000 ),
 .UNSPECIFIED. ) 
 GEOMETRIC_REPRESENTATION_ITEM ( )  RATIONAL_B_SPLINE_SURFACE ( (
 ( 1.000000000000000000, 0.9238795325112867385, 1.000000000000000000, 0.9238795325112867385, 1.000000000000000000, 0.9238795325112867385, 1.000000000000000000, 0.9238795325112867385, 1.000000000000000000, 0.9238795325112867385, 1.000000000000000000, 0.9238795325112867385, 1.000000000000000000, 0.9238795325112867385, 1.000000000000000000, 0.9238795325112867385, 1.000000000000000000, 0.9238795325112867385, 1.000000000000000000, 0.9238795325112867385, 1.000000000000000000, 0.9238795325112867385, 1.000000000000000000, 0.9238795325112867385, 1.000000000000000000, 0.9238795325112867385, 1.000000000000000000, 0.9238795325112867385, 1.000000000000000000, 0.9238795325112867385, 1.000000000000000000, 0.9238795325112867385, 1.000000000000000000, 0.9238795325112867385, 1.000000000000000000, 0.9238795325112867385, 1.000000000000000000, 0.9238795325112867385, 1.000000000000000000, 0.9238795325112867385, 1.000000000000000000, 0.9238795325112867385, 1.000000000000000000, 0.9238795325112867385, 1.000000000000000000, 0.9238795325112867385, 1.000000000000000000, 0.9238795325112867385, 1.000000000000000000, 0.9238795325112867385, 1.000000000000000000, 0.9238795325112867385, 1.000000000000000000, 0.9238795325112867385, 1.000000000000000000, 0.9238795325112867385, 1.000000000000000000, 0.9238795325112867385, 1.000000000000000000, 0.9238795325112867385, 1.000000000000000000, 0.9238795325112867385, 1.000000000000000000, 0.9238795325112867385, 1.000000000000000000, 0.9238795325112867385, 1.000000000000000000, 0.9238795325112867385, 1.000000000000000000, 0.9238795325112867385, 1.000000000000000000, 0.9238795325112867385, 1.000000000000000000, 0.9238795325112867385, 1.000000000000000000, 0.9238795325112867385, 1.000000000000000000, 0.9238795325112867385, 1.000000000000000000, 0.9238795325112867385, 1.000000000000000000, 0.9238795325112867385, 1.000000000000000000, 0.9238795325112867385, 1.000000000000000000, 0.9238795325112867385, 1.000000000000000000, 0.9238795325112867385, 1.000000000000000000, 0.9238795325112867385, 1.000000000000000000, 0.9238795325112867385, 1.000000000000000000, 0.9238795325112867385, 1.000000000000000000, 0.9238795325112867385, 1.000000000000000000, 0.9238795325112867385, 1.000000000000000000, 0.9238795325112867385, 1.000000000000000000, 0.9238795325112867385, 1.000000000000000000, 0.9238795325112867385, 1.000000000000000000, 0.9238795325112867385, 1.000000000000000000, 0.9238795325112867385, 1.000000000000000000, 0.9238795325112867385, 1.000000000000000000, 0.9238795325112867385, 1.000000000000000000, 0.9238795325112867385, 1.000000000000000000, 0.9238795325112867385, 1.000000000000000000, 0.9238795325112867385, 1.000000000000000000, 0.9238795325112867385, 1.000000000000000000, 0.9238795325112867385, 1.000000000000000000, 0.9238795325112867385, 1.000000000000000000, 0.9238795325112867385, 1.000000000000000000, 0.9238795325112867385, 1.000000000000000000, 0.9238795325112867385, 1.000000000000000000, 0.9238795325112867385, 1.000000000000000000, 0.9238795325112867385, 1.000000000000000000, 0.9238795325112867385, 1.000000000000000000, 0.9238795325112867385, 1.000000000000000000, 0.9238795325112867385, 1.000000000000000000, 0.9238795325112867385, 1.000000000000000000, 0.9238795325112867385, 1.000000000000000000, 0.9238795325112867385, 1.000000000000000000, 0.9238795325112867385, 1.000000000000000000, 0.9238795325112867385, 1.000000000000000000, 0.9238795325112867385, 1.000000000000000000, 0.9238795325112867385, 1.000000000000000000, 0.9238795325112867385, 1.000000000000000000, 0.9238795325112867385, 1.000000000000000000, 0.9238795325112867385, 1.000000000000000000, 0.9238795325112867385, 1.000000000000000000, 0.9238795325112867385, 1.000000000000000000, 0.9238795325112867385, 1.000000000000000000, 0.9238795325112867385, 1.000000000000000000, 0.9238795325112867385, 1.000000000000000000, 0.9238795325112867385, 1.000000000000000000, 0.9238795325112867385, 1.000000000000000000, 0.9238795325112867385, 1.000000000000000000, 0.9238795325112867385, 1.000000000000000000, 0.9238795325112867385, 1.000000000000000000, 0.9238795325112867385, 1.000000000000000000, 0.9238795325112867385, 1.000000000000000000, 0.9238795325112867385, 1.000000000000000000, 0.9238795325112867385, 1.000000000000000000, 0.9238795325112867385, 1.000000000000000000, 0.9238795325112867385, 1.000000000000000000, 0.9238795325112867385, 1.000000000000000000, 0.9238795325112867385, 1.000000000000000000, 0.9238795325112867385, 1.000000000000000000, 0.9238795325112867385, 1.000000000000000000, 0.9238795325112867385, 1.000000000000000000, 0.9238795325112867385, 1.000000000000000000, 0.9238795325112867385, 1.000000000000000000, 0.9238795325112867385, 1.000000000000000000, 0.9238795325112867385, 1.000000000000000000, 0.9238795325112867385, 1.000000000000000000, 0.9238795325112867385, 1.000000000000000000, 0.9238795325112867385, 1.000000000000000000, 0.9238795325112867385, 1.000000000000000000, 0.9238795325112867385, 1.000000000000000000, 0.9238795325112867385, 1.000000000000000000, 0.9238795325112867385, 1.000000000000000000, 0.9238795325112867385, 1.000000000000000000, 0.9238795325112867385, 1.000000000000000000, 0.9238795325112867385, 1.000000000000000000, 0.9238795325112867385, 1.000000000000000000, 0.9238795325112867385, 1.000000000000000000, 0.9238795325112867385, 1.000000000000000000, 0.9238795325112867385, 1.000000000000000000, 0.9238795325112867385, 1.000000000000000000, 0.9238795325112867385, 1.000000000000000000, 0.9238795325112867385, 1.000000000000000000, 0.9238795325112867385, 1.000000000000000000, 0.9238795325112867385, 1.000000000000000000, 0.9238795325112867385, 1.000000000000000000, 0.9238795325112867385, 1.000000000000000000, 0.9238795325112867385, 1.000000000000000000, 0.9238795325112867385, 1.000000000000000000, 0.9238795325112867385, 1.000000000000000000, 0.9238795325112867385, 1.000000000000000000, 0.9238795325112867385, 1.000000000000000000, 0.9238795325112867385, 1.000000000000000000, 0.9238795325112867385, 1.000000000000000000, 0.9238795325112867385, 1.000000000000000000, 0.9238795325112867385, 1.000000000000000000, 0.9238795325112867385, 1.000000000000000000, 0.9238795325112867385, 1.000000000000000000, 0.9238795325112867385, 1.000000000000000000, 0.9238795325112867385, 1.000000000000000000, 0.9238795325112867385, 1.000000000000000000, 0.9238795325112867385, 1.000000000000000000, 0.9238795325112867385, 1.000000000000000000, 0.9238795325112867385, 1.000000000000000000, 0.9238795325112867385, 1.000000000000000000, 0.9238795325112867385, 1.000000000000000000, 0.9238795325112867385, 1.000000000000000000, 0.9238795325112867385, 1.000000000000000000, 0.9238795325112867385, 1.000000000000000000, 0.9238795325112867385, 1.000000000000000000, 0.9238795325112867385, 1.000000000000000000, 0.9238795325112867385, 1.000000000000000000, 0.9238795325112867385, 1.000000000000000000, 0.9238795325112867385, 1.000000000000000000, 0.9238795325112867385, 1.000000000000000000, 0.9238795325112867385, 1.000000000000000000, 0.9238795325112867385, 1.000000000000000000, 0.9238795325112867385, 1.000000000000000000, 0.9238795325112867385, 1.000000000000000000, 0.9238795325112867385, 1.000000000000000000, 0.9238795325112867385, 1.000000000000000000),
 ( 1.000000000000000000, 0.9238795325112867385, 1.000000000000000000, 0.9238795325112867385, 1.000000000000000000, 0.9238795325112867385, 1.000000000000000000, 0.9238795325112867385, 1.000000000000000000, 0.9238795325112867385, 1.000000000000000000, 0.9238795325112867385, 1.000000000000000000, 0.9238795325112867385, 1.000000000000000000, 0.9238795325112867385, 1.000000000000000000, 0.9238795325112867385, 1.000000000000000000, 0.9238795325112867385, 1.000000000000000000, 0.9238795325112867385, 1.000000000000000000, 0.9238795325112867385, 1.000000000000000000, 0.9238795325112867385, 1.000000000000000000, 0.9238795325112867385, 1.000000000000000000, 0.9238795325112867385, 1.000000000000000000, 0.9238795325112867385, 1.000000000000000000, 0.9238795325112867385, 1.000000000000000000, 0.9238795325112867385, 1.000000000000000000, 0.9238795325112867385, 1.000000000000000000, 0.9238795325112867385, 1.000000000000000000, 0.9238795325112867385, 1.000000000000000000, 0.9238795325112867385, 1.000000000000000000, 0.9238795325112867385, 1.000000000000000000, 0.9238795325112867385, 1.000000000000000000, 0.9238795325112867385, 1.000000000000000000, 0.9238795325112867385, 1.000000000000000000, 0.9238795325112867385, 1.000000000000000000, 0.9238795325112867385, 1.000000000000000000, 0.9238795325112867385, 1.000000000000000000, 0.9238795325112867385, 1.000000000000000000, 0.9238795325112867385, 1.000000000000000000, 0.9238795325112867385, 1.000000000000000000, 0.9238795325112867385, 1.000000000000000000, 0.9238795325112867385, 1.000000000000000000, 0.9238795325112867385, 1.000000000000000000, 0.9238795325112867385, 1.000000000000000000, 0.9238795325112867385, 1.000000000000000000, 0.9238795325112867385, 1.000000000000000000, 0.9238795325112867385, 1.000000000000000000, 0.9238795325112867385, 1.000000000000000000, 0.9238795325112867385, 1.000000000000000000, 0.9238795325112867385, 1.000000000000000000, 0.9238795325112867385, 1.000000000000000000, 0.9238795325112867385, 1.000000000000000000, 0.9238795325112867385, 1.000000000000000000, 0.9238795325112867385, 1.000000000000000000, 0.9238795325112867385, 1.000000000000000000, 0.9238795325112867385, 1.000000000000000000, 0.9238795325112867385, 1.000000000000000000, 0.9238795325112867385, 1.000000000000000000, 0.9238795325112867385, 1.000000000000000000, 0.9238795325112867385, 1.000000000000000000, 0.9238795325112867385, 1.000000000000000000, 0.9238795325112867385, 1.000000000000000000, 0.9238795325112867385, 1.000000000000000000, 0.9238795325112867385, 1.000000000000000000, 0.9238795325112867385, 1.000000000000000000, 0.9238795325112867385, 1.000000000000000000, 0.9238795325112867385, 1.000000000000000000, 0.9238795325112867385, 1.000000000000000000, 0.9238795325112867385, 1.000000000000000000, 0.9238795325112867385, 1.000000000000000000, 0.9238795325112867385, 1.000000000000000000, 0.9238795325112867385, 1.000000000000000000, 0.9238795325112867385, 1.000000000000000000, 0.9238795325112867385, 1.000000000000000000, 0.9238795325112867385, 1.000000000000000000, 0.9238795325112867385, 1.000000000000000000, 0.9238795325112867385, 1.000000000000000000, 0.9238795325112867385, 1.000000000000000000, 0.9238795325112867385, 1.000000000000000000, 0.9238795325112867385, 1.000000000000000000, 0.9238795325112867385, 1.000000000000000000, 0.9238795325112867385, 1.000000000000000000, 0.9238795325112867385, 1.000000000000000000, 0.9238795325112867385, 1.000000000000000000, 0.9238795325112867385, 1.000000000000000000, 0.9238795325112867385, 1.000000000000000000, 0.9238795325112867385, 1.000000000000000000, 0.9238795325112867385, 1.000000000000000000, 0.9238795325112867385, 1.000000000000000000, 0.9238795325112867385, 1.000000000000000000, 0.9238795325112867385, 1.000000000000000000, 0.9238795325112867385, 1.000000000000000000, 0.9238795325112867385, 1.000000000000000000, 0.9238795325112867385, 1.000000000000000000, 0.9238795325112867385, 1.000000000000000000, 0.9238795325112867385, 1.000000000000000000, 0.9238795325112867385, 1.000000000000000000, 0.9238795325112867385, 1.000000000000000000, 0.9238795325112867385, 1.000000000000000000, 0.9238795325112867385, 1.000000000000000000, 0.9238795325112867385, 1.000000000000000000, 0.9238795325112867385, 1.000000000000000000, 0.9238795325112867385, 1.000000000000000000, 0.9238795325112867385, 1.000000000000000000, 0.9238795325112867385, 1.000000000000000000, 0.9238795325112867385, 1.000000000000000000, 0.9238795325112867385, 1.000000000000000000, 0.9238795325112867385, 1.000000000000000000, 0.9238795325112867385, 1.000000000000000000, 0.9238795325112867385, 1.000000000000000000, 0.9238795325112867385, 1.000000000000000000, 0.9238795325112867385, 1.000000000000000000, 0.9238795325112867385, 1.000000000000000000, 0.9238795325112867385, 1.000000000000000000, 0.9238795325112867385, 1.000000000000000000, 0.9238795325112867385, 1.000000000000000000, 0.9238795325112867385, 1.000000000000000000, 0.9238795325112867385, 1.000000000000000000, 0.9238795325112867385, 1.000000000000000000, 0.9238795325112867385, 1.000000000000000000, 0.9238795325112867385, 1.000000000000000000, 0.9238795325112867385, 1.000000000000000000, 0.9238795325112867385, 1.000000000000000000, 0.9238795325112867385, 1.000000000000000000, 0.9238795325112867385, 1.000000000000000000, 0.9238795325112867385, 1.000000000000000000, 0.9238795325112867385, 1.000000000000000000, 0.9238795325112867385, 1.000000000000000000, 0.9238795325112867385, 1.000000000000000000, 0.9238795325112867385, 1.000000000000000000, 0.9238795325112867385, 1.000000000000000000, 0.9238795325112867385, 1.000000000000000000, 0.9238795325112867385, 1.000000000000000000, 0.9238795325112867385, 1.000000000000000000, 0.9238795325112867385, 1.000000000000000000, 0.9238795325112867385, 1.000000000000000000, 0.9238795325112867385, 1.000000000000000000, 0.9238795325112867385, 1.000000000000000000, 0.9238795325112867385, 1.000000000000000000, 0.9238795325112867385, 1.000000000000000000, 0.9238795325112867385, 1.000000000000000000, 0.9238795325112867385, 1.000000000000000000, 0.9238795325112867385, 1.000000000000000000, 0.9238795325112867385, 1.000000000000000000, 0.9238795325112867385, 1.000000000000000000, 0.9238795325112867385, 1.000000000000000000, 0.9238795325112867385, 1.000000000000000000, 0.9238795325112867385, 1.000000000000000000, 0.9238795325112867385, 1.000000000000000000, 0.9238795325112867385, 1.000000000000000000, 0.9238795325112867385, 1.000000000000000000, 0.9238795325112867385, 1.000000000000000000, 0.9238795325112867385, 1.000000000000000000, 0.9238795325112867385, 1.000000000000000000, 0.9238795325112867385, 1.000000000000000000, 0.9238795325112867385, 1.000000000000000000, 0.9238795325112867385, 1.000000000000000000, 0.9238795325112867385, 1.000000000000000000, 0.9238795325112867385, 1.000000000000000000, 0.9238795325112867385, 1.000000000000000000, 0.9238795325112867385, 1.000000000000000000, 0.9238795325112867385, 1.000000000000000000, 0.9238795325112867385, 1.000000000000000000, 0.9238795325112867385, 1.000000000000000000, 0.9238795325112867385, 1.000000000000000000, 0.9238795325112867385, 1.000000000000000000, 0.9238795325112867385, 1.000000000000000000, 0.9238795325112867385, 1.000000000000000000) ) ) 
 REPRESENTATION_ITEM ( '' )  SURFACE ( )  );
#30117=ORIENTED_EDGE ( 'NONE', *, *, #6227, .F. ) ;
#30119=CARTESIAN_POINT ( 'NONE',  ( 135.9375000000000568, -4.242640687119298093, -4.242640687119298093 ) ) ;
#30120=ADVANCED_FACE ( 'NONE', ( #30131 ), #11438, .T. ) ;
#30130=CARTESIAN_POINT ( 'NONE',  ( 144.3601497308104058, -3.535533905932725318, -3.535533905932725318 ) ) ;
#30131=FACE_OUTER_BOUND ( 'NONE', #15172, .T. ) ;
#30137=LINE ( 'NONE', #2347, #23615 ) ;
#30141=DIRECTION ( 'NONE',  ( 1.000000000000000000, -0.000000000000000000, -0.000000000000000000 ) ) ;
#30142=DIRECTION ( 'NONE',  ( 1.000000000000000000, -0.000000000000000000, -0.000000000000000000 ) ) ;
#30145=DIRECTION ( 'NONE',  ( -1.000000000000000000, -0.000000000000000000, -0.000000000000000000 ) ) ;
#30149=CARTESIAN_POINT ( 'NONE',  ( 140.7187500000000284, 2.485281374238556218, -6.000000000000005329 ) ) ;
#30150=CARTESIAN_POINT ( 'NONE',  ( 159.9743574244512843, -12.51706875447920275, -3.259670390775218696 ) ) ;
#30152=CARTESIAN_POINT ( 'NONE',  ( 137.5312500000000284, -2.485281374238555774, -6.000000000000005329 ) ) ;
#30157=VERTEX_POINT ( 'NONE', #2032 ) ;
#30165=( LENGTH_UNIT ( ) NAMED_UNIT ( * ) SI_UNIT ( .MILLI., .METRE. ) );
#30166=CARTESIAN_POINT ( 'NONE',  ( 140.0769230769231228, -11.53846153846154898, -4.615384615384614087 ) ) ;
#30169=CARTESIAN_POINT ( 'NONE',  ( 139.7785334105569461, -9.309084377508947128, -7.921262206628336244 ) ) ;
#30170=TOROIDAL_SURFACE ( 'NONE', #16962, 14.49999999999999289, 0.5000000000000000000 ) ;
#30177=CARTESIAN_POINT ( 'NONE',  ( 139.9672529042787517, -9.668691406906541275, 7.713138574913902978 ) ) ;
#30178=CARTESIAN_POINT ( 'NONE',  ( -39.00000000000000000, -20.00000000000021316, 3.000000000000002665 ) ) ;
#30179=CARTESIAN_POINT ( 'NONE',  ( 156.7500000000000284, -6.000000000000005329, 0.000000000000000000 ) ) ;
#30180=CARTESIAN_POINT ( 'NONE',  ( 144.0863248654052313, 0.000000000000000000, 5.500000000000005329 ) ) ;
#30181=VECTOR ( 'NONE', #23295, 1000.000000000000000 ) ;
#30182=CARTESIAN_POINT ( 'NONE',  ( 140.6185434356032715, -11.23708687120643646, -4.230991509104588211 ) ) ;
#30185=FACE_OUTER_BOUND ( 'NONE', #21371, .T. ) ;
#30186=ORIENTED_EDGE ( 'NONE', *, *, #18645, .T. ) ;
#30187=CARTESIAN_POINT ( 'NONE',  ( 155.4375000000000284, -4.242640687119298093, -4.242640687119298093 ) ) ;
#30191=EDGE_CURVE ( 'NONE', #7007, #3410, #14498, .T. ) ;
#30196=CIRCLE ( 'NONE', #24300, 0.4999999999999980016 ) ;
#30201=CARTESIAN_POINT ( 'NONE',  ( -7.956235894060313657E-16, -9.500000000000008882, -4.414213562373099364 ) ) ;
#30202=CARTESIAN_POINT ( 'NONE',  ( 0.7566289708993888530, -15.57043887889865985, 7.988295740404301348 ) ) ;
#30204=CARTESIAN_POINT ( 'NONE',  ( 159.8363248654052313, 0.000000000000000000, -5.500000000000005329 ) ) ;
#30205=EDGE_LOOP ( 'NONE', ( #23483, #10517, #19841, #26437 ) ) ;
#30207=SURFACE_STYLE_FILL_AREA ( #20853 ) ;
#30213=LINE ( 'NONE', #9176, #7440 ) ;
#30214=CARTESIAN_POINT ( 'NONE',  ( 160.6086002691896795, -2.071067811865468400, -4.999999999999989342 ) ) ;
#30215=CARTESIAN_POINT ( 'NONE',  ( 0.1950273200666144402, -15.66255992321439905, 7.807776097887577649 ) ) ;
#30221=CARTESIAN_POINT ( 'NONE',  ( 157.5074251345948824, 2.278174593052074925, -5.499999999999950262 ) ) ;
#30223=( NAMED_UNIT ( * ) PLANE_ANGLE_UNIT ( ) SI_UNIT ( $, .RADIAN. ) );
#30224=CIRCLE ( 'NONE', #12115, 1.000000000000000888 ) ;
#30230=CARTESIAN_POINT ( 'NONE',  ( 148.8750000000000284, 0.000000000000000000, 6.000000000000005329 ) ) ;
#30235=ORIENTED_EDGE ( 'NONE', *, *, #15752, .T. ) ;
#30236=CYLINDRICAL_SURFACE ( 'NONE', #4852, 5.500000000000000000 ) ;
#30241=CARTESIAN_POINT ( 'NONE',  ( 138.0863248654052313, 0.000000000000000000, 5.500000000000005329 ) ) ;
#30242=CARTESIAN_POINT ( 'NONE',  ( 125.0000000000000568, -55.00000000000000711, 7.500000000000007105 ) ) ;
#30243=CARTESIAN_POINT ( 'NONE',  ( 158.3363248654052313, 0.000000000000000000, -5.500000000000005329 ) ) ;
#30251=CARTESIAN_POINT ( 'NONE',  ( 135.0000000000000284, -7.709521259191705056, -8.196030540009623166 ) ) ;
#30253=ORIENTED_EDGE ( 'NONE', *, *, #13614, .F. ) ;
#30256=EDGE_CURVE ( 'NONE', #4026, #15395, #6097, .T. ) ;
#30257=DIRECTION ( 'NONE',  ( -0.000000000000000000, -0.000000000000000000, -1.000000000000000000 ) ) ;
#30259=MECHANICAL_DESIGN_GEOMETRIC_PRESENTATION_REPRESENTATION('',(#25329),#9658);
#30270=DIRECTION ( 'NONE',  ( -0.000000000000000000, -0.000000000000000000, -1.000000000000000000 ) ) ;
#30271=CARTESIAN_POINT ( 'NONE',  ( 133.8750000000000284, 0.000000000000000000, 6.000000000000005329 ) ) ;
#30277=FILL_AREA_STYLE ('',( #14048 ) ) ;
#30281=LINE ( 'NONE', #14, #10819 ) ;
#30283=CARTESIAN_POINT ( 'NONE',  ( 143.9851497308104058, -3.535533905932725318, 3.535533905932725318 ) ) ;
#30287=CARTESIAN_POINT ( 'NONE',  ( 124.9999999999999432, -71.00000000000001421, -5.000000000000004441 ) ) ;
#30293=ORIENTED_EDGE ( 'NONE', *, *, #16267, .F. ) ;
#30298=EDGE_LOOP ( 'NONE', ( #2350, #29767, #24106 ) ) ;
#30300=COLOUR_RGB ( '', 0.08235294, 0.09019608, 0.10196078) ;
#30301=CARTESIAN_POINT ( 'NONE',  ( 137.4375000000000568, -4.242640687119298093, -4.242640687119298093 ) ) ;
#30302=CARTESIAN_POINT ( 'NONE',  ( 159.9864233307189352, -11.54654450223875095, -3.293895598147179360 ) ) ;
#30318=CARTESIAN_POINT ( 'NONE',  ( 154.6949251345948255, 5.500000000000012434, -2.278174593052012309 ) ) ;
#30330=CARTESIAN_POINT ( 'NONE',  ( 116.0000000000000142, 0.000000000000000000, 0.000000000000000000 ) ) ;
#30332=CARTESIAN_POINT ( 'NONE',  ( 150.4836002691896795, 4.999999999999989342, -2.071067811865468400 ) ) ;
#30334=DIRECTION ( 'NONE',  ( 0.000000000000000000, 0.000000000000000000, 1.000000000000000000 ) ) ;
#30335=CARTESIAN_POINT ( 'NONE',  ( 158.3437500000001137, -6.000000000000005329, -2.485281374238556218 ) ) ;
#30336=( NAMED_UNIT ( * ) PLANE_ANGLE_UNIT ( ) SI_UNIT ( $, .RADIAN. ) );
#30341=ADVANCED_FACE ( 'NONE', ( #8555 ), #15972, .F. ) ;
#30343=CARTESIAN_POINT ( 'NONE',  ( 150.5625000000000568, -4.242640687119298093, 4.242640687119298093 ) ) ;
#30353=SURFACE_SIDE_STYLE ('',( #10039 ) ) ;
#30354=CARTESIAN_POINT ( 'NONE',  ( 155.3288997308104342, 4.999999999999989342, -2.071067811865468400 ) ) ;
#30355=CARTESIAN_POINT ( 'NONE',  ( 159.7425748654052313, -2.278174593052159302, -5.499999999999864997 ) ) ;
#30356=VERTEX_POINT ( 'NONE', #18562 ) ;
#30362=EDGE_CURVE ( 'NONE', #8862, #2367, #2068, .T. ) ;
#30367=CARTESIAN_POINT ( 'NONE',  ( 162.2961002691896510, 2.071067811865468400, -4.999999999999989342 ) ) ;
#30368=CARTESIAN_POINT ( 'NONE',  ( 0.8631338372297875372, -15.37878787878789133, 8.351220472436782671 ) ) ;
#30375=ORIENTED_EDGE ( 'NONE', *, *, #13663, .F. ) ;
#30377=DIRECTION ( 'NONE',  ( 0.000000000000000000, -1.000000000000000000, 0.000000000000000000 ) ) ;
#30382=VERTEX_POINT ( 'NONE', #18410 ) ;
#30383=CARTESIAN_POINT ( 'NONE',  ( 150.2812500000000284, 2.485281374238585972, 6.000000000000005329 ) ) ;
#30388=ORIENTED_EDGE ( 'NONE', *, *, #7409, .T. ) ;
#30389=LINE ( 'NONE', #7047, #13263 ) ;
#30393=VECTOR ( 'NONE', #24639, 1000.000000000000000 ) ;
#30396=DIRECTION ( 'NONE',  ( 0.000000000000000000, 0.000000000000000000, 1.000000000000000000 ) ) ;
#30397=CARTESIAN_POINT ( 'NONE',  ( 158.2425748654052029, -2.278174593052166852, -5.499999999999857003 ) ) ;
#30400=CARTESIAN_POINT ( 'NONE',  ( -0.5000000000000009992, -10.00000000000000888, -5.000000000000004441 ) ) ;
#30401=DIRECTION ( 'NONE',  ( -0.000000000000000000, -0.000000000000000000, -1.000000000000000000 ) ) ;
#30404=CARTESIAN_POINT ( 'NONE',  ( 135.0000000000000284, -7.311326655561703802, -8.296327616267555882 ) ) ;
#30409=CIRCLE ( 'NONE', #13280, 0.5000000000000004441 ) ;
ENDSEC;
END-ISO-10303-21;
